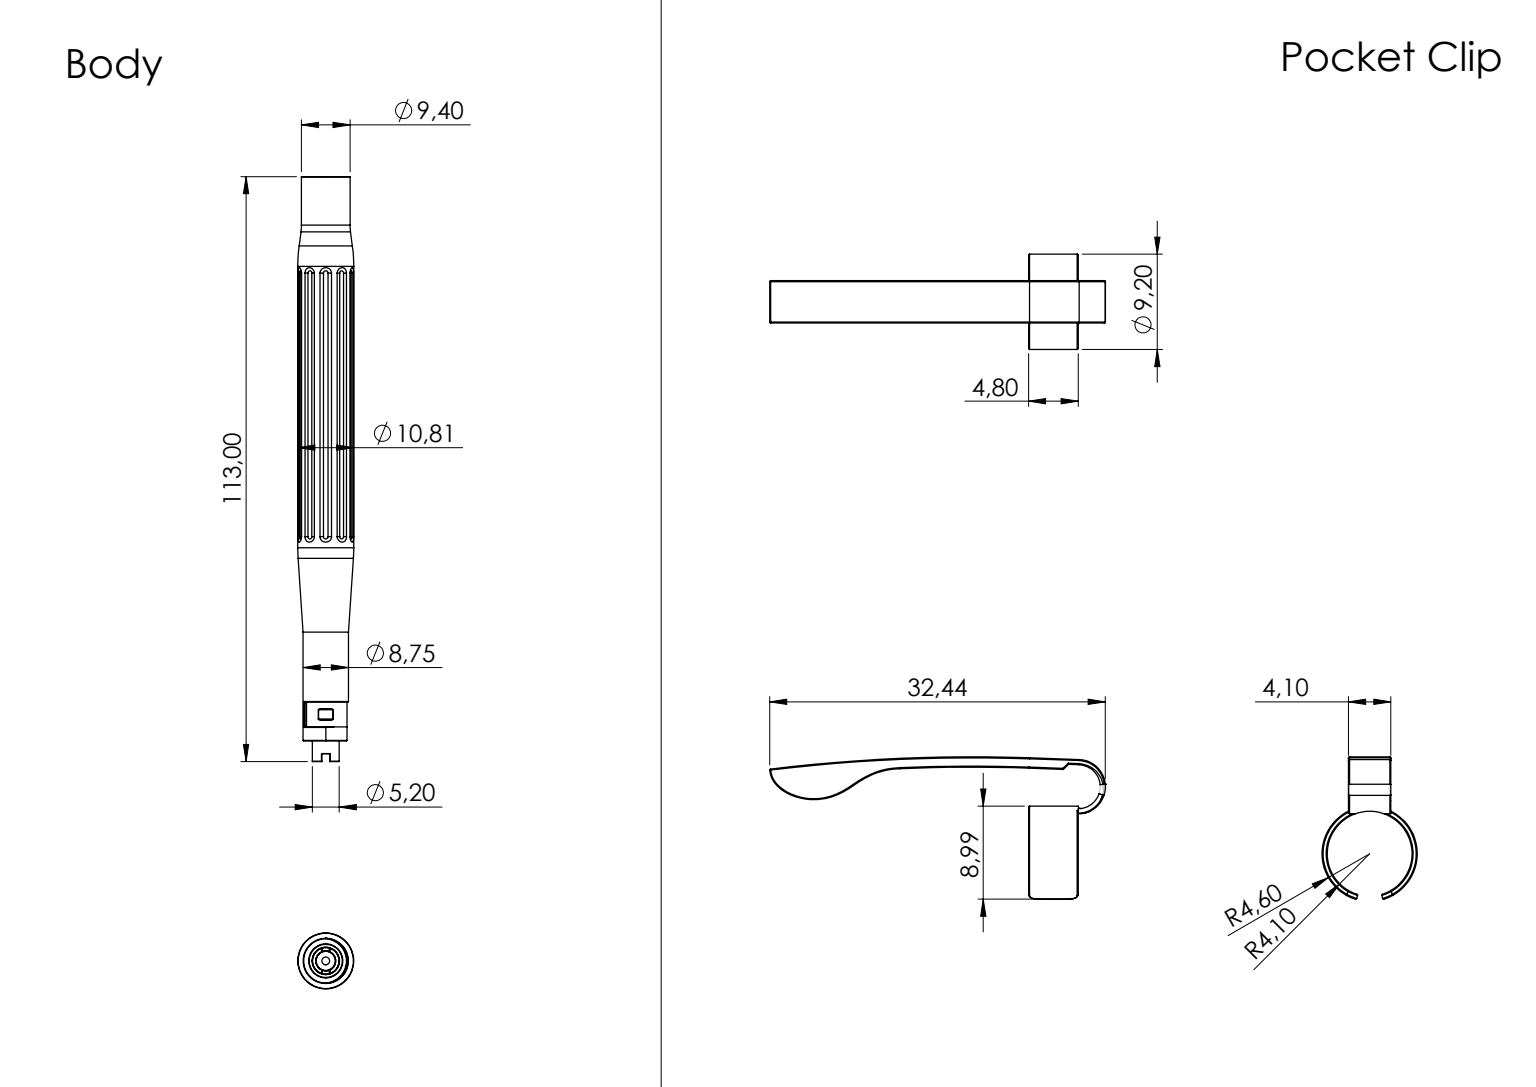
ISO-10303-21;
HEADER;
FILE_DESCRIPTION (('STEP AP214'),
    '1' );
FILE_NAME ('Body.step',
    '2026-10-06T14:00:01',
    ( '' ),
    ( '' ),
    'SwSTEP 2.0',
    'SolidWorks 2020',
    '' );
FILE_SCHEMA (( 'AUTOMOTIVE_DESIGN' ));
ENDSEC;

DATA;
#2=CARTESIAN_POINT ( 'NONE',  ( 51.90000000000001279, -4.227689052994015206, -1.125730994152046804 ) ) ;
#3=CARTESIAN_POINT ( 'NONE',  ( 15.76675455518197388, -3.095036031508637375, 4.435288302043580266 ) ) ;
#4=CARTESIAN_POINT ( 'NONE',  ( 48.30000000000001847, 0.7900853852131533017, -4.025789903357282817 ) ) ;
#5=ADVANCED_FACE ( 'NONE', ( #27029 ), #12933, .F. ) ;
#6=FACE_OUTER_BOUND ( 'NONE', #21820, .T. ) ;
#9=AXIS2_PLACEMENT_3D ( 'NONE', #6479, #25787, #7416 ) ;
#13=EDGE_CURVE ( 'NONE', #19424, #10038, #3404, .T. ) ;
#17=DIRECTION ( 'NONE',  ( 1.000000000000000000, 2.586136946169074517E-16, -0.000000000000000000 ) ) ;
#21=DIRECTION ( 'NONE',  ( 0.000000000000000000, -1.000000000000000000, 0.000000000000000000 ) ) ;
#22=CARTESIAN_POINT ( 'NONE',  ( -35.98994760229849987, 4.804073784580248585, 2.042134692980175803 ) ) ;
#23=LINE ( 'NONE', #15037, #26178 ) ;
#28=ORIENTED_EDGE ( 'NONE', *, *, #15447, .F. ) ;
#29=CARTESIAN_POINT ( 'NONE',  ( 56.95000000000001705, 0.000000000000000000, 0.000000000000000000 ) ) ;
#30=CARTESIAN_POINT ( 'NONE',  ( -35.85663232820584057, -3.426725943139554698, -3.937891353488750301 ) ) ;
#35=ORIENTED_EDGE ( 'NONE', *, *, #5756, .F. ) ;
#39=CIRCLE ( 'NONE', #6115, 0.4576450603546999840 ) ;
#43=CARTESIAN_POINT ( 'NONE',  ( -54.49999999999997868, -1.550000000000000044, 3.332135201338624508 ) ) ;
#47=CARTESIAN_POINT ( 'NONE',  ( -35.85663232820581925, -0.4576450603547171925, -5.200000000000000178 ) ) ;
#49=FACE_OUTER_BOUND ( 'NONE', #3992, .T. ) ;
#50=CARTESIAN_POINT ( 'NONE',  ( 54.42253022455169997, -6.265509898922181047E-05, -4.373069084971676013 ) ) ;
#51=DIRECTION ( 'NONE',  ( 0.000000000000000000, 1.224646799147353454E-16, 1.000000000000000000 ) ) ;
#54=CARTESIAN_POINT ( 'NONE',  ( -36.00197790576391554, -4.683225679163350641, -2.703237727951247393 ) ) ;
#56=CARTESIAN_POINT ( 'NONE',  ( 48.48092587705050960, -1.391939743175890420, 3.849999999996903899 ) ) ;
#61=AXIS2_PLACEMENT_3D ( 'NONE', #970, #25337, #5708 ) ;
#63=ORIENTED_EDGE ( 'NONE', *, *, #635, .F. ) ;
#68=DIRECTION ( 'NONE',  ( 0.000000000000000000, -1.000000000000000000, 0.000000000000000000 ) ) ;
#70=CARTESIAN_POINT ( 'NONE',  ( 48.45334018241207730, -1.329038565861417220, 3.861394075523871816 ) ) ;
#78=CARTESIAN_POINT ( 'NONE',  ( 56.95000000000001705, 0.6999999999999999556, -2.452039967047845437 ) ) ;
#79=CARTESIAN_POINT ( 'NONE',  ( -54.49999516060625382, -1.549196738101655590, 4.063926895246979143 ) ) ;
#82=CARTESIAN_POINT ( 'NONE',  ( 57.03951379057714632, 0.7794871794871794934, 1.732743413496389939 ) ) ;
#83=EDGE_CURVE ( 'NONE', #616, #4702, #25049, .T. ) ;
#88=CARTESIAN_POINT ( 'NONE',  ( 51.80000000000001847, -3.726179070414208372, 1.041421356237310025 ) ) ;
#94=ADVANCED_FACE ( 'NONE', ( #17865 ), #19516, .T. ) ;
#97=CYLINDRICAL_SURFACE ( 'NONE', #25500, 1.000000000000000000 ) ;
#99=CARTESIAN_POINT ( 'NONE',  ( 16.08093158123428523, 5.047763082740414298, 1.943828653492576608 ) ) ;
#101=ORIENTED_EDGE ( 'NONE', *, *, #4763, .T. ) ;
#102=ORIENTED_EDGE ( 'NONE', *, *, #5168, .T. ) ;
#103=DIRECTION ( 'NONE',  ( 0.000000000000000000, 0.000000000000000000, -1.000000000000000000 ) ) ;
#108=CARTESIAN_POINT ( 'NONE',  ( -36.40878371307408656, 5.360483378448119396, 0.7132926830813313135 ) ) ;
#110=FACE_OUTER_BOUND ( 'NONE', #15279, .T. ) ;
#112=DIRECTION ( 'NONE',  ( 0.000000000000000000, 0.000000000000000000, -1.000000000000000000 ) ) ;
#113=DIRECTION ( 'NONE',  ( -1.000000000000000000, -2.586136946169074517E-16, 0.000000000000000000 ) ) ;
#115=CIRCLE ( 'NONE', #28430, 0.1000000000000002554 ) ;
#117=ADVANCED_FACE ( 'NONE', ( #25134 ), #3461, .F. ) ;
#120=CARTESIAN_POINT ( 'NONE',  ( 50.41422517315185559, 1.132063507975340277, -3.941224428058361262 ) ) ;
#121=ADVANCED_FACE ( 'NONE', ( #2812 ), #19777, .T. ) ;
#127=CARTESIAN_POINT ( 'NONE',  ( -36.21152527658242803, -3.291455042465435632, -4.036171416105485577 ) ) ;
#131=EDGE_CURVE ( 'NONE', #11967, #18572, #4827, .T. ) ;
#132=CARTESIAN_POINT ( 'NONE',  ( -54.45981523601835761, 1.500740478982482973, 4.030402907299741599 ) ) ;
#134=FACE_OUTER_BOUND ( 'NONE', #215, .T. ) ;
#135=CARTESIAN_POINT ( 'NONE',  ( 48.39253357792949117, 1.341874354110782486, 3.874311046529112623 ) ) ;
#138=ORIENTED_EDGE ( 'NONE', *, *, #14220, .T. ) ;
#140=CARTESIAN_POINT ( 'NONE',  ( 15.03925126672133139, -3.817150320980667200, 2.203324261490537062 ) ) ;
#141=CARTESIAN_POINT ( 'NONE',  ( 33.47623932017462778, 1.123735532908285650, -5.289358697221546279 ) ) ;
#146=DIRECTION ( 'NONE',  ( 0.000000000000000000, 0.000000000000000000, -1.000000000000000000 ) ) ;
#147=EDGE_CURVE ( 'NONE', #30927, #10142, #27583, .T. ) ;
#148=CARTESIAN_POINT ( 'NONE',  ( -41.12388279035661753, -1.755788972190012401E-14, 0.000000000000000000 ) ) ;
#167=AXIS2_PLACEMENT_3D ( 'NONE', #14057, #2660, #14363 ) ;
#170=FACE_OUTER_BOUND ( 'NONE', #26252, .T. ) ;
#176=CARTESIAN_POINT ( 'NONE',  ( 47.00000000000002132, 2.428612866367529932E-14, -4.100000000000022737 ) ) ;
#178=ADVANCED_FACE ( 'NONE', ( #15936 ), #13241, .T. ) ;
#179=CARTESIAN_POINT ( 'NONE',  ( -35.98952425903315344, -5.086913993735696415, -1.171642046065874743 ) ) ;
#180=ORIENTED_EDGE ( 'NONE', *, *, #3282, .F. ) ;
#183=ORIENTED_EDGE ( 'NONE', *, *, #7527, .F. ) ;
#188=ADVANCED_FACE ( 'NONE', ( #10875 ), #20563, .T. ) ;
#191=CARTESIAN_POINT ( 'NONE',  ( 46.99980596162997415, -4.243812330823901746, 1.064491855880303151 ) ) ;
#192=CARTESIAN_POINT ( 'NONE',  ( 48.40116939571129961, 0.8930800907916158771, -3.925677024646232027 ) ) ;
#194=CARTESIAN_POINT ( 'NONE',  ( 34.55000000000001847, 3.184081677783118191E-16, -2.600000000000000089 ) ) ;
#209=CARTESIAN_POINT ( 'NONE',  ( 15.41170998834797778, 5.326676561279727551, 0.9978806102897876951 ) ) ;
#213=CARTESIAN_POINT ( 'NONE',  ( 48.48434962373865886, -1.386108502191528924, 3.851082811767820413 ) ) ;
#215=EDGE_LOOP ( 'NONE', ( #11588, #9037, #5325, #4414 ) ) ;
#216=CARTESIAN_POINT ( 'NONE',  ( 54.49969840703174384, -0.002993017367635220170, 4.282759600741086636 ) ) ;
#225=CYLINDRICAL_SURFACE ( 'NONE', #7886, 1.000000000000000000 ) ;
#226=PLANE ( 'NONE',  #873 ) ;
#227=CIRCLE ( 'NONE', #16912, 5.147405183146873675 ) ;
#230=VECTOR ( 'NONE', #19201, 1000.000000000000000 ) ;
#234=ORIENTED_EDGE ( 'NONE', *, *, #24307, .F. ) ;
#237=( BOUNDED_SURFACE ( )  B_SPLINE_SURFACE ( 3, 2, ( 
 ( #18207, #22472, #769 ),
 ( #20118, #8066, #17731 ),
 ( #5683, #3307, #12957 ),
 ( #11840, #21216, #1694 ),
 ( #4235, #13877, #16129 ),
 ( #28318, #30847, #18668 ),
 ( #14053, #11689, #9166 ),
 ( #18827, #11541, #18508 ),
 ( #23571, #16434, #23884 ),
 ( #28471, #4086, #21370 ),
 ( #6773, #6625, #1872 ),
 ( #26091, #21047, #30996 ),
 ( #16288, #9487, #23735 ),
 ( #25616, #2026, #30687 ),
 ( #28630, #2175, #8818 ),
 ( #21517, #4405, #13726 ) ),
 .UNSPECIFIED., .F., .F., .F. ) 
 B_SPLINE_SURFACE_WITH_KNOTS ( ( 4, 2, 2, 2, 2, 2, 2, 4 ),
 ( 3, 3 ),
 ( 0.001780502285214259107, 0.002558945925323788048, 0.002753556835351170500, 0.002948167745378552952, 0.003337389565433317423, 0.003726611385488081893, 0.004115833205542846797, 0.004894276845652375738 ),
 ( 0.000000000000000000, 1.000000000000000000 ),
 .UNSPECIFIED. ) 
 GEOMETRIC_REPRESENTATION_ITEM ( )  RATIONAL_B_SPLINE_SURFACE ( (
 ( 1.000000000000000000, 0.9418517008537233837, 1.000000000000000000),
 ( 1.000000000000000000, 0.9417987965885065149, 1.000000000000000000),
 ( 1.000000000000000000, 0.9418198861734086158, 1.000000000000000000),
 ( 1.000000000000000000, 0.9434060303845573925, 1.000000000000000000),
 ( 1.000000000000000000, 0.9437939819948161224, 1.000000000000000000),
 ( 1.000000000000000000, 0.9445989566712799101, 1.000000000000000000),
 ( 1.000000000000000000, 0.9450169930049959754, 1.000000000000000000),
 ( 1.000000000000000000, 0.9461610507673308135, 1.000000000000000000),
 ( 1.000000000000000000, 0.9467217966427053932, 1.000000000000000000),
 ( 1.000000000000000000, 0.9467345476124492398, 1.000000000000000000),
 ( 1.000000000000000000, 0.9461964028052997078, 1.000000000000000000),
 ( 1.000000000000000000, 0.9446801822473757104, 1.000000000000000000),
 ( 1.000000000000000000, 0.9437582546536171790, 1.000000000000000000),
 ( 1.000000000000000000, 0.9418129560296412128, 1.000000000000000000),
 ( 1.000000000000000000, 0.9418016889776917866, 1.000000000000000000),
 ( 1.000000000000000000, 0.9418517008537223845, 1.000000000000000000) ) ) 
 REPRESENTATION_ITEM ( '' )  SURFACE ( )  );
#240=CARTESIAN_POINT ( 'NONE',  ( 16.10667815269232150, 5.098435263432238962, 1.807398698456221142 ) ) ;
#242=ORIENTED_EDGE ( 'NONE', *, *, #16474, .T. ) ;
#246=CARTESIAN_POINT ( 'NONE',  ( -44.49999999999997868, -1.499999999999998668, 4.029888335921975262 ) ) ;
#247=VERTEX_POINT ( 'NONE', #25065 ) ;
#248=EDGE_CURVE ( 'NONE', #1696, #20370, #611, .T. ) ;
#250=ORIENTED_EDGE ( 'NONE', *, *, #30955, .F. ) ;
#252=ADVANCED_FACE ( 'NONE', ( #17489 ), #5461, .T. ) ;
#256=DIRECTION ( 'NONE',  ( -1.000000000000000000, -0.000000000000000000, -0.000000000000000000 ) ) ;
#257=CARTESIAN_POINT ( 'NONE',  ( 16.07512358269907438, -5.233646053067085191, -1.367284724151294872 ) ) ;
#261=EDGE_CURVE ( 'NONE', #13894, #14026, #10669, .T. ) ;
#263=CARTESIAN_POINT ( 'NONE',  ( -36.39645873810205501, -3.590618801409528160, -4.051716037497291367 ) ) ;
#266=CIRCLE ( 'NONE', #22541, 1.000000000000000000 ) ;
#269=CARTESIAN_POINT ( 'NONE',  ( 56.99370871690835116, -0.8156862421929632623, -2.468735699563065378 ) ) ;
#274=CARTESIAN_POINT ( 'NONE',  ( 36.55000000000001847, 0.000000000000000000, -1.899999999999999911 ) ) ;
#278=CARTESIAN_POINT ( 'NONE',  ( 15.22780280894145832, 0.7747498539022198427, -5.363501450340349308 ) ) ;
#279=CARTESIAN_POINT ( 'NONE',  ( -36.56390771145526486, -5.205077242910963520, 1.471673150993815238 ) ) ;
#280=CARTESIAN_POINT ( 'NONE',  ( 48.50000000000002132, -1.426739617975173013, -3.843750000000023093 ) ) ;
#282=ORIENTED_EDGE ( 'NONE', *, *, #8503, .F. ) ;
#290=CARTESIAN_POINT ( 'NONE',  ( 57.04536243881683788, -0.7794871794871796045, 1.732743413496389939 ) ) ;
#291=AXIS2_PLACEMENT_3D ( 'NONE', #19148, #17077, #12003 ) ;
#292=DIRECTION ( 'NONE',  ( -1.000000000000000000, -0.000000000000000000, -0.000000000000000000 ) ) ;
#301=CARTESIAN_POINT ( 'NONE',  ( 51.90000000000001279, 1.734723475976807094E-15, 0.000000000000000000 ) ) ;
#304=EDGE_CURVE ( 'NONE', #17048, #21964, #18751, .T. ) ;
#315=CARTESIAN_POINT ( 'NONE',  ( 57.01990854087920013, 0.7399312420039723115, -2.427820937803477630 ) ) ;
#324=EDGE_CURVE ( 'NONE', #29888, #4483, #21821, .T. ) ;
#325=DIRECTION ( 'NONE',  ( -1.000000000000000000, -2.586136946169074517E-16, 0.000000000000000000 ) ) ;
#328=CARTESIAN_POINT ( 'NONE',  ( 51.70000000000001705, -4.179189514726507682, 0.9999999999999997780 ) ) ;
#332=CARTESIAN_POINT ( 'NONE',  ( -36.92443669619682112, -5.094475812726876995, -1.819860688632578771 ) ) ;
#341=CARTESIAN_POINT ( 'NONE',  ( 50.40811050917463376, 1.340787288841451819, 3.874691554877328414 ) ) ;
#343=CARTESIAN_POINT ( 'NONE',  ( -54.47754877553799702, -1.508273929415538506, 3.305418158118663463 ) ) ;
#349=CARTESIAN_POINT ( 'NONE',  ( -36.43290890416756866, 0.4851603899458080682, -5.391500295856532787 ) ) ;
#350=EDGE_CURVE ( 'NONE', #30188, #2736, #13683, .T. ) ;
#353=CARTESIAN_POINT ( 'NONE',  ( 15.49702763512084047, 4.928592478219022688, -1.658905555082578864 ) ) ;
#354=CARTESIAN_POINT ( 'NONE',  ( 56.95000000000001705, -0.7137254901960784492, 2.500119182087999548 ) ) ;
#364=CARTESIAN_POINT ( 'NONE',  ( 33.47623932017462778, 1.734723475976807489E-15, 0.000000000000000000 ) ) ;
#368=EDGE_LOOP ( 'NONE', ( #14579, #11671, #14342, #26811 ) ) ;
#371=CARTESIAN_POINT ( 'NONE',  ( 15.56401610563845317, 5.370189181194952255, 0.6649548426264916268 ) ) ;
#373=CARTESIAN_POINT ( 'NONE',  ( 48.40000000000001990, -0.6304760106459033064, 3.950000000000022826 ) ) ;
#374=CIRCLE ( 'NONE', #8458, 0.05000000000000012768 ) ;
#376=ORIENTED_EDGE ( 'NONE', *, *, #28015, .T. ) ;
#380=CARTESIAN_POINT ( 'NONE',  ( -35.85663232820584057, 1.793057972834822156, -4.026191436120376999 ) ) ;
#384=CARTESIAN_POINT ( 'NONE',  ( -54.48779575765000516, -1.517266520141195896, 4.041867453639656382 ) ) ;
#386=AXIS2_PLACEMENT_3D ( 'NONE', #15477, #25133, #23717 ) ;
#393=ADVANCED_FACE ( 'NONE', ( #19503 ), #26715, .T. ) ;
#415=ORIENTED_EDGE ( 'NONE', *, *, #7693, .T. ) ;
#420=CARTESIAN_POINT ( 'NONE',  ( 15.41217651307630376, -4.863043649742736285, -1.860644097022675414 ) ) ;
#424=CARTESIAN_POINT ( 'NONE',  ( 50.36059168657180862, 1.279117291415143853, -3.870058441400159754 ) ) ;
#426=CARTESIAN_POINT ( 'NONE',  ( 15.18463186935387377, -4.683225679163126820, -2.703237727951754543 ) ) ;
#432=CARTESIAN_POINT ( 'NONE',  ( -36.68133364217528225, -3.736273719777210456, -3.909490113446789206 ) ) ;
#438=CARTESIAN_POINT ( 'NONE',  ( -36.11692583559979397, -4.683225668089311178, 2.703237747136467473 ) ) ;
#440=CARTESIAN_POINT ( 'NONE',  ( 56.95000000000001705, 0.000000000000000000, 0.000000000000000000 ) ) ;
#441=EDGE_LOOP ( 'NONE', ( #30062, #24496, #16415, #15926 ) ) ;
#444=CARTESIAN_POINT ( 'NONE',  ( 50.50000000000002132, 0.6304760106459513791, 3.950000000000021938 ) ) ;
#446=CARTESIAN_POINT ( 'NONE',  ( -54.44999999999997442, 0.000000000000000000, 4.349999999999997868 ) ) ;
#458=CIRCLE ( 'NONE', #5023, 0.05000000000000012768 ) ;
#467=DIRECTION ( 'NONE',  ( 1.000000000000000000, 3.385297212316258532E-16, -2.459562394685744279E-16 ) ) ;
#469=DIRECTION ( 'NONE',  ( 0.000000000000000000, 0.000000000000000000, 1.000000000000000000 ) ) ;
#473=VERTEX_POINT ( 'NONE', #3169 ) ;
#475=DIRECTION ( 'NONE',  ( -1.000000000000000000, -0.000000000000000000, -0.000000000000000000 ) ) ;
#476=EDGE_CURVE ( 'NONE', #20395, #3490, #29876, .T. ) ;
#478=ORIENTED_EDGE ( 'NONE', *, *, #27718, .F. ) ;
#480=CARTESIAN_POINT ( 'NONE',  ( 50.39883060428874728, 0.8930800907916158771, 3.925677024646232027 ) ) ;
#481=CARTESIAN_POINT ( 'NONE',  ( -36.68133364217572989, -5.320649567603509489, -0.9667173501063568430 ) ) ;
#487=EDGE_CURVE ( 'NONE', #25704, #26503, #27864, .T. ) ;
#494=CARTESIAN_POINT ( 'NONE',  ( 48.37881665787880081, -1.311095223031167656, -3.884869838566831657 ) ) ;
#496=CARTESIAN_POINT ( 'NONE',  ( 51.80019403837007275, -4.243812330823898193, -1.064491855880295157 ) ) ;
#502=EDGE_CURVE ( 'NONE', #31046, #17227, #27711, .T. ) ;
#505=CARTESIAN_POINT ( 'NONE',  ( 15.17256654081408307, 4.804073784580281448, -2.042134692980007937 ) ) ;
#508=LINE ( 'NONE', #19531, #10386 ) ;
#510=CARTESIAN_POINT ( 'NONE',  ( 15.29449157529453984, 2.734387802834222558, -4.440904455451668120 ) ) ;
#513=ORIENTED_EDGE ( 'NONE', *, *, #6499, .F. ) ;
#518=VERTEX_POINT ( 'NONE', #3495 ) ;
#519=ORIENTED_EDGE ( 'NONE', *, *, #15693, .T. ) ;
#520=CARTESIAN_POINT ( 'NONE',  ( 15.03925126672132784, 5.377732432866634937, 0.5657657256216264141 ) ) ;
#524=DIRECTION ( 'NONE',  ( -4.117859380279907901E-15, -0.9495137264943731559, -0.3137254901960768172 ) ) ;
#529=EDGE_CURVE ( 'NONE', #10936, #30188, #15204, .T. ) ;
#533=EDGE_CURVE ( 'NONE', #27746, #12623, #23876, .T. ) ;
#534=CARTESIAN_POINT ( 'NONE',  ( -54.49608498031047787, -1.530604779201329091, 4.051096982736678953 ) ) ;
#539=DIRECTION ( 'NONE',  ( 1.000000000000000000, 0.000000000000000000, 0.000000000000000000 ) ) ;
#540=EDGE_CURVE ( 'NONE', #20985, #4962, #20292, .T. ) ;
#548=ORIENTED_EDGE ( 'NONE', *, *, #30878, .F. ) ;
#558=EDGE_LOOP ( 'NONE', ( #6600, #18904, #20461, #4910 ) ) ;
#560=VERTEX_POINT ( 'NONE', #22668 ) ;
#562=ORIENTED_EDGE ( 'NONE', *, *, #8648, .F. ) ;
#567=CARTESIAN_POINT ( 'NONE',  ( 15.22780280894113325, -4.861582133260076155, -2.394243994562784916 ) ) ;
#568=EDGE_CURVE ( 'NONE', #19552, #25905, #3138, .T. ) ;
#573=CARTESIAN_POINT ( 'NONE',  ( -44.49999999999997868, -1.500000000000000000, 3.300094695611020867 ) ) ;
#581=CARTESIAN_POINT ( 'NONE',  ( -36.30347965937272647, -3.148602930107041065, -4.139959549308994902 ) ) ;
#598=CARTESIAN_POINT ( 'NONE',  ( 56.95000000000001705, -0.6820512820512819596, 1.773360101234998210 ) ) ;
#600=CARTESIAN_POINT ( 'NONE',  ( 58.50000000000001421, 0.000000000000000000, 0.000000000000000000 ) ) ;
#601=AXIS2_PLACEMENT_3D ( 'NONE', #25474, #29769, #15523 ) ;
#603=CIRCLE ( 'NONE', #61, 4.700000000000000178 ) ;
#605=CARTESIAN_POINT ( 'NONE',  ( 48.40000000000001990, 2.428612866367529932E-14, 0.000000000000000000 ) ) ;
#607=ORIENTED_EDGE ( 'NONE', *, *, #22678, .F. ) ;
#608=CARTESIAN_POINT ( 'NONE',  ( 16.07279755198631932, 2.910597594660116805, 4.559461819278099348 ) ) ;
#611=B_SPLINE_CURVE_WITH_KNOTS ( 'NONE', 3,
 ( #22873, #22726, #25234, #10817, #1022, #20026, #10673, #13190, #29668, #29978, #1162, #27768, #14940, #12569, #5615, #22258, #19870, #29499, #7815 ),
 .UNSPECIFIED., .F., .F.,
 ( 4, 3, 3, 3, 3, 3, 4 ),
 ( 0.000000000000000000, 1.485152479261659526E-05, 2.963899638137937738E-05, 4.531421101975830796E-05, 6.339282692920775891E-05, 8.412900350910317146E-05, 8.561427748423838346E-05 ),
 .UNSPECIFIED. ) ;
#612=LINE ( 'NONE', #20579, #31143 ) ;
#613=CARTESIAN_POINT ( 'NONE',  ( -36.38012252111234091, 4.735538777079434603, -2.618062770414225859 ) ) ;
#616=VERTEX_POINT ( 'NONE', #13744 ) ;
#618=VERTEX_POINT ( 'NONE', #31015 ) ;
#622=DIRECTION ( 'NONE',  ( 0.000000000000000000, 0.2745098039215694841, -0.9615843008030765526 ) ) ;
#623=DIRECTION ( 'NONE',  ( -1.000000000000000000, -2.586136946169074517E-16, 0.000000000000000000 ) ) ;
#633=CARTESIAN_POINT ( 'NONE',  ( -36.56390771145526486, -5.076023720898236391, -1.868859051106839475 ) ) ;
#635=EDGE_CURVE ( 'NONE', #25117, #29888, #25505, .T. ) ;
#641=DIRECTION ( 'NONE',  ( 0.000000000000000000, 1.000000000000000000, 0.000000000000000000 ) ) ;
#643=CARTESIAN_POINT ( 'NONE',  ( 15.45522337368519850, -0.1928884786867813006, 5.200000000471195705 ) ) ;
#649=CIRCLE ( 'NONE', #30477, 4.300000000000019362 ) ;
#650=DIRECTION ( 'NONE',  ( 0.000000000000000000, -0.000000000000000000, -1.000000000000000000 ) ) ;
#651=CARTESIAN_POINT ( 'NONE',  ( 15.97944027357901753, -3.614202567155989421, 4.024415706308047014 ) ) ;
#652=CARTESIAN_POINT ( 'NONE',  ( 15.76675455518219238, 5.110933801299809787, -1.769007076671054390 ) ) ;
#655=CARTESIAN_POINT ( 'NONE',  ( 50.42106458229518751, -0.9199776782966014865, -3.998258245321812510 ) ) ;
#656=CARTESIAN_POINT ( 'NONE',  ( -35.85663232820583346, -4.683225679163351529, -2.703237727951242952 ) ) ;
#657=CARTESIAN_POINT ( 'NONE',  ( 15.44631504820162426, 2.881190829692330979, -4.334245811858005837 ) ) ;
#674=ORIENTED_EDGE ( 'NONE', *, *, #25991, .F. ) ;
#678=CIRCLE ( 'NONE', #10773, 1.850000000000000089 ) ;
#681=PLANE ( 'NONE',  #3139 ) ;
#684=FACE_OUTER_BOUND ( 'NONE', #441, .T. ) ;
#686=EDGE_CURVE ( 'NONE', #24297, #29070, #5670, .T. ) ;
#687=CARTESIAN_POINT ( 'NONE',  ( -36.48821680285185209, -3.495540671458102988, 4.131527132740904662 ) ) ;
#688=CARTESIAN_POINT ( 'NONE',  ( 15.03925126672133139, -4.945493884734801782, 1.606888370749709027 ) ) ;
#689=CARTESIAN_POINT ( 'NONE',  ( 50.40000000000001990, 2.428612866367529932E-14, 0.000000000000000000 ) ) ;
#693=AXIS2_PLACEMENT_3D ( 'NONE', #28518, #6823, #16487 ) ;
#694=EDGE_LOOP ( 'NONE', ( #11145, #17669, #9882, #6922 ) ) ;
#697=ORIENTED_EDGE ( 'NONE', *, *, #22187, .T. ) ;
#699=CARTESIAN_POINT ( 'NONE',  ( -54.44999999999997442, 1.499999999999999556, -4.029888335921975262 ) ) ;
#701=CARTESIAN_POINT ( 'NONE',  ( 15.59140265158955074, 4.755985070912251977, 2.573747172434746933 ) ) ;
#708=EDGE_CURVE ( 'NONE', #25469, #23625, #14965, .T. ) ;
#711=EDGE_CURVE ( 'NONE', #13242, #19150, #227, .T. ) ;
#715=CARTESIAN_POINT ( 'NONE',  ( 15.44259799936802047, -4.878092280899799071, -1.814329181850236727 ) ) ;
#722=DIRECTION ( 'NONE',  ( -1.000000000000000000, -0.000000000000000000, -0.000000000000000000 ) ) ;
#726=LINE ( 'NONE', #12044, #17578 ) ;
#727=( BOUNDED_SURFACE ( )  B_SPLINE_SURFACE ( 3, 2, ( 
 ( #12834, #20466, #5581 ),
 ( #10487, #25026, #12537 ),
 ( #20162, #17300, #5726 ),
 ( #27562, #24567, #15231 ),
 ( #22842, #24876, #22516 ),
 ( #10317, #17450, #27263 ),
 ( #26944, #29627, #819 ),
 ( #5891, #1131, #29792 ),
 ( #7953, #13008, #10783 ),
 ( #3357, #17618, #24731 ),
 ( #2886, #5252, #13156 ),
 ( #3192, #8255, #657 ),
 ( #8106, #3044, #22692 ),
 ( #5419, #22223, #510 ),
 ( #12687, #17775, #987 ),
 ( #10167, #27416, #17922 ) ),
 .UNSPECIFIED., .F., .F., .F. ) 
 B_SPLINE_SURFACE_WITH_KNOTS ( ( 4, 2, 2, 2, 2, 2, 2, 4 ),
 ( 3, 3 ),
 ( 0.001780502285214198826, 0.002558945925323778507, 0.002753556835351173536, 0.002948167745378568131, 0.003337389565433357755, 0.003726611385488147379, 0.004115833205542937002, 0.004894276845652516250 ),
 ( 0.000000000000000000, 1.000000000000000000 ),
 .UNSPECIFIED. ) 
 GEOMETRIC_REPRESENTATION_ITEM ( )  RATIONAL_B_SPLINE_SURFACE ( (
 ( 1.000000000000000000, 0.9418517008537241608, 1.000000000000000000),
 ( 1.000000000000000000, 0.9417987965884988544, 1.000000000000000000),
 ( 1.000000000000000000, 0.9418198861734230487, 1.000000000000000000),
 ( 1.000000000000000000, 0.9434060303845539508, 1.000000000000000000),
 ( 1.000000000000000000, 0.9437939819948095721, 1.000000000000000000),
 ( 1.000000000000000000, 0.9445989566712880148, 1.000000000000000000),
 ( 1.000000000000000000, 0.9450169930049983069, 1.000000000000000000),
 ( 1.000000000000000000, 0.9461610507673332560, 1.000000000000000000),
 ( 1.000000000000000000, 0.9467217966427213804, 1.000000000000000000),
 ( 1.000000000000000000, 0.9467345476124363612, 1.000000000000000000),
 ( 1.000000000000000000, 0.9461964028052722853, 1.000000000000000000),
 ( 1.000000000000000000, 0.9446801822474062416, 1.000000000000000000),
 ( 1.000000000000000000, 0.9437582546536901207, 1.000000000000000000),
 ( 1.000000000000000000, 0.9418129560294949965, 1.000000000000000000),
 ( 1.000000000000000000, 0.9418016889778024758, 1.000000000000000000),
 ( 1.000000000000000000, 0.9418517008537236057, 1.000000000000000000) ) ) 
 REPRESENTATION_ITEM ( '' )  SURFACE ( )  );
#731=ADVANCED_FACE ( 'NONE', ( #7124 ), #21860, .F. ) ;
#733=CARTESIAN_POINT ( 'NONE',  ( -36.26369610968621515, -2.881190829692320321, -4.334245811858070674 ) ) ;
#736=DIRECTION ( 'NONE',  ( 0.000000000000000000, -0.9119702176296791141, -0.4102564102564098536 ) ) ;
#739=CARTESIAN_POINT ( 'NONE',  ( 15.30042582489635095, -1.123735543663344938, -5.289358694936611371 ) ) ;
#740=AXIS2_PLACEMENT_3D ( 'NONE', #8039, #24813, #27350 ) ;
#745=DIRECTION ( 'NONE',  ( 0.000000000000000000, 0.000000000000000000, -1.000000000000000000 ) ) ;
#746=DIRECTION ( 'NONE',  ( 0.000000000000000000, 0.000000000000000000, -1.000000000000000000 ) ) ;
#747=ORIENTED_EDGE ( 'NONE', *, *, #9238, .F. ) ;
#749=DIRECTION ( 'NONE',  ( -1.000000000000000000, -2.586136946169074517E-16, 0.000000000000000000 ) ) ;
#750=AXIS2_PLACEMENT_3D ( 'NONE', #11893, #21738, #11742 ) ;
#751=CARTESIAN_POINT ( 'NONE',  ( -44.49999999999997868, 0.000000000000000000, 0.000000000000000000 ) ) ;
#754=CARTESIAN_POINT ( 'NONE',  ( 56.97512559646294505, -0.7466375667864569854, 1.747149777169433094 ) ) ;
#759=CARTESIAN_POINT ( 'NONE',  ( 15.59055531549694074, 0.9785522574022036402, 5.318456145981286909 ) ) ;
#768=CARTESIAN_POINT ( 'NONE',  ( -35.85663232820582635, 4.861582140531628404, -2.394243978978282783 ) ) ;
#769=CARTESIAN_POINT ( 'NONE',  ( -35.85663232820581925, 0.4576450603546987073, 5.200000000000000178 ) ) ;
#770=CARTESIAN_POINT ( 'NONE',  ( 48.44629147628577215, 1.309359793766484925, -3.864871860988134955 ) ) ;
#774=ORIENTED_EDGE ( 'NONE', *, *, #19717, .T. ) ;
#777=CARTESIAN_POINT ( 'NONE',  ( 15.03925126672133139, -4.018128179617529661, -3.618665901676669350 ) ) ;
#778=DIRECTION ( 'NONE',  ( -1.000000000000000000, -0.000000000000000000, -0.000000000000000000 ) ) ;
#787=CARTESIAN_POINT ( 'NONE',  ( 51.79804399563283823, -4.143014423056512463, 1.077153443819862000 ) ) ;
#792=CIRCLE ( 'NONE', #10394, 0.05000000000000012768 ) ;
#809=CARTESIAN_POINT ( 'NONE',  ( 58.50000000000001421, -0.8156862745098042433, 2.468735688885369317 ) ) ;
#812=CARTESIAN_POINT ( 'NONE',  ( -35.85663232820584057, 3.426725943139577790, -3.937891353488711221 ) ) ;
#813=EDGE_CURVE ( 'NONE', #21791, #9481, #23476, .T. ) ;
#816=CARTESIAN_POINT ( 'NONE',  ( 58.45000000000001705, 0.8000000000000002665, 2.421260002560650104 ) ) ;
#818=CARTESIAN_POINT ( 'NONE',  ( 19.23646557533807666, -5.338914163118011480, 0.000000000000000000 ) ) ;
#819=CARTESIAN_POINT ( 'NONE',  ( 15.45522337368517007, 3.212533369474642075, -4.093511368021645502 ) ) ;
#820=CARTESIAN_POINT ( 'NONE',  ( 15.03925126672132961, -0.4576450603546909912, -5.200000000000000178 ) ) ;
#825=TOROIDAL_SURFACE ( 'NONE', #18539, 4.275000000000000355, 0.1000000000000000056 ) ;
#829=ORIENTED_EDGE ( 'NONE', *, *, #540, .T. ) ;
#830=AXIS2_PLACEMENT_3D ( 'NONE', #10089, #14821, #7562 ) ;
#831=CARTESIAN_POINT ( 'NONE',  ( 16.10660252424456118, 5.053896291911992300, -1.944420249220595087 ) ) ;
#832=FACE_OUTER_BOUND ( 'NONE', #30522, .T. ) ;
#838=CIRCLE ( 'NONE', #28645, 0.05000000000000002359 ) ;
#839=DIRECTION ( 'NONE',  ( 0.000000000000000000, 0.000000000000000000, 1.000000000000000000 ) ) ;
#850=CARTESIAN_POINT ( 'NONE',  ( 57.02888841125436414, -0.7778303923484506388, -1.733491207451775207 ) ) ;
#853=CARTESIAN_POINT ( 'NONE',  ( 50.50000000000002132, 2.478823385132571406E-14, 4.100000000000022737 ) ) ;
#855=TOROIDAL_SURFACE ( 'NONE', #7439, 14.70000000000000995, 10.00000000000000000 ) ;
#857=CARTESIAN_POINT ( 'NONE',  ( 50.30000000000001847, -1.426739617975173013, -3.843750000000023093 ) ) ;
#862=AXIS2_PLACEMENT_3D ( 'NONE', #23773, #6339, #16472 ) ;
#867=CARTESIAN_POINT ( 'NONE',  ( -54.49999999999997868, 1.549999999999999600, -4.064480286580312907 ) ) ;
#871=ORIENTED_EDGE ( 'NONE', *, *, #6348, .T. ) ;
#873=AXIS2_PLACEMENT_3D ( 'NONE', #4818, #30956, #16389 ) ;
#877=LINE ( 'NONE', #29989, #14989 ) ;
#879=ORIENTED_EDGE ( 'NONE', *, *, #28610, .F. ) ;
#881=ORIENTED_EDGE ( 'NONE', *, *, #9302, .T. ) ;
#883=ADVANCED_FACE ( 'NONE', ( #20259, #26238, #4545, #26073, #16117, #21027 ), #30830, .T. ) ;
#889=AXIS2_PLACEMENT_3D ( 'NONE', #16006, #20779, #20468 ) ;
#890=CARTESIAN_POINT ( 'NONE',  ( 15.03925126672133139, -5.086913985776139846, -1.171642053949128126 ) ) ;
#895=CIRCLE ( 'NONE', #25653, 0.7500000000000186517 ) ;
#898=FACE_OUTER_BOUND ( 'NONE', #17661, .T. ) ;
#903=CARTESIAN_POINT ( 'NONE',  ( -35.85663232820583346, -4.383220986679503994, -0.4611378927914501769 ) ) ;
#905=CARTESIAN_POINT ( 'NONE',  ( 58.45000000000001705, 0.8000000000000000444, -2.421260002560649660 ) ) ;
#907=ORIENTED_EDGE ( 'NONE', *, *, #18125, .T. ) ;
#910=CIRCLE ( 'NONE', #6467, 30.00000000000000000 ) ;
#918=FACE_OUTER_BOUND ( 'NONE', #25241, .T. ) ;
#926=DIRECTION ( 'NONE',  ( 0.000000000000000000, 0.000000000000000000, 1.000000000000000000 ) ) ;
#927=CARTESIAN_POINT ( 'NONE',  ( 34.55000000000001847, 0.000000000000000000, -2.649999999999999911 ) ) ;
#933=CARTESIAN_POINT ( 'NONE',  ( 51.70000000000001705, -4.179189514726506793, -1.000000000000000000 ) ) ;
#938=( BOUNDED_SURFACE ( )  B_SPLINE_SURFACE ( 3, 2, ( 
 ( #19024, #11734, #2554 ),
 ( #30892, #16809, #26139 ),
 ( #9821, #23778, #2069 ),
 ( #9208, #19488, #24077 ),
 ( #6815, #12054, #9683 ),
 ( #7455, #26771, #5074 ),
 ( #14726, #24387, #18869 ),
 ( #21408, #28682, #26299 ),
 ( #4600, #23927, #17739 ),
 ( #27380, #15509, #24528 ),
 ( #12649, #29433, #19952 ),
 ( #15193, #29585, #12336 ),
 ( #12966, #5373, #3313 ),
 ( #7745, #5690, #17411 ),
 ( #24842, #10282, #22184 ),
 ( #777, #24694, #20281 ) ),
 .UNSPECIFIED., .F., .F., .F. ) 
 B_SPLINE_SURFACE_WITH_KNOTS ( ( 4, 2, 2, 2, 2, 2, 2, 4 ),
 ( 3, 3 ),
 ( 0.001780502285214210318, 0.002558945925323797589, 0.002753556835351194353, 0.002948167745378591116, 0.003337389565433385077, 0.003726611385488179037, 0.004115833205542972564, 0.004894276845652559618 ),
 ( 0.000000000000000000, 1.000000000000000000 ),
 .UNSPECIFIED. ) 
 GEOMETRIC_REPRESENTATION_ITEM ( )  RATIONAL_B_SPLINE_SURFACE ( (
 ( 1.000000000000000000, 0.9418517008537219404, 1.000000000000000000),
 ( 1.000000000000000000, 0.9417987965885504797, 1.000000000000000000),
 ( 1.000000000000000000, 0.9418198861733489968, 1.000000000000000000),
 ( 1.000000000000000000, 0.9434060303845699380, 1.000000000000000000),
 ( 1.000000000000000000, 0.9437939819948041320, 1.000000000000000000),
 ( 1.000000000000000000, 0.9445989566712896801, 1.000000000000000000),
 ( 1.000000000000000000, 0.9450169930049926448, 1.000000000000000000),
 ( 1.000000000000000000, 0.9461610507673384740, 1.000000000000000000),
 ( 1.000000000000000000, 0.9467217966427268205, 1.000000000000000000),
 ( 1.000000000000000000, 0.9467345476124273684, 1.000000000000000000),
 ( 1.000000000000000000, 0.9461964028052701758, 1.000000000000000000),
 ( 1.000000000000000000, 0.9446801822474041321, 1.000000000000000000),
 ( 1.000000000000000000, 0.9437582546536517070, 1.000000000000000000),
 ( 1.000000000000000000, 0.9418129560295660507, 1.000000000000000000),
 ( 1.000000000000000000, 0.9418016889777457434, 1.000000000000000000),
 ( 1.000000000000000000, 0.9418517008537213853, 1.000000000000000000) ) ) 
 REPRESENTATION_ITEM ( '' )  SURFACE ( )  );
#941=CARTESIAN_POINT ( 'NONE',  ( 58.45000000000001705, -0.8000000000000000444, -2.421260002560650104 ) ) ;
#943=EDGE_CURVE ( 'NONE', #26590, #11900, #22875, .T. ) ;
#949=FACE_OUTER_BOUND ( 'NONE', #15304, .T. ) ;
#956=CARTESIAN_POINT ( 'NONE',  ( 58.50000000000001421, 0.8000000000000000444, -2.421260002560650104 ) ) ;
#958=VECTOR ( 'NONE', #6160, 1000.000000000000000 ) ;
#969=EDGE_CURVE ( 'NONE', #29917, #14986, #115, .T. ) ;
#970=CARTESIAN_POINT ( 'NONE',  ( -45.15971931043468146, 0.000000000000000000, 0.000000000000000000 ) ) ;
#974=CARTESIAN_POINT ( 'NONE',  ( 15.03925126672132961, 0.4576450603546987073, 5.200000000000000178 ) ) ;
#976=CARTESIAN_POINT ( 'NONE',  ( 57.05000000000001847, -0.7500000000000000000, -2.421260002560649660 ) ) ;
#983=ORIENTED_EDGE ( 'NONE', *, *, #25197, .F. ) ;
#984=CARTESIAN_POINT ( 'NONE',  ( 50.29999999999740368, -1.409901620923685206, -3.849999999997240518 ) ) ;
#987=CARTESIAN_POINT ( 'NONE',  ( 15.17256654081427492, 2.686240678227970413, -4.475885392925021300 ) ) ;
#992=CARTESIAN_POINT ( 'NONE',  ( 47.10000000000002274, -4.179189514726507682, 0.9999999999999997780 ) ) ;
#994=ORIENTED_EDGE ( 'NONE', *, *, #9268, .T. ) ;
#1000=ORIENTED_EDGE ( 'NONE', *, *, #568, .F. ) ;
#1001=DIRECTION ( 'NONE',  ( 1.000000000000000000, 8.626663965456006092E-17, 1.494526870159786164E-16 ) ) ;
#1007=ORIENTED_EDGE ( 'NONE', *, *, #19113, .F. ) ;
#1008=CIRCLE ( 'NONE', #25269, 0.05000000000000014155 ) ;
#1011=DIRECTION ( 'NONE',  ( -1.000000000000000000, 0.000000000000000000, 0.000000000000000000 ) ) ;
#1012=DIRECTION ( 'NONE',  ( 0.000000000000000000, 0.000000000000000000, 1.000000000000000000 ) ) ;
#1019=DIRECTION ( 'NONE',  ( 1.000000000000000000, 4.939082069373669245E-17, -1.520093157366878429E-16 ) ) ;
#1020=CIRCLE ( 'NONE', #14671, 4.100000000000022737 ) ;
#1022=CARTESIAN_POINT ( 'NONE',  ( -54.46926330052497178, 1.503605180550108944, -3.302415457191590242 ) ) ;
#1028=ORIENTED_EDGE ( 'NONE', *, *, #14158, .T. ) ;
#1029=ORIENTED_EDGE ( 'NONE', *, *, #3047, .F. ) ;
#1035=ORIENTED_EDGE ( 'NONE', *, *, #13354, .T. ) ;
#1044=CARTESIAN_POINT ( 'NONE',  ( 47.07331232995326786, -4.179189507151050087, -1.000000000000000000 ) ) ;
#1049=CARTESIAN_POINT ( 'NONE',  ( 48.47377487419020525, 1.373801017329653762, 3.853344662332955473 ) ) ;
#1065=AXIS2_PLACEMENT_3D ( 'NONE', #15106, #7993, #24766 ) ;
#1071=FACE_OUTER_BOUND ( 'NONE', #23504, .T. ) ;
#1073=DIRECTION ( 'NONE',  ( 0.000000000000000000, -1.000000000000000000, -1.532429380227459806E-15 ) ) ;
#1076=CARTESIAN_POINT ( 'NONE',  ( -36.77443515226919857, 5.298557911012499844, -1.088945631943488701 ) ) ;
#1080=EDGE_CURVE ( 'NONE', #7967, #2662, #20471, .T. ) ;
#1082=EDGE_CURVE ( 'NONE', #13576, #11503, #6680, .T. ) ;
#1085=CARTESIAN_POINT ( 'NONE',  ( 15.61033468494287213, 2.777216423307958593, 4.646230875016923889 ) ) ;
#1086=DIRECTION ( 'NONE',  ( 1.000000000000000000, 0.000000000000000000, 0.000000000000000000 ) ) ;
#1093=VERTEX_POINT ( 'NONE', #17980 ) ;
#1097=CARTESIAN_POINT ( 'NONE',  ( 48.41523095594689607, 1.115727354199254950, 3.895947837398489266 ) ) ;
#1098=CARTESIAN_POINT ( 'NONE',  ( 33.47623932017462778, -4.374999999999999112, 0.000000000000000000 ) ) ;
#1100=EDGE_LOOP ( 'NONE', ( #28602, #8868, #21545 ) ) ;
#1101=VERTEX_POINT ( 'NONE', #24789 ) ;
#1103=CIRCLE ( 'NONE', #12224, 0.05000000000000009298 ) ;
#1105=ORIENTED_EDGE ( 'NONE', *, *, #20548, .F. ) ;
#1110=EDGE_CURVE ( 'NONE', #3021, #6673, #8594, .T. ) ;
#1118=CARTESIAN_POINT ( 'NONE',  ( 48.40000000000002700, -0.6304760106459031954, -3.950000000000022826 ) ) ;
#1120=CARTESIAN_POINT ( 'NONE',  ( 15.87128154250933321, 0.7269167730138683670, 5.359285300587708356 ) ) ;
#1123=CARTESIAN_POINT ( 'NONE',  ( -36.04581030752770232, 0.7747498452705172678, -5.363501451416294863 ) ) ;
#1125=DIRECTION ( 'NONE',  ( 1.000000000000000000, 0.000000000000000000, 0.000000000000000000 ) ) ;
#1126=LINE ( 'NONE', #8249, #22099 ) ;
#1127=EDGE_LOOP ( 'NONE', ( #21119, #3709, #15108, #26941 ) ) ;
#1128=CARTESIAN_POINT ( 'NONE',  ( -35.85663232820584057, -1.123735532908306523, -5.289358697221545391 ) ) ;
#1129=CARTESIAN_POINT ( 'NONE',  ( -36.81959771849334828, 3.629052419422239328, -4.014440194077178781 ) ) ;
#1131=CARTESIAN_POINT ( 'NONE',  ( 15.74504787372188730, 3.350344226587782082, -4.246692235171858343 ) ) ;
#1134=EDGE_CURVE ( 'NONE', #8004, #2659, #17833, .T. ) ;
#1137=CARTESIAN_POINT ( 'NONE',  ( 47.05702803641548826, -4.175266387598157714, 1.009028806847064974 ) ) ;
#1139=EDGE_CURVE ( 'NONE', #17756, #7548, #15178, .T. ) ;
#1140=CARTESIAN_POINT ( 'NONE',  ( 47.04142135623732202, -3.767600426651517509, -1.000000000000000000 ) ) ;
#1141=VERTEX_POINT ( 'NONE', #8013 ) ;
#1142=DIRECTION ( 'NONE',  ( 1.000000000000000000, 2.586136946169074517E-16, -0.000000000000000000 ) ) ;
#1147=ORIENTED_EDGE ( 'NONE', *, *, #8319, .F. ) ;
#1148=CARTESIAN_POINT ( 'NONE',  ( 56.96065904101961763, 0.7273651001630837554, -1.755300599839360265 ) ) ;
#1155=CARTESIAN_POINT ( 'NONE',  ( 57.01898512823798626, -0.7746824256175574019, -1.734896867090173211 ) ) ;
#1162=CARTESIAN_POINT ( 'NONE',  ( -54.49181037333889321, 1.522049374736507144, -3.314263409011526385 ) ) ;
#1169=ORIENTED_EDGE ( 'NONE', *, *, #28931, .F. ) ;
#1177=EDGE_LOOP ( 'NONE', ( #22526, #8657, #22619, #30488 ) ) ;
#1181=ORIENTED_EDGE ( 'NONE', *, *, #20952, .T. ) ;
#1182=FACE_OUTER_BOUND ( 'NONE', #8330, .T. ) ;
#1185=DIRECTION ( 'NONE',  ( 1.000000000000000000, 2.586136946169074517E-16, -0.000000000000000000 ) ) ;
#1188=CARTESIAN_POINT ( 'NONE',  ( -54.44999999999997442, 0.000000000000000000, 4.650000000000000355 ) ) ;
#1190=CARTESIAN_POINT ( 'NONE',  ( 58.45000000000001705, -0.8000000000000000444, 1.778341924377873751 ) ) ;
#1203=ORIENTED_EDGE ( 'NONE', *, *, #21381, .T. ) ;
#1208=ORIENTED_EDGE ( 'NONE', *, *, #19680, .T. ) ;
#1210=CARTESIAN_POINT ( 'NONE',  ( 57.01262970566578758, -0.7335977677777304473, -1.792760110902297921 ) ) ;
#1212=DIRECTION ( 'NONE',  ( 1.000000000000000000, 2.586136946169074517E-16, -0.000000000000000000 ) ) ;
#1213=ORIENTED_EDGE ( 'NONE', *, *, #1304, .T. ) ;
#1214=AXIS2_PLACEMENT_3D ( 'NONE', #1245, #29438, #7751 ) ;
#1215=CARTESIAN_POINT ( 'NONE',  ( -36.31414349454750123, 4.927920137446164972, -1.660974799722044093 ) ) ;
#1218=CARTESIAN_POINT ( 'NONE',  ( -36.14490256869205353, -3.997744010329726816, 3.641645661657106903 ) ) ;
#1219=DIRECTION ( 'NONE',  ( 0.000000000000000000, -1.000000000000000000, -1.532429380227459806E-15 ) ) ;
#1221=DIRECTION ( 'NONE',  ( 0.000000000000000000, -1.000000000000000000, 0.000000000000000000 ) ) ;
#1222=CIRCLE ( 'NONE', #28022, 4.000000000000022204 ) ;
#1224=EDGE_LOOP ( 'NONE', ( #5036, #21057, #27990, #17078 ) ) ;
#1225=CARTESIAN_POINT ( 'NONE',  ( 15.94709373951304698, 2.670851142931325306, 4.702170608191319268 ) ) ;
#1230=CARTESIAN_POINT ( 'NONE',  ( -35.85663232820579793, 4.683225679163358635, -2.703237727951174119 ) ) ;
#1235=B_SPLINE_CURVE_WITH_KNOTS ( 'NONE', 3,
 ( #13102, #18341, #1218, #3609, #27837, #5829, #29892, #25767, #8204, #1386, #13391, #10879, #23090, #13717, #20411, #20568 ),
 .UNSPECIFIED., .F., .F.,
 ( 4, 2, 2, 2, 2, 2, 2, 4 ),
 ( 0.000000000000000000, 0.0004351083927046433489, 0.0008702167854092866979, 0.001740433570818574263, 0.002175541963523217829, 0.002610650356227860527, 0.003045758748932504093, 0.003480867141637147659 ),
 .UNSPECIFIED. ) ;
#1239=VECTOR ( 'NONE', #17750, 1000.000000000000000 ) ;
#1240=CARTESIAN_POINT ( 'NONE',  ( 50.42181344116571751, -1.309616516426922006, 3.885368734293527471 ) ) ;
#1241=CARTESIAN_POINT ( 'NONE',  ( 48.41306782696076993, 1.296871156637316114, 3.889656364559859192 ) ) ;
#1245=CARTESIAN_POINT ( 'NONE',  ( 57.05000000000001847, 0.8000000000000001554, 1.778341924377873973 ) ) ;
#1251=CIRCLE ( 'NONE', #7827, 0.05000000000000143219 ) ;
#1255=CIRCLE ( 'NONE', #22008, 0.1000000000000000472 ) ;
#1257=CARTESIAN_POINT ( 'NONE',  ( 47.00195600436720866, -4.143014423056512463, -1.077153443819862222 ) ) ;
#1259=CARTESIAN_POINT ( 'NONE',  ( 58.45000000000001705, 0.7500000000000000000, 1.778341924377873751 ) ) ;
#1260=CARTESIAN_POINT ( 'NONE',  ( 15.44631504820158874, 0.2166734227622383879, 5.199999998325004924 ) ) ;
#1270=EDGE_CURVE ( 'NONE', #13515, #9408, #13646, .T. ) ;
#1277=EDGE_CURVE ( 'NONE', #13977, #31086, #23503, .T. ) ;
#1282=( BOUNDED_SURFACE ( )  B_SPLINE_SURFACE ( 3, 2, ( 
 ( #8208, #18200, #22466 ),
 ( #20109, #29743, #12950 ),
 ( #27367, #5676, #20577 ),
 ( #27684, #15329, #13108 ),
 ( #13250, #1085, #8356 ),
 ( #1225, #5355, #15018 ),
 ( #22640, #27510, #24976 ),
 ( #608, #10734, #24681 ),
 ( #7890, #10269, #20417 ),
 ( #18036, #6005, #30209 ),
 ( #3616, #19938, #29569 ),
 ( #5525, #15179, #3147 ),
 ( #24831, #12787, #27842 ),
 ( #15946, #20732, #11529 ),
 ( #3926, #13721, #13571 ),
 ( #25773, #23099, #30676 ) ),
 .UNSPECIFIED., .F., .F., .F. ) 
 B_SPLINE_SURFACE_WITH_KNOTS ( ( 4, 2, 2, 2, 2, 2, 2, 4 ),
 ( 3, 3 ),
 ( 0.001780502285214191020, 0.002558945925323769834, 0.002753556835351164429, 0.002948167745378559024, 0.003337389565433348214, 0.003726611385488137838, 0.004115833205542927462, 0.004894276845652505842 ),
 ( 0.000000000000000000, 1.000000000000000000 ),
 .UNSPECIFIED. ) 
 GEOMETRIC_REPRESENTATION_ITEM ( )  RATIONAL_B_SPLINE_SURFACE ( (
 ( 1.000000000000000000, 0.9418517008537246049, 1.000000000000000000),
 ( 1.000000000000000000, 0.9417987965884757617, 1.000000000000000000),
 ( 1.000000000000000000, 0.9418198861734519145, 1.000000000000000000),
 ( 1.000000000000000000, 0.9434060303845467343, 1.000000000000000000),
 ( 1.000000000000000000, 0.9437939819948202302, 1.000000000000000000),
 ( 1.000000000000000000, 0.9445989566712769125, 1.000000000000000000),
 ( 1.000000000000000000, 0.9450169930049800993, 1.000000000000000000),
 ( 1.000000000000000000, 0.9461610507673693382, 1.000000000000000000),
 ( 1.000000000000000000, 0.9467217966427217135, 1.000000000000000000),
 ( 1.000000000000000000, 0.9467345476124366943, 1.000000000000000000),
 ( 1.000000000000000000, 0.9461964028052434195, 1.000000000000000000),
 ( 1.000000000000000000, 0.9446801822474353294, 1.000000000000000000),
 ( 1.000000000000000000, 0.9437582546536613659, 1.000000000000000000),
 ( 1.000000000000000000, 0.9418129560295538383, 1.000000000000000000),
 ( 1.000000000000000000, 0.9418016889777609535, 1.000000000000000000),
 ( 1.000000000000000000, 0.9418517008537241608, 1.000000000000000000) ) ) 
 REPRESENTATION_ITEM ( '' )  SURFACE ( )  );
#1284=CIRCLE ( 'NONE', #13906, 4.300000000000019362 ) ;
#1285=CARTESIAN_POINT ( 'NONE',  ( 47.10000000000002274, -3.826179070414207573, -1.000000000000000000 ) ) ;
#1287=CARTESIAN_POINT ( 'NONE',  ( 15.18463186935387554, 4.018128179617989737, -3.618665901676263896 ) ) ;
#1289=ORIENTED_EDGE ( 'NONE', *, *, #1134, .T. ) ;
#1293=ORIENTED_EDGE ( 'NONE', *, *, #6756, .F. ) ;
#1297=VERTEX_POINT ( 'NONE', #9102 ) ;
#1302=CARTESIAN_POINT ( 'NONE',  ( 56.95000000000001705, -0.6820512820512819596, -1.773360101234998210 ) ) ;
#1303=AXIS2_PLACEMENT_3D ( 'NONE', #19478, #1396, #29899 ) ;
#1304=EDGE_CURVE ( 'NONE', #2662, #9911, #23210, .T. ) ;
#1305=DIRECTION ( 'NONE',  ( -0.000000000000000000, -5.942513678379226626E-16, -1.000000000000000000 ) ) ;
#1314=CARTESIAN_POINT ( 'NONE',  ( 48.48125827213484484, -1.426739617975169905, 3.843750000000023537 ) ) ;
#1319=CIRCLE ( 'NONE', #830, 0.09999999999999986677 ) ;
#1327=CARTESIAN_POINT ( 'NONE',  ( 51.80000000000001847, -3.726179070414207040, -1.041421356237309581 ) ) ;
#1328=ORIENTED_EDGE ( 'NONE', *, *, #18494, .T. ) ;
#1331=CARTESIAN_POINT ( 'NONE',  ( 58.50000000000001421, 0.8000000000000000444, -1.778341924377873751 ) ) ;
#1334=AXIS2_PLACEMENT_3D ( 'NONE', #23771, #1731, #18861 ) ;
#1346=CARTESIAN_POINT ( 'NONE',  ( 15.90468948301721674, 2.602043737612613317, 4.741394629686831230 ) ) ;
#1348=EDGE_CURVE ( 'NONE', #31043, #14710, #13675, .T. ) ;
#1350=CIRCLE ( 'NONE', #6931, 1.000000000000000000 ) ;
#1351=EDGE_CURVE ( 'NONE', #1564, #30058, #17023, .T. ) ;
#1353=CARTESIAN_POINT ( 'NONE',  ( 57.05000000000001847, -0.7500000000000000000, 2.421260002560649660 ) ) ;
#1359=AXIS2_PLACEMENT_3D ( 'NONE', #25228, #8134, #15260 ) ;
#1365=EDGE_CURVE ( 'NONE', #18736, #6720, #22787, .T. ) ;
#1371=DIRECTION ( 'NONE',  ( 0.000000000000000000, 0.000000000000000000, -1.000000000000000000 ) ) ;
#1379=DIRECTION ( 'NONE',  ( 1.000000000000000000, 0.000000000000000000, 0.000000000000000000 ) ) ;
#1380=FACE_OUTER_BOUND ( 'NONE', #4096, .T. ) ;
#1383=CARTESIAN_POINT ( 'NONE',  ( -36.27260443516981780, 4.885888067249658739, -1.790336215468594894 ) ) ;
#1386=CARTESIAN_POINT ( 'NONE',  ( -36.79682133506353381, -2.710596767400086371, 4.680923748383016836 ) ) ;
#1388=VECTOR ( 'NONE', #20619, 1000.000000000000000 ) ;
#1393=CARTESIAN_POINT ( 'NONE',  ( 33.47623932017462778, 1.734723475976807094E-15, -4.375000000000000000 ) ) ;
#1396=DIRECTION ( 'NONE',  ( 0.000000000000000000, -0.9119702176296791141, -0.4102564102564098536 ) ) ;
#1400=CARTESIAN_POINT ( 'NONE',  ( 48.29999997184167881, 0.7900353715961344614, -4.025797886239747214 ) ) ;
#1406=CARTESIAN_POINT ( 'NONE',  ( 48.43940831342823117, 1.279117291415143853, 3.870058441400159754 ) ) ;
#1408=ORIENTED_EDGE ( 'NONE', *, *, #21117, .T. ) ;
#1410=DIRECTION ( 'NONE',  ( -0.000000000000000000, -1.000000000000000000, 0.000000000000000000 ) ) ;
#1413=DIRECTION ( 'NONE',  ( 1.000000000000000000, 0.000000000000000000, 0.000000000000000000 ) ) ;
#1414=ORIENTED_EDGE ( 'NONE', *, *, #7933, .F. ) ;
#1416=DIRECTION ( 'NONE',  ( 0.000000000000000000, -0.4102564102564100201, -0.9119702176296790030 ) ) ;
#1420=B_SPLINE_CURVE_WITH_KNOTS ( 'NONE', 3,
 ( #857, #29359, #15104, #27138, #24763, #12721, #5612, #25062, #3395, #13186, #22399, #20197 ),
 .UNSPECIFIED., .F., .F.,
 ( 4, 2, 2, 2, 2, 4 ),
 ( 0.000000000000000000, 5.522938194211729973E-05, 0.0001104587638842345995, 0.0002209175277684801765, 0.0004418350555369711949, 0.0008836701110739511719 ),
 .UNSPECIFIED. ) ;
#1423=CARTESIAN_POINT ( 'NONE',  ( 47.08054495771335013, -4.178364716350985830, -1.001910748144235308 ) ) ;
#1424=CARTESIAN_POINT ( 'NONE',  ( -36.23324115033477000, 3.272294129011982466, -4.050092634493898558 ) ) ;
#1426=PLANE ( 'NONE',  #20033 ) ;
#1429=CARTESIAN_POINT ( 'NONE',  ( -36.11780688638202008, 1.123735543663980208, -5.289358694936469263 ) ) ;
#1437=DIRECTION ( 'NONE',  ( 0.000000000000000000, 0.000000000000000000, -1.000000000000000000 ) ) ;
#1440=FACE_OUTER_BOUND ( 'NONE', #22331, .T. ) ;
#1447=ADVANCED_FACE ( 'NONE', ( #22244 ), #19856, .F. ) ;
#1449=CARTESIAN_POINT ( 'NONE',  ( 15.90468948301722918, 3.705258523861290509, -3.939862169952828452 ) ) ;
#1455=ORIENTED_EDGE ( 'NONE', *, *, #30812, .T. ) ;
#1456=FACE_OUTER_BOUND ( 'NONE', #29555, .T. ) ;
#1462=DIRECTION ( 'NONE',  ( 0.000000000000000000, 0.000000000000000000, -1.000000000000000000 ) ) ;
#1464=CARTESIAN_POINT ( 'NONE',  ( 57.05000000000001847, -0.7794871794871796045, -1.732743413496389939 ) ) ;
#1474=( BOUNDED_SURFACE ( )  B_SPLINE_SURFACE ( 3, 2, ( 
 ( #6266, #6430, #13691 ),
 ( #16090, #25570, #25741 ),
 ( #4049, #21477, #2759 ),
 ( #26692, #2464, #4989 ),
 ( #23846, #12408, #24158 ),
 ( #12121, #26368, #7211 ) ),
 .UNSPECIFIED., .F., .F., .F. ) 
 B_SPLINE_SURFACE_WITH_KNOTS ( ( 4, 2, 4 ),
 ( 3, 3 ),
 ( 0.0001437848949530132453, 0.0003024153973479680024, 0.0004610458997429227324 ),
 ( 0.000000000000000000, 1.000000000000000000 ),
 .UNSPECIFIED. ) 
 GEOMETRIC_REPRESENTATION_ITEM ( )  RATIONAL_B_SPLINE_SURFACE ( (
 ( 1.000000000000000000, 0.7071067811865723307, 1.000000000000000000),
 ( 1.000000000000000000, 0.7306243023312024576, 1.000000000000000000),
 ( 1.000000000000000000, 0.7490085278696598792, 1.000000000000000000),
 ( 1.000000000000000000, 0.7725095633943623863, 1.000000000000000000),
 ( 1.000000000000000000, 0.7779630306550003871, 1.000000000000000000),
 ( 1.000000000000000000, 0.7779866052154992273, 1.000000000000000000) ) ) 
 REPRESENTATION_ITEM ( '' )  SURFACE ( )  );
#1475=CARTESIAN_POINT ( 'NONE',  ( 57.00872446408695993, 0.7491456045391122753, -2.490007504536590588 ) ) ;
#1479=CARTESIAN_POINT ( 'NONE',  ( -54.49999999999997868, -6.938893903907228378E-14, 0.000000000000000000 ) ) ;
#1483=ORIENTED_EDGE ( 'NONE', *, *, #18154, .T. ) ;
#1489=EDGE_CURVE ( 'NONE', #14148, #10802, #5358, .T. ) ;
#1490=VERTEX_POINT ( 'NONE', #21073 ) ;
#1491=ORIENTED_EDGE ( 'NONE', *, *, #1862, .F. ) ;
#1493=CARTESIAN_POINT ( 'NONE',  ( 48.49151045397272242, -1.391941090707485396, 3.850000000000024070 ) ) ;
#1497=DIRECTION ( 'NONE',  ( 0.000000000000000000, 0.000000000000000000, -1.000000000000000000 ) ) ;
#1506=CARTESIAN_POINT ( 'NONE',  ( 15.03925126672132961, 2.199885893005915527, 4.939696249117695892 ) ) ;
#1510=LINE ( 'NONE', #4047, #10365 ) ;
#1511=AXIS2_PLACEMENT_3D ( 'NONE', #13170, #3373, #5266 ) ;
#1524=CARTESIAN_POINT ( 'NONE',  ( -36.58413561666602476, 3.095036031508457519, 4.435288302043179698 ) ) ;
#1528=EDGE_CURVE ( 'NONE', #28315, #6738, #5269, .T. ) ;
#1535=ORIENTED_EDGE ( 'NONE', *, *, #18081, .T. ) ;
#1536=CARTESIAN_POINT ( 'NONE',  ( -35.98994760229851408, 5.086913989685197812, -1.171642050077498665 ) ) ;
#1538=VECTOR ( 'NONE', #7234, 1000.000000000000000 ) ;
#1539=CARTESIAN_POINT ( 'NONE',  ( -35.85663232820584057, 2.199885893005902204, 4.939696249117695892 ) ) ;
#1540=CARTESIAN_POINT ( 'NONE',  ( 57.05000000000001137, 0.7500000000000000000, 1.746008434843730583 ) ) ;
#1545=CARTESIAN_POINT ( 'NONE',  ( 36.50000000000002132, 9.184850993605150903E-17, 0.7500000000000001110 ) ) ;
#1549=ORIENTED_EDGE ( 'NONE', *, *, #18038, .T. ) ;
#1553=CARTESIAN_POINT ( 'NONE',  ( 48.47204894654066010, 1.409900792624787513, 3.850000304694921827 ) ) ;
#1555=ORIENTED_EDGE ( 'NONE', *, *, #533, .T. ) ;
#1559=EDGE_CURVE ( 'NONE', #3444, #19303, #1222, .T. ) ;
#1563=DIRECTION ( 'NONE',  ( 0.000000000000000000, 0.000000000000000000, -1.000000000000000000 ) ) ;
#1564=VERTEX_POINT ( 'NONE', #5200 ) ;
#1571=VERTEX_POINT ( 'NONE', #19638 ) ;
#1572=ADVANCED_FACE ( 'NONE', ( #4893 ), #27035, .T. ) ;
#1581=CYLINDRICAL_SURFACE ( 'NONE', #862, 1.000000000000000000 ) ;
#1584=VECTOR ( 'NONE', #2324, 1000.000000000000000 ) ;
#1588=CARTESIAN_POINT ( 'NONE',  ( 15.74504787372211290, -5.206628483174585931, 1.466363261642503302 ) ) ;
#1591=FACE_OUTER_BOUND ( 'NONE', #3116, .T. ) ;
#1592=ADVANCED_FACE ( 'NONE', ( #2680 ), #9968, .F. ) ;
#1595=ORIENTED_EDGE ( 'NONE', *, *, #21006, .T. ) ;
#1613=DIRECTION ( 'NONE',  ( 1.520093157366878429E-16, -0.5877852522924742473, 0.8090169943749465631 ) ) ;
#1617=CARTESIAN_POINT ( 'NONE',  ( 56.97364842551142061, 0.7795706648299629560, 2.480376902516343129 ) ) ;
#1619=CARTESIAN_POINT ( 'NONE',  ( 50.39884346364546985, 0.8930148142854623661, -3.925689827643446428 ) ) ;
#1626=CARTESIAN_POINT ( 'NONE',  ( 58.45000000000001705, 0.8000000000000000444, 1.778341924377873751 ) ) ;
#1630=ORIENTED_EDGE ( 'NONE', *, *, #27322, .T. ) ;
#1643=CARTESIAN_POINT ( 'NONE',  ( 47.06862320199297756, -4.259946794064910058, -1.000000024775397289 ) ) ;
#1645=CARTESIAN_POINT ( 'NONE',  ( -45.15971931043468146, 4.700000000000000178, 0.000000000000000000 ) ) ;
#1647=CARTESIAN_POINT ( 'NONE',  ( 15.32752150720753725, 3.997744010329658426, 3.641645661657159749 ) ) ;
#1650=CARTESIAN_POINT ( 'NONE',  ( -36.27260443516977517, -2.900433254921178428, 4.320265374240116252 ) ) ;
#1655=DIRECTION ( 'NONE',  ( 0.000000000000000000, 0.000000000000000000, 1.000000000000000000 ) ) ;
#1658=ORIENTED_EDGE ( 'NONE', *, *, #20916, .T. ) ;
#1664=ADVANCED_FACE ( 'NONE', ( #29419 ), #7881, .T. ) ;
#1668=CARTESIAN_POINT ( 'NONE',  ( -36.92443669619590452, 3.051830235923023604, 4.466755975380251265 ) ) ;
#1672=CYLINDRICAL_SURFACE ( 'NONE', #20988, 4.100000000000022737 ) ;
#1674=DIRECTION ( 'NONE',  ( 0.000000000000000000, -1.000000000000000000, 0.000000000000000000 ) ) ;
#1680=DIRECTION ( 'NONE',  ( -1.000000000000000000, 0.000000000000000000, 0.000000000000000000 ) ) ;
#1687=CARTESIAN_POINT ( 'NONE',  ( 50.40000000000001279, 0.7711297561636268894, -3.938774833552663335 ) ) ;
#1688=EDGE_CURVE ( 'NONE', #3021, #30927, #2747, .T. ) ;
#1691=ADVANCED_FACE ( 'NONE', ( #2535, #12183 ), #29117, .T. ) ;
#1694=CARTESIAN_POINT ( 'NONE',  ( -36.21152527658243514, 0.2904410314644398361, 5.200000000384614296 ) ) ;
#1696=VERTEX_POINT ( 'NONE', #18198 ) ;
#1698=ORIENTED_EDGE ( 'NONE', *, *, #22069, .F. ) ;
#1700=CARTESIAN_POINT ( 'NONE',  ( 48.39328721529930277, 1.343285922954075007, 3.873819829599202791 ) ) ;
#1706=CARTESIAN_POINT ( 'NONE',  ( -44.49999999999997868, 1.499999999999999556, -4.029888335921975262 ) ) ;
#1708=CARTESIAN_POINT ( 'NONE',  ( 58.45000000000001705, 0.7500000000000000000, -1.745709025009608784 ) ) ;
#1709=VERTEX_POINT ( 'NONE', #20571 ) ;
#1720=CARTESIAN_POINT ( 'NONE',  ( 57.04306286658350444, -0.7495164233357125561, 1.778776689171566172 ) ) ;
#1721=CARTESIAN_POINT ( 'NONE',  ( -36.89250464418361020, 3.430438802933478470, -4.182416543699397415 ) ) ;
#1723=AXIS2_PLACEMENT_3D ( 'NONE', #11069, #8535, #18221 ) ;
#1727=CARTESIAN_POINT ( 'NONE',  ( 16.08093158123429234, 0.2888463313200336779, -5.401384060636564399 ) ) ;
#1730=AXIS2_PLACEMENT_3D ( 'NONE', #7436, #14709, #22794 ) ;
#1731=DIRECTION ( 'NONE',  ( 1.000000000000000000, 0.000000000000000000, 0.000000000000000000 ) ) ;
#1738=CARTESIAN_POINT ( 'NONE',  ( -36.11780688638068426, 4.683225673667265276, 2.703237737472885538 ) ) ;
#1739=CARTESIAN_POINT ( 'NONE',  ( 15.66436536804551771, -5.256245472275819175, 1.286369972357283675 ) ) ;
#1740=( GEOMETRIC_REPRESENTATION_CONTEXT ( 3 ) GLOBAL_UNCERTAINTY_ASSIGNED_CONTEXT ( ( #4743 ) ) GLOBAL_UNIT_ASSIGNED_CONTEXT ( ( #18140, #23030, #8747 ) ) REPRESENTATION_CONTEXT ( 'NONE', 'WORKASPACE' ) );
#1741=EDGE_LOOP ( 'NONE', ( #26496, #6868, #28975, #18320 ) ) ;
#1744=CARTESIAN_POINT ( 'NONE',  ( 48.37818655883430807, 1.309616516426969302, 3.885368734293527471 ) ) ;
#1746=ADVANCED_FACE ( 'NONE', ( #13104 ), #15655, .F. ) ;
#1748=AXIS2_PLACEMENT_3D ( 'NONE', #12275, #19279, #14185 ) ;
#1749=CARTESIAN_POINT ( 'NONE',  ( -35.85663232820583346, -3.817150320980530864, 2.203324261490918090 ) ) ;
#1759=ORIENTED_EDGE ( 'NONE', *, *, #20992, .T. ) ;
#1771=VECTOR ( 'NONE', #23692, 1000.000000000000000 ) ;
#1772=CARTESIAN_POINT ( 'NONE',  ( 16.07279755198653604, 5.235729994560204048, -1.359191621353886159 ) ) ;
#1778=CARTESIAN_POINT ( 'NONE',  ( 15.03925126672132784, 3.817150320980643663, 2.203324261490567704 ) ) ;
#1782=CARTESIAN_POINT ( 'NONE',  ( 51.80000000000001847, -3.726179070414207928, 1.100000000000000533 ) ) ;
#1787=VERTEX_POINT ( 'NONE', #18624 ) ;
#1790=ORIENTED_EDGE ( 'NONE', *, *, #24377, .F. ) ;
#1800=VERTEX_POINT ( 'NONE', #1645 ) ;
#1813=AXIS2_PLACEMENT_3D ( 'NONE', #13875, #30364, #15808 ) ;
#1814=CARTESIAN_POINT ( 'NONE',  ( 57.03906491987265781, 0.7487895892850940927, -1.779428968492786867 ) ) ;
#1823=FACE_OUTER_BOUND ( 'NONE', #28727, .T. ) ;
#1830=CARTESIAN_POINT ( 'NONE',  ( 51.85588625589981859, 0.1560022812617363475, -4.362189373992536368 ) ) ;
#1832=AXIS2_PLACEMENT_3D ( 'NONE', #11958, #30628, #30802 ) ;
#1836=CARTESIAN_POINT ( 'NONE',  ( -36.38139716712170468, 2.291889356119548804, 4.901871067649744340 ) ) ;
#1837=ORIENTED_EDGE ( 'NONE', *, *, #11563, .T. ) ;
#1838=LINE ( 'NONE', #21016, #12869 ) ;
#1842=DIRECTION ( 'NONE',  ( -1.000000000000000000, 0.000000000000000000, 0.000000000000000000 ) ) ;
#1844=AXIS2_PLACEMENT_3D ( 'NONE', #9808, #26758, #28820 ) ;
#1851=CARTESIAN_POINT ( 'NONE',  ( -35.85663232820584057, 1.123735532908267665, -5.289358697221546279 ) ) ;
#1856=CARTESIAN_POINT ( 'NONE',  ( 51.86925381625176357, 0.07373004000955572790, 4.369615861601171325 ) ) ;
#1860=DIRECTION ( 'NONE',  ( -1.000000000000000000, 0.000000000000000000, 0.000000000000000000 ) ) ;
#1861=AXIS2_PLACEMENT_3D ( 'NONE', #24937, #17517, #2537 ) ;
#1862=EDGE_CURVE ( 'NONE', #15671, #16732, #14052, .T. ) ;
#1867=ORIENTED_EDGE ( 'NONE', *, *, #22678, .T. ) ;
#1868=CIRCLE ( 'NONE', #21107, 2.549999999999999822 ) ;
#1872=CARTESIAN_POINT ( 'NONE',  ( -36.30424252565905618, -0.1108756495952975957, 5.200000001675011418 ) ) ;
#1878=ORIENTED_EDGE ( 'NONE', *, *, #11695, .T. ) ;
#1886=CIRCLE ( 'NONE', #27175, 0.05000000000000005829 ) ;
#1902=LINE ( 'NONE', #31188, #22603 ) ;
#1904=CARTESIAN_POINT ( 'NONE',  ( -36.31440869660544735, 3.100731772197836911, -4.174739983989952385 ) ) ;
#1905=EDGE_CURVE ( 'NONE', #15713, #3198, #25367, .T. ) ;
#1907=CARTESIAN_POINT ( 'NONE',  ( -35.85663232820584057, -1.854603232583471356E-14, -5.200000000000000178 ) ) ;
#1913=CARTESIAN_POINT ( 'NONE',  ( 50.33046473658142617, -1.366509374015013600, -3.854674997130604908 ) ) ;
#1914=ORIENTED_EDGE ( 'NONE', *, *, #8510, .F. ) ;
#1916=CARTESIAN_POINT ( 'NONE',  ( -54.44999999999997442, -6.938893903907228378E-14, 0.000000000000000000 ) ) ;
#1923=CARTESIAN_POINT ( 'NONE',  ( 48.34316787720665332, 1.211455355144567703, 3.917539841352833285 ) ) ;
#1924=CARTESIAN_POINT ( 'NONE',  ( 50.34656340841117839, -1.329326705022595201, 3.861343257506214766 ) ) ;
#1935=VERTEX_POINT ( 'NONE', #19094 ) ;
#1941=CARTESIAN_POINT ( 'NONE',  ( 57.01810253486932112, -0.8103601741748552856, 2.470489098966295316 ) ) ;
#1942=DIRECTION ( 'NONE',  ( 0.000000000000000000, 0.000000000000000000, -1.000000000000000000 ) ) ;
#1946=( BOUNDED_SURFACE ( )  B_SPLINE_SURFACE ( 3, 2, ( 
 ( #18514, #3770, #28157 ),
 ( #15673, #20889, #13409 ),
 ( #20745, #30055, #22811 ),
 ( #1097, #3940, #6310 ),
 ( #25624, #16295, #22951 ),
 ( #1406, #1241, #27996 ),
 ( #20431, #8676, #1700 ),
 ( #30694, #25320, #8369 ),
 ( #13581, #1553, #6478 ),
 ( #28325, #11216, #13732 ) ),
 .UNSPECIFIED., .F., .F., .F. ) 
 B_SPLINE_SURFACE_WITH_KNOTS ( ( 4, 2, 2, 2, 4 ),
 ( 3, 3 ),
 ( 0.0004005301535625022482, 0.0008279283193725973976, 0.001041627402277645054, 0.001148476943730168936, 0.001255326485182692601 ),
 ( 0.000000000000000000, 1.000000000000000000 ),
 .UNSPECIFIED. ) 
 GEOMETRIC_REPRESENTATION_ITEM ( )  RATIONAL_B_SPLINE_SURFACE ( (
 ( 1.000000000000000000, 0.7071067811865260344, 1.000000000000000000),
 ( 1.000000000000000000, 0.7463463187144947497, 1.000000000000000000),
 ( 1.000000000000000000, 0.7946150999565809725, 1.000000000000000000),
 ( 1.000000000000000000, 0.8720431506958414847, 1.000000000000000000),
 ( 1.000000000000000000, 0.8987780092778684393, 1.000000000000000000),
 ( 1.000000000000000000, 0.9375340664365204857, 1.000000000000000000),
 ( 1.000000000000000000, 0.9504270566176279411, 1.000000000000000000),
 ( 1.000000000000000000, 0.9732249474031190450, 1.000000000000000000),
 ( 1.000000000000000000, 0.9839441327696822892, 1.000000000000000000),
 ( 1.000000000000000000, 0.9842509842514762797, 1.000000000000000000) ) ) 
 REPRESENTATION_ITEM ( '' )  SURFACE ( )  );
#1949=CARTESIAN_POINT ( 'NONE',  ( 57.05000000000001847, 0.7500000000000000000, -2.489477856900920383 ) ) ;
#1951=CARTESIAN_POINT ( 'NONE',  ( 15.44259799936806488, 5.012895491272638893, -1.399447560527434797 ) ) ;
#1955=ORIENTED_EDGE ( 'NONE', *, *, #9126, .T. ) ;
#1972=CARTESIAN_POINT ( 'NONE',  ( 51.80000000000001847, -0.2842225609755594795, -1.577752156565102655E-15 ) ) ;
#1973=ADVANCED_FACE ( 'NONE', ( #26683 ), #14477, .F. ) ;
#1978=LINE ( 'NONE', #26031, #19825 ) ;
#1981=ORIENTED_EDGE ( 'NONE', *, *, #21499, .T. ) ;
#1987=DIRECTION ( 'NONE',  ( -1.000000000000000000, 0.000000000000000000, 0.000000000000000000 ) ) ;
#1988=DIRECTION ( 'NONE',  ( 0.000000000000000000, 0.000000000000000000, 1.000000000000000000 ) ) ;
#1989=DIRECTION ( 'NONE',  ( 0.000000000000000000, -0.000000000000000000, 1.000000000000000000 ) ) ;
#1990=DIRECTION ( 'NONE',  ( 0.000000000000000000, 0.000000000000000000, -1.000000000000000000 ) ) ;
#1993=VERTEX_POINT ( 'NONE', #10515 ) ;
#1995=VERTEX_POINT ( 'NONE', #22717 ) ;
#1999=CARTESIAN_POINT ( 'NONE',  ( -36.22955757456080761, 3.272340825137115772, 4.050058705652215707 ) ) ;
#2002=ORIENTED_EDGE ( 'NONE', *, *, #26851, .F. ) ;
#2003=ADVANCED_FACE ( 'NONE', ( #27591 ), #10192, .T. ) ;
#2007=CARTESIAN_POINT ( 'NONE',  ( 50.45688046812396976, 1.211457450596386209, 3.917546004217189015 ) ) ;
#2009=VERTEX_POINT ( 'NONE', #24598 ) ;
#2012=AXIS2_PLACEMENT_3D ( 'NONE', #25284, #1371, #27494 ) ;
#2014=AXIS2_PLACEMENT_3D ( 'NONE', #25807, #25484, #8694 ) ;
#2018=VECTOR ( 'NONE', #20215, 1000.000000000000000 ) ;
#2025=FACE_OUTER_BOUND ( 'NONE', #23862, .T. ) ;
#2026=CARTESIAN_POINT ( 'NONE',  ( -36.22909104983144601, -0.6969927240738240659, 5.374332520738271057 ) ) ;
#2028=ORIENTED_EDGE ( 'NONE', *, *, #11758, .F. ) ;
#2029=CARTESIAN_POINT ( 'NONE',  ( -36.79682133506353381, -4.944296796129610705, 2.193698057025720072 ) ) ;
#2044=CARTESIAN_POINT ( 'NONE',  ( 33.47623932017462778, 1.123735532908310519, 5.289358697221540950 ) ) ;
#2046=EDGE_CURVE ( 'NONE', #11900, #27954, #16272, .T. ) ;
#2050=CARTESIAN_POINT ( 'NONE',  ( -54.44999999999997442, 1.499999999999999556, -4.029888335921975262 ) ) ;
#2054=CARTESIAN_POINT ( 'NONE',  ( -36.27260443516960464, 2.900433254920971038, -4.320265374240186418 ) ) ;
#2055=LINE ( 'NONE', #9194, #17675 ) ;
#2056=B_SPLINE_CURVE_WITH_KNOTS ( 'NONE', 3,
 ( #26685, #6729, #21326, #11956, #14168, #23693, #26510, #26362, #21796, #23990, #9273, #16872, #12258, #18937, #82, #7208 ),
 .UNSPECIFIED., .F., .F.,
 ( 4, 3, 3, 3, 3, 4 ),
 ( 0.000000000000000000, 3.111139534546023401E-05, 6.583698738123831937E-05, 9.811465807641186142E-05, 0.0001294159172546408877, 0.0001609582457662007114 ),
 .UNSPECIFIED. ) ;
#2058=VECTOR ( 'NONE', #19470, 1000.000000000000000 ) ;
#2059=CARTESIAN_POINT ( 'NONE',  ( 57.02528775048638465, -0.7434661330690420789, -2.425538622349843632 ) ) ;
#2061=DIRECTION ( 'NONE',  ( 0.000000000000000000, -1.626303258728255862E-15, 1.000000000000000000 ) ) ;
#2064=CARTESIAN_POINT ( 'NONE',  ( -44.49999999999997868, 1.499999999999998890, 3.300094695611021756 ) ) ;
#2066=ORIENTED_EDGE ( 'NONE', *, *, #28274, .F. ) ;
#2069=CARTESIAN_POINT ( 'NONE',  ( 15.29384114148407647, -2.734418404389891144, -4.440882220947494297 ) ) ;
#2076=CARTESIAN_POINT ( 'NONE',  ( 56.96117471280891209, 0.7619384116854249767, -2.485869561276773165 ) ) ;
#2094=DIRECTION ( 'NONE',  ( 0.000000000000000000, -8.673617379884032317E-15, -1.000000000000000000 ) ) ;
#2098=CARTESIAN_POINT ( 'NONE',  ( 15.29954477411490821, 5.377732435184259252, -0.5657657035920871103 ) ) ;
#2100=DIRECTION ( 'NONE',  ( 1.000000000000000000, 0.000000000000000000, 0.000000000000000000 ) ) ;
#2102=CARTESIAN_POINT ( 'NONE',  ( 50.40000000000001990, 0.6304760106459518232, -3.950000000000022826 ) ) ;
#2104=CARTESIAN_POINT ( 'NONE',  ( 48.37840743871460347, -1.310166284604358244, 3.885185101012172737 ) ) ;
#2105=CARTESIAN_POINT ( 'NONE',  ( 50.34875358082581442, -1.383300983803858797, 3.859740869727655621 ) ) ;
#2107=DIRECTION ( 'NONE',  ( 1.000000000000000000, 0.000000000000000000, 0.000000000000000000 ) ) ;
#2108=AXIS2_PLACEMENT_3D ( 'NONE', #10341, #20014, #7982 ) ;
#2113=ORIENTED_EDGE ( 'NONE', *, *, #18597, .F. ) ;
#2121=EDGE_LOOP ( 'NONE', ( #1483, #30560, #19045, #30745 ) ) ;
#2122=DIRECTION ( 'NONE',  ( -1.000000000000000000, 0.000000000000000000, 0.000000000000000000 ) ) ;
#2124=CARTESIAN_POINT ( 'NONE',  ( 54.40000000000001990, 0.000000000000000000, -3.299999999999999822 ) ) ;
#2136=CARTESIAN_POINT ( 'NONE',  ( 50.40000000000001990, -4.899999999999999467, -4.100000000000022737 ) ) ;
#2137=EDGE_CURVE ( 'NONE', #22777, #5429, #20332, .T. ) ;
#2140=CARTESIAN_POINT ( 'NONE',  ( 34.50000000000001421, 0.000000000000000000, 0.000000000000000000 ) ) ;
#2141=CARTESIAN_POINT ( 'NONE',  ( 58.50000000000001421, 0.8000000000000000444, 2.421260002560649660 ) ) ;
#2143=ORIENTED_EDGE ( 'NONE', *, *, #12156, .T. ) ;
#2144=ORIENTED_EDGE ( 'NONE', *, *, #28819, .F. ) ;
#2145=DIRECTION ( 'NONE',  ( 0.000000000000000000, 0.000000000000000000, 1.000000000000000000 ) ) ;
#2146=ORIENTED_EDGE ( 'NONE', *, *, #31322, .T. ) ;
#2151=CARTESIAN_POINT ( 'NONE',  ( -36.56390771145526486, 3.008101665203156028, 4.495550615867659694 ) ) ;
#2158=CARTESIAN_POINT ( 'NONE',  ( 50.39865716130687190, 0.9106118309513187015, 3.923752762110599424 ) ) ;
#2162=CARTESIAN_POINT ( 'NONE',  ( 57.05000000000001847, 0.7500000000000000000, 1.778341924377873751 ) ) ;
#2163=CARTESIAN_POINT ( 'NONE',  ( -54.49983832461118283, -1.542920080254277959, -3.327619142904491234 ) ) ;
#2167=CARTESIAN_POINT ( 'NONE',  ( 56.95000000000001705, 0.000000000000000000, 0.000000000000000000 ) ) ;
#2169=AXIS2_PLACEMENT_3D ( 'NONE', #4645, #17626, #19994 ) ;
#2171=EDGE_CURVE ( 'NONE', #19277, #10332, #22348, .T. ) ;
#2174=CARTESIAN_POINT ( 'NONE',  ( 57.05000000000001137, -0.7500000000000000000, -2.421260002560653213 ) ) ;
#2175=CARTESIAN_POINT ( 'NONE',  ( -36.04581030752768811, -0.7747498452693805104, 5.363501451415725541 ) ) ;
#2178=CARTESIAN_POINT ( 'NONE',  ( -54.47328085509070661, 1.505517457405397996, 4.033720452520547894 ) ) ;
#2180=CARTESIAN_POINT ( 'NONE',  ( 15.44259799936805422, 0.2181161761757584028, -5.200000001420963969 ) ) ;
#2193=CYLINDRICAL_SURFACE ( 'NONE', #27936, 0.04999999999999991257 ) ;
#2194=CARTESIAN_POINT ( 'NONE',  ( -37.18272003341174070, -1.653865106024005477E-14, 0.000000000000000000 ) ) ;
#2198=DIRECTION ( 'NONE',  ( 0.000000000000000000, 0.000000000000000000, 1.000000000000000000 ) ) ;
#2199=DIRECTION ( 'NONE',  ( 1.000000000000000000, 0.000000000000000000, -4.738179285253022937E-16 ) ) ;
#2200=EDGE_CURVE ( 'NONE', #11901, #24741, #8672, .T. ) ;
#2202=CARTESIAN_POINT ( 'NONE',  ( 57.00320971560400096, -0.7176258130632211518, 1.806074485252040285 ) ) ;
#2207=CARTESIAN_POINT ( 'NONE',  ( 57.03559403007977124, -0.7482252654948684523, -2.422430812887707230 ) ) ;
#2216=ORIENTED_EDGE ( 'NONE', *, *, #635, .T. ) ;
#2217=LINE ( 'NONE', #11881, #7261 ) ;
#2221=CARTESIAN_POINT ( 'NONE',  ( 16.07512358269929464, -5.037778396015496263, 1.970103387724016386 ) ) ;
#2227=CARTESIAN_POINT ( 'NONE',  ( 57.02825620192501077, 0.8138444489294278661, -2.469346200785457413 ) ) ;
#2232=SURFACE_STYLE_FILL_AREA ( #21893 ) ;
#2239=CARTESIAN_POINT ( 'NONE',  ( -54.44999999999997442, 5.755839955992559655E-16, -4.700000000000000178 ) ) ;
#2242=DIRECTION ( 'NONE',  ( 0.000000000000000000, -1.000000000000000000, 0.000000000000000000 ) ) ;
#2244=EDGE_CURVE ( 'NONE', #19839, #15713, #16035, .T. ) ;
#2245=CARTESIAN_POINT ( 'NONE',  ( 15.03925126672132961, 1.123735532908280765, -5.289358697221546279 ) ) ;
#2246=CARTESIAN_POINT ( 'NONE',  ( -35.85663232820584057, -3.056483311920867862, 4.206888370749728878 ) ) ;
#2251=PLANE ( 'NONE',  #17506 ) ;
#2253=VERTEX_POINT ( 'NONE', #26633 ) ;
#2255=AXIS2_PLACEMENT_3D ( 'NONE', #14695, #24356, #31005 ) ;
#2257=CARTESIAN_POINT ( 'NONE',  ( 48.37893541770432648, -0.9199776782965987110, 3.998258245321878235 ) ) ;
#2258=CARTESIAN_POINT ( 'NONE',  ( 50.40896409817931101, -1.199904535326220767, 3.921111011342365060 ) ) ;
#2261=EDGE_CURVE ( 'NONE', #24391, #2569, #19237, .T. ) ;
#2262=EDGE_LOOP ( 'NONE', ( #1555, #13342, #20827, #1981 ) ) ;
#2265=CARTESIAN_POINT ( 'NONE',  ( -43.84599839145305111, 4.786668705877430874, 0.000000000000000000 ) ) ;
#2268=ORIENTED_EDGE ( 'NONE', *, *, #21431, .T. ) ;
#2278=EDGE_CURVE ( 'NONE', #4498, #9785, #4044, .T. ) ;
#2281=ORIENTED_EDGE ( 'NONE', *, *, #4470, .F. ) ;
#2283=ADVANCED_FACE ( 'NONE', ( #7016 ), #29163, .T. ) ;
#2298=ORIENTED_EDGE ( 'NONE', *, *, #16497, .F. ) ;
#2301=ORIENTED_EDGE ( 'NONE', *, *, #27476, .F. ) ;
#2306=CARTESIAN_POINT ( 'NONE',  ( -35.85663232820584057, 2.686240680702099759, 4.475885388010746979 ) ) ;
#2309=VERTEX_POINT ( 'NONE', #24103 ) ;
#2315=ORIENTED_EDGE ( 'NONE', *, *, #3799, .T. ) ;
#2321=CARTESIAN_POINT ( 'NONE',  ( 57.00000000000001421, 0.6999999999999999556, 1.820027472320129736 ) ) ;
#2324=DIRECTION ( 'NONE',  ( 1.000000000000000000, 2.586136946169074517E-16, -0.000000000000000000 ) ) ;
#2331=CARTESIAN_POINT ( 'NONE',  ( 57.05000000000001847, 0.7500000000000000000, -1.778341924377873751 ) ) ;
#2334=AXIS2_PLACEMENT_3D ( 'NONE', #29970, #27291, #5607 ) ;
#2336=VECTOR ( 'NONE', #6657, 1000.000000000000000 ) ;
#2338=CARTESIAN_POINT ( 'NONE',  ( -36.92398358572908990, -0.2875137064282174415, 5.407399902318747564 ) ) ;
#2339=ORIENTED_EDGE ( 'NONE', *, *, #5681, .F. ) ;
#2340=CARTESIAN_POINT ( 'NONE',  ( 56.95000000000001705, 0.6820512820512819596, 1.773360101234998210 ) ) ;
#2341=CARTESIAN_POINT ( 'NONE',  ( 57.05000000000001847, -0.7794871794871796045, 1.732743413496389939 ) ) ;
#2345=SPHERICAL_SURFACE ( 'NONE', #167, 0.05000000000000000278 ) ;
#2346=ORIENTED_EDGE ( 'NONE', *, *, #30119, .T. ) ;
#2347=CARTESIAN_POINT ( 'NONE',  ( 15.41217651307626291, 0.2668145608218919218, -5.199999998579035498 ) ) ;
#2354=AXIS2_PLACEMENT_3D ( 'NONE', #28391, #16518, #7178 ) ;
#2356=DIRECTION ( 'NONE',  ( 0.000000000000000000, 0.000000000000000000, -1.000000000000000000 ) ) ;
#2360=CARTESIAN_POINT ( 'NONE',  ( 57.00000000000001421, 0.6999999999999999556, 2.452039967047845437 ) ) ;
#2363=AXIS2_PLACEMENT_3D ( 'NONE', #7095, #24024, #28929 ) ;
#2374=CIRCLE ( 'NONE', #4401, 1.899999999999999911 ) ;
#2381=DIRECTION ( 'NONE',  ( 0.000000000000000000, -1.000000000000000000, 0.000000000000000000 ) ) ;
#2382=DIRECTION ( 'NONE',  ( -1.000000000000000000, -2.586136946169074517E-16, 0.000000000000000000 ) ) ;
#2384=VECTOR ( 'NONE', #15364, 1000.000000000000000 ) ;
#2385=CARTESIAN_POINT ( 'NONE',  ( 58.45000000000001705, 0.8000000000000000444, -2.471260002560649927 ) ) ;
#2392=CARTESIAN_POINT ( 'NONE',  ( -36.04581030752630255, 4.861582136949842869, 2.394243986683832315 ) ) ;
#2394=EDGE_LOOP ( 'NONE', ( #27307, #9449, #29332, #27452 ) ) ;
#2395=ORIENTED_EDGE ( 'NONE', *, *, #12678, .F. ) ;
#2396=CARTESIAN_POINT ( 'NONE',  ( 50.30000000000001847, 1.391941090707534023, -3.750000000000022649 ) ) ;
#2398=DIRECTION ( 'NONE',  ( 1.000000000000000000, -0.000000000000000000, -0.000000000000000000 ) ) ;
#2402=CARTESIAN_POINT ( 'NONE',  ( -36.23324115033477710, -4.863061488092512263, -1.860589201779685231 ) ) ;
#2403=ORIENTED_EDGE ( 'NONE', *, *, #2856, .F. ) ;
#2404=VECTOR ( 'NONE', #21854, 1000.000000000000000 ) ;
#2418=EDGE_CURVE ( 'NONE', #14402, #20590, #21249, .T. ) ;
#2420=CARTESIAN_POINT ( 'NONE',  ( -36.92443669619682112, 0.1565107631086873063, -5.407502298984291578 ) ) ;
#2423=CARTESIAN_POINT ( 'NONE',  ( 47.06870114826936913, -4.259946762565045120, 1.000000153509832179 ) ) ;
#2428=AXIS2_PLACEMENT_3D ( 'NONE', #27057, #28981, #2556 ) ;
#2430=CARTESIAN_POINT ( 'NONE',  ( 15.03925126672132961, -0.4576450603546987628, 5.200000000000000178 ) ) ;
#2431=CARTESIAN_POINT ( 'NONE',  ( 48.42155979508061137, -1.181909706220196643, 3.885998080850099790 ) ) ;
#2432=CARTESIAN_POINT ( 'NONE',  ( 50.30000000000001847, -1.409901620910170017, 3.850000000000021849 ) ) ;
#2435=ORIENTED_EDGE ( 'NONE', *, *, #10032, .F. ) ;
#2457=DIRECTION ( 'NONE',  ( 0.000000000000000000, -1.000000000000000000, 0.000000000000000000 ) ) ;
#2464=CARTESIAN_POINT ( 'NONE',  ( 51.76226673693759039, -4.256154442720826658, 1.015631899367400948 ) ) ;
#2479=CARTESIAN_POINT ( 'NONE',  ( 50.40000000000001990, -4.899999999999999467, 4.100000000000022737 ) ) ;
#2485=EDGE_LOOP ( 'NONE', ( #8470, #10363, #14101, #4533 ) ) ;
#2486=CARTESIAN_POINT ( 'NONE',  ( -36.92398358572908990, 5.053896291911939009, 1.944420249220693675 ) ) ;
#2487=ADVANCED_FACE ( 'NONE', ( #17602 ), #14936, .T. ) ;
#2489=CARTESIAN_POINT ( 'NONE',  ( 56.95000076968187130, -0.7321971888534951622, 1.754073505128400878 ) ) ;
#2491=CARTESIAN_POINT ( 'NONE',  ( 57.03449256411899881, 0.7475344026195360758, 1.780552047803072302 ) ) ;
#2492=CARTESIAN_POINT ( 'NONE',  ( -35.85663232820583346, -4.817150320980683631, 2.203324261490539282 ) ) ;
#2497=DIRECTION ( 'NONE',  ( 0.000000000000000000, 0.000000000000000000, 1.000000000000000000 ) ) ;
#2498=CARTESIAN_POINT ( 'NONE',  ( 50.32795105345940101, 1.409900792624783294, -3.850000304694921827 ) ) ;
#2499=CARTESIAN_POINT ( 'NONE',  ( 15.59055531549694429, -5.360541651686761000, -0.7128348320084266776 ) ) ;
#2500=CARTESIAN_POINT ( 'NONE',  ( -36.72207054450174724, 0.6818242347930701941, 5.365311767243446717 ) ) ;
#2505=CARTESIAN_POINT ( 'NONE',  ( -36.23324115033477710, -2.840672495176407075, -4.363684107482597163 ) ) ;
#2507=CYLINDRICAL_SURFACE ( 'NONE', #7444, 0.1000000000000000472 ) ;
#2515=CARTESIAN_POINT ( 'NONE',  ( 15.03925126672122836, 1.123735532908292312, -5.289358697221543615 ) ) ;
#2516=CARTESIAN_POINT ( 'NONE',  ( -36.11122220296839203, -4.822476035523795446, 1.985498375066742982 ) ) ;
#2518=FACE_OUTER_BOUND ( 'NONE', #27815, .T. ) ;
#2519=ORIENTED_EDGE ( 'NONE', *, *, #8623, .T. ) ;
#2523=DIRECTION ( 'NONE',  ( 0.000000000000000000, -1.000000000000000000, 0.000000000000000000 ) ) ;
#2525=CARTESIAN_POINT ( 'NONE',  ( -54.49999516060625382, -1.549196738101655368, -4.063926895246979143 ) ) ;
#2531=AXIS2_PLACEMENT_3D ( 'NONE', #20331, #12549, #15089 ) ;
#2534=CARTESIAN_POINT ( 'NONE',  ( -35.85663232820584057, 1.793057972834477765, -4.026191436120592826 ) ) ;
#2535=FACE_OUTER_BOUND ( 'NONE', #11935, .T. ) ;
#2537=DIRECTION ( 'NONE',  ( 0.000000000000000000, 0.000000000000000000, 1.000000000000000000 ) ) ;
#2538=CARTESIAN_POINT ( 'NONE',  ( 15.45522337368514521, -3.212533369474619427, 4.093511368021648167 ) ) ;
#2546=AXIS2_PLACEMENT_3D ( 'NONE', #9299, #21498, #9465 ) ;
#2552=ADVANCED_FACE ( 'NONE', ( #3795 ), #15832, .T. ) ;
#2553=CARTESIAN_POINT ( 'NONE',  ( 54.40000000000001990, 1.029992063861229212E-15, -4.375000000000002665 ) ) ;
#2554=CARTESIAN_POINT ( 'NONE',  ( 15.03925126672127810, -2.686240680702128625, -4.475885388010734545 ) ) ;
#2555=CARTESIAN_POINT ( 'NONE',  ( -35.85663232820584057, -3.275050215668598774, -2.949461045527609127 ) ) ;
#2556=DIRECTION ( 'NONE',  ( 0.000000000000000000, 0.000000000000000000, -1.000000000000000000 ) ) ;
#2567=B_SPLINE_CURVE_WITH_KNOTS ( 'NONE', 3,
 ( #27347, #29723, #29402, #5656, #8035, #12925, #19919, #14833, #21987, #280 ),
 .UNSPECIFIED., .F., .F.,
 ( 4, 2, 2, 2, 4 ),
 ( 0.000000000000000000, 0.0004363777631660865864, 0.0006545666447491310181, 0.0007636610855406569202, 0.0008727555263321828223 ),
 .UNSPECIFIED. ) ;
#2569=VERTEX_POINT ( 'NONE', #18379 ) ;
#2572=AXIS2_PLACEMENT_3D ( 'NONE', #7590, #12181, #16636 ) ;
#2579=CARTESIAN_POINT ( 'NONE',  ( -36.56390771145571961, 0.2088129849843024799, -5.405094643512487806 ) ) ;
#2581=CARTESIAN_POINT ( 'NONE',  ( 16.10660252424457184, -2.945786441214570672, 4.543674732827748031 ) ) ;
#2582=CARTESIAN_POINT ( 'NONE',  ( 54.49860577577695864, -0.002682860454195030130, -4.292318283074052054 ) ) ;
#2584=EDGE_CURVE ( 'NONE', #23640, #22807, #11115, .T. ) ;
#2587=CARTESIAN_POINT ( 'NONE',  ( -36.14504829323105639, -5.374753047227058822, -0.5963205376973962357 ) ) ;
#2588=VECTOR ( 'NONE', #13273, 1000.000000000000000 ) ;
#2589=DIRECTION ( 'NONE',  ( 1.000000000000000000, -1.165806029810706544E-15, -1.108125256279691767E-14 ) ) ;
#2596=ORIENTED_EDGE ( 'NONE', *, *, #14438, .T. ) ;
#2607=ORIENTED_EDGE ( 'NONE', *, *, #4355, .F. ) ;
#2610=CARTESIAN_POINT ( 'NONE',  ( -54.48118151432741030, -1.510613940323803694, 4.037256667234631280 ) ) ;
#2613=FACE_OUTER_BOUND ( 'NONE', #3696, .T. ) ;
#2615=FACE_OUTER_BOUND ( 'NONE', #17055, .T. ) ;
#2617=DIRECTION ( 'NONE',  ( 0.000000000000000000, 0.000000000000000000, -1.000000000000000000 ) ) ;
#2619=AXIS2_PLACEMENT_3D ( 'NONE', #12861, #1012, #24757 ) ;
#2623=CIRCLE ( 'NONE', #4124, 0.4576450603546982632 ) ;
#2624=VERTEX_POINT ( 'NONE', #1259 ) ;
#2625=CARTESIAN_POINT ( 'NONE',  ( 44.98443556292537693, -3.826179070414207573, 1.100000000000000311 ) ) ;
#2628=CARTESIAN_POINT ( 'NONE',  ( -35.85663232820601820, 2.199885893005899096, 4.939696249117697668 ) ) ;
#2634=EDGE_CURVE ( 'NONE', #24678, #14148, #6039, .T. ) ;
#2637=ORIENTED_EDGE ( 'NONE', *, *, #6688, .T. ) ;
#2646=CARTESIAN_POINT ( 'NONE',  ( 15.03925126672132961, -3.275050215668596998, 2.949461045527590475 ) ) ;
#2653=VECTOR ( 'NONE', #22802, 1000.000000000000000 ) ;
#2654=ORIENTED_EDGE ( 'NONE', *, *, #3672, .F. ) ;
#2658=DIRECTION ( 'NONE',  ( 0.000000000000000000, 1.000000000000000000, -0.000000000000000000 ) ) ;
#2659=VERTEX_POINT ( 'NONE', #26120 ) ;
#2660=DIRECTION ( 'NONE',  ( 0.000000000000000000, 1.000000000000000000, 0.000000000000000000 ) ) ;
#2661=APPLICATION_CONTEXT ( 'automotive_design' ) ;
#2662=VERTEX_POINT ( 'NONE', #26284 ) ;
#2663=CARTESIAN_POINT ( 'NONE',  ( 15.45522337368515409, 0.1928884786868352297, -5.200000000471178829 ) ) ;
#2664=CARTESIAN_POINT ( 'NONE',  ( -36.21152527658240672, -4.855742670514293202, 1.883114206442314309 ) ) ;
#2668=CARTESIAN_POINT ( 'NONE',  ( -35.85663232820584057, 3.426725943139577790, -3.937891353488711221 ) ) ;
#2669=DIRECTION ( 'NONE',  ( 0.000000000000000000, 1.000000000000000000, 0.000000000000000000 ) ) ;
#2678=DIRECTION ( 'NONE',  ( 0.000000000000000000, 1.000000000000000000, 0.000000000000000000 ) ) ;
#2679=AXIS2_PLACEMENT_3D ( 'NONE', #9089, #10829, #20512 ) ;
#2680=FACE_OUTER_BOUND ( 'NONE', #20214, .T. ) ;
#2681=EDGE_CURVE ( 'NONE', #16826, #29056, #7594, .T. ) ;
#2682=ORIENTED_EDGE ( 'NONE', *, *, #31061, .T. ) ;
#2684=CARTESIAN_POINT ( 'NONE',  ( 15.94709373951305409, -3.646691605040370820, 3.993181011920696299 ) ) ;
#2688=EDGE_CURVE ( 'NONE', #31086, #4137, #11081, .T. ) ;
#2691=CARTESIAN_POINT ( 'NONE',  ( -45.15971931043468146, -14.70000000000001883, 1.800230794746610701E-15 ) ) ;
#2692=VERTEX_POINT ( 'NONE', #28821 ) ;
#2694=ORIENTED_EDGE ( 'NONE', *, *, #17758, .F. ) ;
#2702=LINE ( 'NONE', #12342, #230 ) ;
#2705=CARTESIAN_POINT ( 'NONE',  ( 50.38154193469295450, 1.153441674035750708, 3.890342980189691158 ) ) ;
#2706=CARTESIAN_POINT ( 'NONE',  ( -36.56242893520637693, -5.206628483174487343, -1.466363261642641191 ) ) ;
#2709=EDGE_CURVE ( 'NONE', #9170, #21964, #16667, .T. ) ;
#2715=CARTESIAN_POINT ( 'NONE',  ( 58.45000000000001705, 0.8000000000000000444, 2.421260002560649660 ) ) ;
#2717=DIRECTION ( 'NONE',  ( -1.000000000000000000, -0.000000000000000000, -0.000000000000000000 ) ) ;
#2718=CARTESIAN_POINT ( 'NONE',  ( 51.80000000000001847, -4.227689052994008101, -1.125730994152045472 ) ) ;
#2719=DIRECTION ( 'NONE',  ( 1.000000000000000000, 0.000000000000000000, 0.000000000000000000 ) ) ;
#2723=CARTESIAN_POINT ( 'NONE',  ( 48.43966969621123297, 1.282137971188145320, -3.869545987293864897 ) ) ;
#2724=CARTESIAN_POINT ( 'NONE',  ( 15.03925126672132784, 4.683225679163376398, -2.703237727951165237 ) ) ;
#2727=ORIENTED_EDGE ( 'NONE', *, *, #25782, .T. ) ;
#2736=VERTEX_POINT ( 'NONE', #31190 ) ;
#2738=DIRECTION ( 'NONE',  ( -1.000000000000000000, -1.293068473084537258E-16, -0.000000000000000000 ) ) ;
#2747=CIRCLE ( 'NONE', #11346, 0.09999999999999982514 ) ;
#2750=CARTESIAN_POINT ( 'NONE',  ( 48.50000000000002132, -1.409787217987148233, 3.850000000000022737 ) ) ;
#2753=CARTESIAN_POINT ( 'NONE',  ( 51.80000000000001847, -4.131056160354152240, -1.100000000000000089 ) ) ;
#2755=CARTESIAN_POINT ( 'NONE',  ( -35.85663232820584057, 0.9159215771349650259, 4.311190327366005270 ) ) ;
#2756=CARTESIAN_POINT ( 'NONE',  ( 57.00000000000001421, 0.6999999999999999556, 2.452039967047845437 ) ) ;
#2757=CARTESIAN_POINT ( 'NONE',  ( 54.40000000000001990, 0.000000000000000000, 0.000000000000000000 ) ) ;
#2759=CARTESIAN_POINT ( 'NONE',  ( 51.87924854942583863, -4.254543194710165288, 1.020305229671191416 ) ) ;
#2771=AXIS2_PLACEMENT_3D ( 'NONE', #25710, #30445, #11460 ) ;
#2773=AXIS2_PLACEMENT_3D ( 'NONE', #24761, #539, #14935 ) ;
#2778=ORIENTED_EDGE ( 'NONE', *, *, #13678, .T. ) ;
#2791=CIRCLE ( 'NONE', #17473, 4.349999999999997868 ) ;
#2794=CARTESIAN_POINT ( 'NONE',  ( 57.05000000000001137, -0.7500000000000000000, -2.490438859776672231 ) ) ;
#2795=CARTESIAN_POINT ( 'NONE',  ( -36.22955757456082893, -3.272340825137205478, -4.050058705652198832 ) ) ;
#2805=CARTESIAN_POINT ( 'NONE',  ( 58.45000000000001705, 0.8000000000000000444, -2.421260002560649660 ) ) ;
#2806=EDGE_CURVE ( 'NONE', #23938, #13242, #2055, .T. ) ;
#2807=ORIENTED_EDGE ( 'NONE', *, *, #28988, .F. ) ;
#2812=FACE_OUTER_BOUND ( 'NONE', #24844, .T. ) ;
#2814=DIRECTION ( 'NONE',  ( 1.000000000000000000, 0.000000000000000000, 0.000000000000000000 ) ) ;
#2817=AXIS2_PLACEMENT_3D ( 'NONE', #301, #19643, #22172 ) ;
#2820=CARTESIAN_POINT ( 'NONE',  ( 50.30000000000001847, -4.899999999999999467, 3.950000000000022826 ) ) ;
#2821=EDGE_CURVE ( 'NONE', #20943, #1564, #27600, .T. ) ;
#2822=DIRECTION ( 'NONE',  ( 1.000000000000000000, -0.000000000000000000, -0.000000000000000000 ) ) ;
#2827=CARTESIAN_POINT ( 'NONE',  ( 15.48609859788819954, -3.148602930107186282, 4.139959549308917630 ) ) ;
#2829=CARTESIAN_POINT ( 'NONE',  ( 50.50000000000002132, -0.6304760106459029734, 3.950000000000022826 ) ) ;
#2831=CIRCLE ( 'NONE', #16498, 1.000000000000000000 ) ;
#2835=DIRECTION ( 'NONE',  ( 0.000000000000000000, 0.000000000000000000, -1.000000000000000000 ) ) ;
#2837=ORIENTED_EDGE ( 'NONE', *, *, #20652, .T. ) ;
#2838=DIRECTION ( 'NONE',  ( 0.000000000000000000, 0.000000000000000000, -1.000000000000000000 ) ) ;
#2843=CARTESIAN_POINT ( 'NONE',  ( 57.04458252721509126, 0.7500000000000000000, -2.421260002560649660 ) ) ;
#2844=CARTESIAN_POINT ( 'NONE',  ( 44.98443556292537693, -3.726179070414207928, -1.000000000000002220 ) ) ;
#2846=AXIS2_PLACEMENT_3D ( 'NONE', #15912, #30631, #6734 ) ;
#2852=AXIS2_PLACEMENT_3D ( 'NONE', #10632, #1125, #6191 ) ;
#2855=VECTOR ( 'NONE', #4319, 1000.000000000000000 ) ;
#2856=EDGE_CURVE ( 'NONE', #8076, #4056, #458, .T. ) ;
#2859=CARTESIAN_POINT ( 'NONE',  ( -36.63359589171323449, -5.330414537250521612, -0.9106291984479789603 ) ) ;
#2860=ORIENTED_EDGE ( 'NONE', *, *, #14964, .F. ) ;
#2862=FACE_OUTER_BOUND ( 'NONE', #8637, .T. ) ;
#2867=AXIS2_PLACEMENT_3D ( 'NONE', #30258, #21098, #8709 ) ;
#2869=VECTOR ( 'NONE', #28675, 1000.000000000000000 ) ;
#2871=CARTESIAN_POINT ( 'NONE',  ( 48.43940831342823117, -1.279117291415095448, -3.870058441400159754 ) ) ;
#2872=CARTESIAN_POINT ( 'NONE',  ( 51.90000000000001279, 1.734723475976807094E-15, 0.000000000000000000 ) ) ;
#2879=CIRCLE ( 'NONE', #26641, 0.04999999999999969746 ) ;
#2881=CARTESIAN_POINT ( 'NONE',  ( 54.48476976571165409, -0.001523517289327013143, -4.328047699026194017 ) ) ;
#2883=DIRECTION ( 'NONE',  ( -1.000000000000000000, -0.000000000000000000, -0.000000000000000000 ) ) ;
#2884=CARTESIAN_POINT ( 'NONE',  ( -35.85663232820583346, -5.377732432866659806, -0.5657657256215629094 ) ) ;
#2886=CARTESIAN_POINT ( 'NONE',  ( 16.07512358269928399, 2.917650619476306328, -4.554978966839664523 ) ) ;
#2890=ORIENTED_EDGE ( 'NONE', *, *, #2709, .F. ) ;
#2893=ADVANCED_FACE ( 'NONE', ( #10846 ), #8019, .T. ) ;
#2895=ORIENTED_EDGE ( 'NONE', *, *, #11678, .F. ) ;
#2897=CARTESIAN_POINT ( 'NONE',  ( 15.18463186935387910, -5.377732432866779710, 0.5657657256210123498 ) ) ;
#2900=CARTESIAN_POINT ( 'NONE',  ( 15.03925126672132784, 4.683225679163368405, -2.703237727951182112 ) ) ;
#2908=AXIS2_PLACEMENT_3D ( 'NONE', #15482, #4479, #26174 ) ;
#2913=CARTESIAN_POINT ( 'NONE',  ( 51.78359321857947606, -4.158733306197476942, -1.045116725612200259 ) ) ;
#2918=DIRECTION ( 'NONE',  ( 1.000000000000000000, -0.000000000000000000, -0.000000000000000000 ) ) ;
#2919=CARTESIAN_POINT ( 'NONE',  ( 57.02528775048638465, 0.7434661330690420789, 2.425538622349843632 ) ) ;
#2921=CIRCLE ( 'NONE', #6978, 1.899999999999999911 ) ;
#2925=DIRECTION ( 'NONE',  ( 1.000000000000000000, 0.000000000000000000, 0.000000000000000000 ) ) ;
#2941=CIRCLE ( 'NONE', #21682, 4.100000000000022737 ) ;
#2944=EDGE_LOOP ( 'NONE', ( #6028, #13857, #28987 ) ) ;
#2946=EDGE_LOOP ( 'NONE', ( #26559, #27622, #13768, #9867, #4918 ) ) ;
#2950=CARTESIAN_POINT ( 'NONE',  ( 15.44631504820156387, -5.012449653004652284, -1.400819699606176583 ) ) ;
#2958=CIRCLE ( 'NONE', #10540, 0.4576450603546999840 ) ;
#2959=CARTESIAN_POINT ( 'NONE',  ( 51.80000000000001847, 1.029992063861229212E-15, -4.375000000000002665 ) ) ;
#2972=DIRECTION ( 'NONE',  ( -1.000000000000000000, 0.000000000000000000, 0.000000000000000000 ) ) ;
#2985=CARTESIAN_POINT ( 'NONE',  ( 57.03612573316699041, -0.7785448249619018046, 1.733167030474859205 ) ) ;
#2986=CARTESIAN_POINT ( 'NONE',  ( 16.10667815269232861, -3.062358472872038107, -4.459001320275592484 ) ) ;
#2992=CARTESIAN_POINT ( 'NONE',  ( 47.00000000000002132, -3.726179070414207928, 1.710435481158852244 ) ) ;
#2994=CARTESIAN_POINT ( 'NONE',  ( 15.87128154250933321, -2.562020839648921910, 4.763023844700866150 ) ) ;
#2998=CARTESIAN_POINT ( 'NONE',  ( -35.85663232820582635, 4.804073783693455724, -2.042134687550313910 ) ) ;
#3001=ORIENTED_EDGE ( 'NONE', *, *, #8441, .F. ) ;
#3002=CONICAL_SURFACE ( 'NONE', #10584, 4.375000000000000000, 0.06758856876739828545 ) ;
#3004=DIRECTION ( 'NONE',  ( 1.000000000000000000, 0.000000000000000000, -0.000000000000000000 ) ) ;
#3008=CYLINDRICAL_SURFACE ( 'NONE', #6532, 0.9999999999999995559 ) ;
#3009=EDGE_CURVE ( 'NONE', #5897, #24423, #18693, .T. ) ;
#3010=ORIENTED_EDGE ( 'NONE', *, *, #20548, .T. ) ;
#3011=ORIENTED_EDGE ( 'NONE', *, *, #943, .T. ) ;
#3018=CARTESIAN_POINT ( 'NONE',  ( -36.31440869660544024, -4.928592478219097295, -1.658905555082604621 ) ) ;
#3021=VERTEX_POINT ( 'NONE', #13687 ) ;
#3022=AXIS2_PLACEMENT_3D ( 'NONE', #18836, #9497, #13885 ) ;
#3027=CARTESIAN_POINT ( 'NONE',  ( 15.29954477411524039, -1.123735554575206574, 5.289358692618363555 ) ) ;
#3028=EDGE_CURVE ( 'NONE', #28557, #11230, #27764, .T. ) ;
#3029=CARTESIAN_POINT ( 'NONE',  ( 51.73129885173067066, -4.259946762565045120, -1.000000153509809531 ) ) ;
#3036=CARTESIAN_POINT ( 'NONE',  ( 54.47883572522132312, -0.001215825626373222409, -4.337530305537235620 ) ) ;
#3040=AXIS2_PLACEMENT_3D ( 'NONE', #29692, #20375, #13211 ) ;
#3043=CARTESIAN_POINT ( 'NONE',  ( -36.89831264271881395, -5.226279933021941382, -1.394410282272816382 ) ) ;
#3044=CARTESIAN_POINT ( 'NONE',  ( 15.61552784268241822, 2.776541361170906885, -4.646985486732077675 ) ) ;
#3047=EDGE_CURVE ( 'NONE', #21976, #3728, #25735, .T. ) ;
#3052=CARTESIAN_POINT ( 'NONE',  ( 15.03925126672133139, -5.377732432866647372, 0.5657657256215454789 ) ) ;
#3055=CARTESIAN_POINT ( 'NONE',  ( 16.00221665700882312, 4.939398376933317181, -2.210903708596424710 ) ) ;
#3056=EDGE_LOOP ( 'NONE', ( #24773, #10858, #16742, #13020 ) ) ;
#3060=ORIENTED_EDGE ( 'NONE', *, *, #4821, .T. ) ;
#3061=CARTESIAN_POINT ( 'NONE',  ( 54.48476976571165409, -0.001523517289377870247, 4.328047699026194017 ) ) ;
#3062=DIRECTION ( 'NONE',  ( 0.000000000000000000, -1.000000000000000000, 0.000000000000000000 ) ) ;
#3065=CARTESIAN_POINT ( 'NONE',  ( 51.75285304771053774, -4.172892586174061336, -1.014428651009326554 ) ) ;
#3069=EDGE_CURVE ( 'NONE', #25469, #1935, #2831, .T. ) ;
#3072=CARTESIAN_POINT ( 'NONE',  ( -36.22909104983144601, -3.722832355337217791, 3.938244298533509991 ) ) ;
#3076=DIRECTION ( 'NONE',  ( 0.000000000000000000, 0.000000000000000000, -1.000000000000000000 ) ) ;
#3081=ORIENTED_EDGE ( 'NONE', *, *, #1365, .F. ) ;
#3082=VERTEX_POINT ( 'NONE', #21327 ) ;
#3087=ORIENTED_EDGE ( 'NONE', *, *, #20145, .T. ) ;
#3092=ORIENTED_EDGE ( 'NONE', *, *, #18636, .F. ) ;
#3095=DIRECTION ( 'NONE',  ( -0.000000000000000000, 1.000000000000000000, 1.224646799147353207E-16 ) ) ;
#3097=CARTESIAN_POINT ( 'NONE',  ( 15.74504787372189085, -5.074157625981885467, -1.874066637979881822 ) ) ;
#3106=FACE_OUTER_BOUND ( 'NONE', #3671, .T. ) ;
#3108=CARTESIAN_POINT ( 'NONE',  ( 57.00000000000001421, -0.7500000000000000000, 3.499999999999999556 ) ) ;
#3110=CARTESIAN_POINT ( 'NONE',  ( -35.85663232820584057, 3.056483311920880297, -4.206888370749704897 ) ) ;
#3111=EDGE_LOOP ( 'NONE', ( #5349, #1535, #31123, #17405 ) ) ;
#3114=CARTESIAN_POINT ( 'NONE',  ( -36.92443669619772351, -3.051830235923030266, -4.466755975380271693 ) ) ;
#3116=EDGE_LOOP ( 'NONE', ( #8128, #12278, #22121, #22936 ) ) ;
#3118=FACE_OUTER_BOUND ( 'NONE', #13555, .T. ) ;
#3125=VERTEX_POINT ( 'NONE', #18106 ) ;
#3127=B_SPLINE_CURVE_WITH_KNOTS ( 'NONE', 3,
 ( #6196, #5725, #15547, #20465, #20315, #1129, #18246, #25025, #29945, #8411, #25352, #10782, #25200, #15844, #25496, #3808 ),
 .UNSPECIFIED., .F., .F.,
 ( 4, 2, 2, 2, 2, 2, 2, 4 ),
 ( 0.000000000000000000, 0.0004351083927046398795, 0.0008702167854092797590, 0.001740433570818559518, 0.002175541963523200048, 0.002610650356227840578, 0.003045758748932481542, 0.003480867141637122072 ),
 .UNSPECIFIED. ) ;
#3130=AXIS2_PLACEMENT_3D ( 'NONE', #13486, #23470, #9230 ) ;
#3133=CARTESIAN_POINT ( 'NONE',  ( -54.45487361440510909, -1.499999999999999556, -4.029888335921975262 ) ) ;
#3138=CIRCLE ( 'NONE', #8681, 1.000000000000000000 ) ;
#3139=AXIS2_PLACEMENT_3D ( 'NONE', #20012, #12399, #7980 ) ;
#3141=CARTESIAN_POINT ( 'NONE',  ( 57.00000000000001421, -0.6999999999999999556, -1.820027472320129736 ) ) ;
#3144=ORIENTED_EDGE ( 'NONE', *, *, #9670, .T. ) ;
#3147=CARTESIAN_POINT ( 'NONE',  ( 15.44631504820161716, 3.231775792180334061, 4.079530926931304258 ) ) ;
#3149=CARTESIAN_POINT ( 'NONE',  ( 51.70000000000001705, -0.1421112804877788793, -1.100000000000000089 ) ) ;
#3156=PRODUCT_DEFINITION_CONTEXT ( 'detailed design', #26971, 'design' ) ;
#3160=ORIENTED_EDGE ( 'NONE', *, *, #20049, .T. ) ;
#3161=ORIENTED_EDGE ( 'NONE', *, *, #3819, .F. ) ;
#3162=CARTESIAN_POINT ( 'NONE',  ( 58.45000000000001705, 0.7500000000000000000, -2.421260002560649660 ) ) ;
#3163=DIRECTION ( 'NONE',  ( -1.000000000000000000, 0.000000000000000000, 0.000000000000000000 ) ) ;
#3166=CARTESIAN_POINT ( 'NONE',  ( 51.80000000000001847, -4.137078223593629644, 1.088692053889325217 ) ) ;
#3168=AXIS2_PLACEMENT_3D ( 'NONE', #2141, #16570, #18944 ) ;
#3169=CARTESIAN_POINT ( 'NONE',  ( 51.80000000000001847, -3.726179070414207928, -1.710435481158852467 ) ) ;
#3173=ORIENTED_EDGE ( 'NONE', *, *, #13867, .T. ) ;
#3176=CARTESIAN_POINT ( 'NONE',  ( -39.16187796471576377, -1.705048840508494473E-14, 0.000000000000000000 ) ) ;
#3179=ADVANCED_FACE ( 'NONE', ( #15717 ), #6358, .T. ) ;
#3180=CARTESIAN_POINT ( 'NONE',  ( 51.89999993196679640, -4.241636233590472926, -1.073352279313352087 ) ) ;
#3185=DIRECTION ( 'NONE',  ( 0.000000000000000000, -0.9663289263986323263, -0.2573099415204678220 ) ) ;
#3186=CARTESIAN_POINT ( 'NONE',  ( 15.32752150720753725, -2.228039998204434102, 4.927410888447834481 ) ) ;
#3189=EDGE_LOOP ( 'NONE', ( #5675, #9137, #1698, #24754 ) ) ;
#3191=DIRECTION ( 'NONE',  ( 1.000000000000000000, 0.000000000000000000, 0.000000000000000000 ) ) ;
#3192=CARTESIAN_POINT ( 'NONE',  ( 15.95705409078441583, 2.672993279333413241, -4.702725322014949860 ) ) ;
#3195=ORIENTED_EDGE ( 'NONE', *, *, #11695, .F. ) ;
#3198=VERTEX_POINT ( 'NONE', #8266 ) ;
#3199=DIRECTION ( 'NONE',  ( 0.000000000000000000, 1.000000000000000000, 0.000000000000000000 ) ) ;
#3200=ORIENTED_EDGE ( 'NONE', *, *, #23820, .F. ) ;
#3203=CARTESIAN_POINT ( 'NONE',  ( 15.59140265158955430, 5.360483378448146041, -0.7132926830812214014 ) ) ;
#3204=EDGE_LOOP ( 'NONE', ( #12274, #24194, #26446, #18263, #22081 ) ) ;
#3209=CARTESIAN_POINT ( 'NONE',  ( 54.49932581792542408, -0.002837702349018913269, 4.287546236934917765 ) ) ;
#3212=DIRECTION ( 'NONE',  ( 0.000000000000000000, -1.000000000000000000, 0.000000000000000000 ) ) ;
#3221=DIRECTION ( 'NONE',  ( -1.000000000000000000, 0.000000000000000000, 0.000000000000000000 ) ) ;
#3222=CARTESIAN_POINT ( 'NONE',  ( 56.97542489291938494, -0.7477441023849552559, -1.746698826563745977 ) ) ;
#3226=DIRECTION ( 'NONE',  ( 2.459562394685749209E-16, -0.9510565162951544194, 0.3090169943749447312 ) ) ;
#3229=CARTESIAN_POINT ( 'NONE',  ( 33.47623932017462778, 1.734723475976807094E-15, 0.000000000000000000 ) ) ;
#3231=CARTESIAN_POINT ( 'NONE',  ( 48.30000000000001847, -0.6462379109120514054, 4.048750000000023164 ) ) ;
#3241=ORIENTED_EDGE ( 'NONE', *, *, #8062, .F. ) ;
#3242=ADVANCED_FACE ( 'NONE', ( #832 ), #825, .T. ) ;
#3243=ORIENTED_EDGE ( 'NONE', *, *, #24868, .F. ) ;
#3246=ORIENTED_EDGE ( 'NONE', *, *, #22066, .T. ) ;
#3254=CARTESIAN_POINT ( 'NONE',  ( 15.68751737981906125, -5.024465639091984848, -2.007392901578175515 ) ) ;
#3267=CARTESIAN_POINT ( 'NONE',  ( -36.14504829323105639, 1.093755498983955521, 5.295967089285810836 ) ) ;
#3268=ORIENTED_EDGE ( 'NONE', *, *, #2681, .T. ) ;
#3273=VERTEX_POINT ( 'NONE', #11421 ) ;
#3275=ORIENTED_EDGE ( 'NONE', *, *, #27382, .F. ) ;
#3282=EDGE_CURVE ( 'NONE', #29056, #11687, #30129, .T. ) ;
#3292=ORIENTED_EDGE ( 'NONE', *, *, #2244, .T. ) ;
#3300=ORIENTED_EDGE ( 'NONE', *, *, #17085, .T. ) ;
#3301=CARTESIAN_POINT ( 'NONE',  ( 15.03925126672132961, -2.686240680702166816, 4.475885388010711452 ) ) ;
#3307=CARTESIAN_POINT ( 'NONE',  ( -36.22818246778668794, 0.6967302926296138343, 5.374298406428920316 ) ) ;
#3309=ORIENTED_EDGE ( 'NONE', *, *, #7693, .F. ) ;
#3310=FACE_OUTER_BOUND ( 'NONE', #19501, .T. ) ;
#3313=CARTESIAN_POINT ( 'NONE',  ( 15.41586008885044734, -3.272294129011796837, -4.050092634494051325 ) ) ;
#3315=AXIS2_PLACEMENT_3D ( 'NONE', #5512, #20406, #10110 ) ;
#3327=AXIS2_PLACEMENT_3D ( 'NONE', #8358, #1086, #13252 ) ;
#3328=CARTESIAN_POINT ( 'NONE',  ( -35.98994760229851408, -4.804073784580272566, -2.042134692980068333 ) ) ;
#3339=CARTESIAN_POINT ( 'NONE',  ( 48.48122134030800368, -1.391940262981015586, -3.850000000000022293 ) ) ;
#3340=CARTESIAN_POINT ( 'NONE',  ( 15.61033468494287746, -0.4841707035674406301, 5.391286593723129350 ) ) ;
#3345=CARTESIAN_POINT ( 'NONE',  ( -35.85663232820584057, 5.086913985776147840, -1.171642053949061513 ) ) ;
#3347=AXIS2_PLACEMENT_3D ( 'NONE', #20804, #18424, #27765 ) ;
#3350=CIRCLE ( 'NONE', #20045, 1.000000000000000000 ) ;
#3354=CARTESIAN_POINT ( 'NONE',  ( 47.00000000000002132, -3.826179070414207573, 1.000000000000000222 ) ) ;
#3356=DIRECTION ( 'NONE',  ( -1.000000000000000000, 0.000000000000000000, 0.000000000000000000 ) ) ;
#3357=CARTESIAN_POINT ( 'NONE',  ( 16.10705563471230306, 3.051830235923028933, -4.466755975380259258 ) ) ;
#3358=CARTESIAN_POINT ( 'NONE',  ( 57.05000000000001137, 0.7500000000000000000, 2.421260002560653213 ) ) ;
#3363=EDGE_LOOP ( 'NONE', ( #2146, #10642, #5548, #30651 ) ) ;
#3365=CARTESIAN_POINT ( 'NONE',  ( 15.59055531549693896, -4.755763096844272120, 2.574151833883791873 ) ) ;
#3366=EDGE_CURVE ( 'NONE', #10988, #5143, #15953, .T. ) ;
#3368=AXIS2_PLACEMENT_3D ( 'NONE', #2691, #14860, #9679 ) ;
#3369=CARTESIAN_POINT ( 'NONE',  ( 16.00221665700882667, 2.696520634775366076, -4.691964194339891314 ) ) ;
#3370=DIRECTION ( 'NONE',  ( 0.000000000000000000, 0.000000000000000000, 1.000000000000000000 ) ) ;
#3371=ORIENTED_EDGE ( 'NONE', *, *, #24152, .T. ) ;
#3373=DIRECTION ( 'NONE',  ( 1.000000000000000000, 9.742518634817235071E-17, 4.338815227941366087E-17 ) ) ;
#3376=CIRCLE ( 'NONE', #16531, 1.000000000000000000 ) ;
#3377=CARTESIAN_POINT ( 'NONE',  ( 56.98303665332567647, 0.7553445069156616842, -1.743428900644034885 ) ) ;
#3389=CARTESIAN_POINT ( 'NONE',  ( 57.00059118976931671, -0.7088470050679284151, 2.446935707828179485 ) ) ;
#3393=ADVANCED_FACE ( 'NONE', ( #2025 ), #30995, .T. ) ;
#3395=CARTESIAN_POINT ( 'NONE',  ( 50.46999119548826940, -1.140870969100513888, -3.938727831757874664 ) ) ;
#3400=CARTESIAN_POINT ( 'NONE',  ( 51.90000000000001279, -1.084202172485504434E-16, 4.374999999999999112 ) ) ;
#3402=B_SPLINE_CURVE_WITH_KNOTS ( 'NONE', 3,
 ( #976, #29934, #8243, #17908, #2207, #13912, #2059, #14088, #20913, #28348, #11721, #19185, #16316, #18858, #13754, #23608 ),
 .UNSPECIFIED., .F., .F.,
 ( 4, 3, 3, 3, 3, 4 ),
 ( 0.000000000000000000, 8.780272313934440255E-06, 2.643179650512019594E-05, 4.557815634108688274E-05, 6.564640436636450416E-05, 8.596378008536510913E-05 ),
 .UNSPECIFIED. ) ;
#3404=CIRCLE ( 'NONE', #21120, 0.05000000000000012768 ) ;
#3406=VECTOR ( 'NONE', #5662, 1000.000000000000000 ) ;
#3407=EDGE_CURVE ( 'NONE', #17261, #15970, #6471, .T. ) ;
#3414=CARTESIAN_POINT ( 'NONE',  ( 51.80000000000001847, -4.131056160354152240, 1.099999999999999867 ) ) ;
#3423=CARTESIAN_POINT ( 'NONE',  ( 34.50000000000001421, 0.000000000000000000, 0.000000000000000000 ) ) ;
#3425=CIRCLE ( 'NONE', #28180, 1.000000000000000000 ) ;
#3434=CARTESIAN_POINT ( 'NONE',  ( 47.00000000000002132, -3.726179070414207928, 1.100000000000000311 ) ) ;
#3437=CARTESIAN_POINT ( 'NONE',  ( 58.45000000000001705, -0.8000000000000000444, 2.421260002560649660 ) ) ;
#3438=CARTESIAN_POINT ( 'NONE',  ( -35.85663232820584057, 1.123735532908288315, 5.289358697221541838 ) ) ;
#3444=VERTEX_POINT ( 'NONE', #25614 ) ;
#3448=EDGE_LOOP ( 'NONE', ( #24740, #30646, #21922, #14424 ) ) ;
#3454=DIRECTION ( 'NONE',  ( -0.000000000000000000, 0.9875000000000001554, -0.1576190026614806561 ) ) ;
#3457=CARTESIAN_POINT ( 'NONE',  ( 57.00000000000001421, -0.6999999999999999556, -1.820027472320129736 ) ) ;
#3458=VERTEX_POINT ( 'NONE', #1545 ) ;
#3460=DIRECTION ( 'NONE',  ( 0.000000000000000000, 0.000000000000000000, 1.000000000000000000 ) ) ;
#3461=CYLINDRICAL_SURFACE ( 'NONE', #23554, 0.1000000000000000472 ) ;
#3467=CIRCLE ( 'NONE', #25191, 0.1000000000000000472 ) ;
#3472=DIRECTION ( 'NONE',  ( 0.000000000000000000, 0.000000000000000000, -1.000000000000000000 ) ) ;
#3473=EDGE_CURVE ( 'NONE', #9481, #8076, #3850, .T. ) ;
#3477=ORIENTED_EDGE ( 'NONE', *, *, #7992, .F. ) ;
#3484=ORIENTED_EDGE ( 'NONE', *, *, #14885, .T. ) ;
#3485=ORIENTED_EDGE ( 'NONE', *, *, #29057, .T. ) ;
#3488=CIRCLE ( 'NONE', #9586, 3.675000000000029132 ) ;
#3490=VERTEX_POINT ( 'NONE', #11208 ) ;
#3495=CARTESIAN_POINT ( 'NONE',  ( 51.90000000000001279, -4.227689052994015206, 1.125730994152046582 ) ) ;
#3498=ORIENTED_EDGE ( 'NONE', *, *, #15692, .T. ) ;
#3502=CARTESIAN_POINT ( 'NONE',  ( 15.67083574136752233, 0.3995010896672199774, 5.397102918580290343 ) ) ;
#3503=EDGE_CURVE ( 'NONE', #26503, #9408, #20882, .T. ) ;
#3510=DIRECTION ( 'NONE',  ( 0.000000000000000000, 0.000000000000000000, 1.000000000000000000 ) ) ;
#3514=ORIENTED_EDGE ( 'NONE', *, *, #2244, .F. ) ;
#3515=CARTESIAN_POINT ( 'NONE',  ( 50.40741710815419196, -1.342093792059618762, -3.874237195466570416 ) ) ;
#3516=CARTESIAN_POINT ( 'NONE',  ( 36.50000000000002132, 0.000000000000000000, 0.000000000000000000 ) ) ;
#3519=CARTESIAN_POINT ( 'NONE',  ( -54.44999999999997442, -1.500000000000000222, -3.300094695611020867 ) ) ;
#3528=EDGE_LOOP ( 'NONE', ( #415, #8028, #2607, #19594 ) ) ;
#3529=B_SPLINE_CURVE_WITH_KNOTS ( 'NONE', 3,
 ( #28835, #26448, #17738, #27523, #15192, #1240, #5689, #15339, #25463, #29755 ),
 .UNSPECIFIED., .F., .F.,
 ( 4, 2, 2, 2, 4 ),
 ( 0.000000000000000000, 0.0004363777631660871827, 0.0006545666447491323191, 0.0007636610855406580044, 0.0008727555263321836896 ),
 .UNSPECIFIED. ) ;
#3532=VERTEX_POINT ( 'NONE', #19444 ) ;
#3534=CIRCLE ( 'NONE', #29310, 0.09999999999999986677 ) ;
#3536=VECTOR ( 'NONE', #28101, 1000.000000000000000 ) ;
#3538=DIRECTION ( 'NONE',  ( -1.000000000000000000, -0.000000000000000000, -0.000000000000000000 ) ) ;
#3544=PLANE ( 'NONE',  #8895 ) ;
#3555=VERTEX_POINT ( 'NONE', #9779 ) ;
#3556=CARTESIAN_POINT ( 'NONE',  ( 50.46953806735880477, -1.143620537822792826, 3.937943076466138059 ) ) ;
#3557=CARTESIAN_POINT ( 'NONE',  ( -36.81959771849335539, 0.5763363385013660078, -5.380853831843024793 ) ) ;
#3558=TOROIDAL_SURFACE ( 'NONE', #21783, 1.850000000000000089, 0.05000000000000000278 ) ;
#3559=ORIENTED_EDGE ( 'NONE', *, *, #15795, .T. ) ;
#3567=VERTEX_POINT ( 'NONE', #26866 ) ;
#3572=VERTEX_POINT ( 'NONE', #6946 ) ;
#3576=DIRECTION ( 'NONE',  ( -1.000000000000000000, -2.586136946169074517E-16, 0.000000000000000000 ) ) ;
#3587=FACE_OUTER_BOUND ( 'NONE', #26256, .T. ) ;
#3588=EDGE_LOOP ( 'NONE', ( #25622, #30153, #8301, #3200 ) ) ;
#3590=ORIENTED_EDGE ( 'NONE', *, *, #9432, .T. ) ;
#3600=CARTESIAN_POINT ( 'NONE',  ( 57.04540039768303217, -0.7500000000000000000, -1.778341924377873751 ) ) ;
#3602=FACE_OUTER_BOUND ( 'NONE', #13881, .T. ) ;
#3603=SPHERICAL_SURFACE ( 'NONE', #30210, 0.05000000000000000278 ) ;
#3609=CARTESIAN_POINT ( 'NONE',  ( -36.40793637698146057, -3.917775493694432676, 3.727542820438226379 ) ) ;
#3610=DIRECTION ( 'NONE',  ( 1.000000000000000000, -1.805490781531896312E-17, 1.716160222047132579E-16 ) ) ;
#3616=CARTESIAN_POINT ( 'NONE',  ( 16.07512358269928399, 3.430438802933705400, 4.182416543699213562 ) ) ;
#3618=ADVANCED_FACE ( 'NONE', ( #26554 ), #5059, .T. ) ;
#3619=DIRECTION ( 'NONE',  ( 0.000000000000000000, 1.000000000000000000, 0.000000000000000000 ) ) ;
#3623=CARTESIAN_POINT ( 'NONE',  ( 48.50000000000354561, 1.426739617988885822, -3.843749999997122746 ) ) ;
#3625=AXIS2_PLACEMENT_3D ( 'NONE', #24149, #3221, #27759 ) ;
#3626=DIRECTION ( 'NONE',  ( 0.000000000000000000, -1.000000000000000000, 0.000000000000000000 ) ) ;
#3627=VERTEX_POINT ( 'NONE', #2340 ) ;
#3632=CARTESIAN_POINT ( 'NONE',  ( 47.00000000000002132, 2.264383216608037083E-15, -4.275000000000000355 ) ) ;
#3653=CARTESIAN_POINT ( 'NONE',  ( -35.85663232820584767, 3.817150320980521983, -2.203324261490877678 ) ) ;
#3655=EDGE_LOOP ( 'NONE', ( #7297, #5658, #2596, #6910 ) ) ;
#3656=CARTESIAN_POINT ( 'NONE',  ( 50.37844020491943553, -1.181909706220196643, -3.885998080850099790 ) ) ;
#3657=( BOUNDED_SURFACE ( )  B_SPLINE_SURFACE ( 3, 2, ( 
 ( #14406, #26451, #31038 ),
 ( #9360, #28513, #11735 ),
 ( #18870, #9537, #30736 ),
 ( #6816, #16481, #21731 ),
 ( #28683, #9043, #16327 ),
 ( #21262, #28836, #18717 ),
 ( #26140, #16810, #19197 ),
 ( #4278, #6997, #28360 ),
 ( #12055, #11884, #4128 ),
 ( #4449, #11408, #16659 ),
 ( #19025, #26300, #6665 ),
 ( #28980, #14099, #21099 ),
 ( #4601, #14258, #23928 ),
 ( #7147, #9209, #24078 ),
 ( #1738, #2392, #22 ),
 ( #25820, #9684, #30893 ) ),
 .UNSPECIFIED., .F., .F., .T. ) 
 B_SPLINE_SURFACE_WITH_KNOTS ( ( 4, 2, 2, 2, 2, 2, 2, 4 ),
 ( 3, 3 ),
 ( 0.001780502285214233737, 0.002558945925323762895, 0.002753556835351145347, 0.002948167745378527799, 0.003337389565433292269, 0.003726611385488056739, 0.004115833205542821643, 0.004894276845652350584 ),
 ( 0.000000000000000000, 1.000000000000000000 ),
 .UNSPECIFIED. ) 
 GEOMETRIC_REPRESENTATION_ITEM ( )  RATIONAL_B_SPLINE_SURFACE ( (
 ( 1.000000000000000000, 0.9418517008537257151, 1.000000000000000000),
 ( 1.000000000000000000, 0.9417987965884543344, 1.000000000000000000),
 ( 1.000000000000000000, 0.9418198861734828897, 1.000000000000000000),
 ( 1.000000000000000000, 0.9434060303845416273, 1.000000000000000000),
 ( 1.000000000000000000, 0.9437939819948035769, 1.000000000000000000),
 ( 1.000000000000000000, 0.9445989566712962304, 1.000000000000000000),
 ( 1.000000000000000000, 0.9450169930049948652, 1.000000000000000000),
 ( 1.000000000000000000, 0.9461610507673405834, 1.000000000000000000),
 ( 1.000000000000000000, 0.9467217966426996201, 1.000000000000000000),
 ( 1.000000000000000000, 0.9467345476124578996, 1.000000000000000000),
 ( 1.000000000000000000, 0.9461964028052806119, 1.000000000000000000),
 ( 1.000000000000000000, 0.9446801822474001353, 1.000000000000000000),
 ( 1.000000000000000000, 0.9437582546536619210, 1.000000000000000000),
 ( 1.000000000000000000, 0.9418129560295545044, 1.000000000000000000),
 ( 1.000000000000000000, 0.9418016889777601763, 1.000000000000000000),
 ( 1.000000000000000000, 0.9418517008537246049, 1.000000000000000000) ) ) 
 REPRESENTATION_ITEM ( '' )  SURFACE ( )  );
#3658=DIRECTION ( 'NONE',  ( 0.000000000000000000, 0.000000000000000000, -1.000000000000000000 ) ) ;
#3669=LINE ( 'NONE', #20478, #23016 ) ;
#3671=EDGE_LOOP ( 'NONE', ( #25294, #8373, #6957, #3275 ) ) ;
#3672=EDGE_CURVE ( 'NONE', #1297, #13242, #18947, .T. ) ;
#3696=EDGE_LOOP ( 'NONE', ( #5415, #9753, #3060, #1213, #6279, #28375 ) ) ;
#3697=LINE ( 'NONE', #25864, #15408 ) ;
#3701=CARTESIAN_POINT ( 'NONE',  ( 51.75857864376271067, -3.767600426651517509, -1.000000000000000000 ) ) ;
#3706=ORIENTED_EDGE ( 'NONE', *, *, #27001, .T. ) ;
#3707=EDGE_CURVE ( 'NONE', #2009, #10802, #17415, .T. ) ;
#3709=ORIENTED_EDGE ( 'NONE', *, *, #4981, .F. ) ;
#3714=CARTESIAN_POINT ( 'NONE',  ( 51.80000000000001847, 1.521694824349937303, 3.995005614707771269 ) ) ;
#3728=VERTEX_POINT ( 'NONE', #25534 ) ;
#3736=CARTESIAN_POINT ( 'NONE',  ( -54.49999999999997868, -1.550000000000000044, 3.332135201338624508 ) ) ;
#3741=CARTESIAN_POINT ( 'NONE',  ( 57.04073536323585358, -0.7493370604887438224, -1.778939771162194372 ) ) ;
#3743=CYLINDRICAL_SURFACE ( 'NONE', #21161, 0.09999999999999982514 ) ;
#3745=DIRECTION ( 'NONE',  ( 1.000000000000000000, 0.000000000000000000, 0.000000000000000000 ) ) ;
#3747=AXIS2_PLACEMENT_3D ( 'NONE', #6171, #15818, #20750 ) ;
#3748=CARTESIAN_POINT ( 'NONE',  ( -36.11187263677958015, 5.068523420888933373, -1.228242390833621300 ) ) ;
#3764=LINE ( 'NONE', #8670, #25720 ) ;
#3770=CARTESIAN_POINT ( 'NONE',  ( 48.40000000000002700, 0.6462379109121008103, 4.048750000000028493 ) ) ;
#3776=DIRECTION ( 'NONE',  ( 0.000000000000000000, 0.000000000000000000, 1.000000000000000000 ) ) ;
#3778=DIRECTION ( 'NONE',  ( 1.000000000000000000, 0.000000000000000000, 0.000000000000000000 ) ) ;
#3784=CIRCLE ( 'NONE', #16427, 3.200000000000000178 ) ;
#3785=DIRECTION ( 'NONE',  ( 1.000000000000000000, 0.000000000000000000, 0.000000000000000000 ) ) ;
#3795=FACE_OUTER_BOUND ( 'NONE', #16966, .T. ) ;
#3799=EDGE_CURVE ( 'NONE', #3728, #14710, #26024, .T. ) ;
#3805=ORIENTED_EDGE ( 'NONE', *, *, #29545, .T. ) ;
#3808=CARTESIAN_POINT ( 'NONE',  ( -35.85663232820584057, 2.199885893005988358, -4.939696249117657700 ) ) ;
#3809=DIRECTION ( 'NONE',  ( 0.000000000000000000, 0.000000000000000000, 1.000000000000000000 ) ) ;
#3813=ORIENTED_EDGE ( 'NONE', *, *, #14851, .T. ) ;
#3818=AXIS2_PLACEMENT_3D ( 'NONE', #8982, #24017, #28305 ) ;
#3819=EDGE_CURVE ( 'NONE', #22708, #13977, #21974, .T. ) ;
#3823=CARTESIAN_POINT ( 'NONE',  ( 15.18459684427939749, 2.199885893006011006, -4.939696249117653259 ) ) ;
#3825=ORIENTED_EDGE ( 'NONE', *, *, #16917, .F. ) ;
#3830=VECTOR ( 'NONE', #23103, 1000.000000000000000 ) ;
#3838=CARTESIAN_POINT ( 'NONE',  ( -54.44999999999997442, 0.000000000000000000, 0.000000000000000000 ) ) ;
#3839=AXIS2_PLACEMENT_3D ( 'NONE', #10193, #5277, #19720 ) ;
#3840=AXIS2_PLACEMENT_3D ( 'NONE', #13794, #18748, #6694 ) ;
#3842=CARTESIAN_POINT ( 'NONE',  ( 15.03925126672132961, -2.686240680702127737, -4.475885388010735433 ) ) ;
#3850=CIRCLE ( 'NONE', #18015, 0.05000000000000012768 ) ;
#3859=ORIENTED_EDGE ( 'NONE', *, *, #30155, .T. ) ;
#3864=CIRCLE ( 'NONE', #30640, 4.000000000000022204 ) ;
#3867=ORIENTED_EDGE ( 'NONE', *, *, #8777, .T. ) ;
#3868=AXIS2_PLACEMENT_3D ( 'NONE', #22289, #7698, #5794 ) ;
#3871=EDGE_LOOP ( 'NONE', ( #16670, #13448, #102, #26624 ) ) ;
#3876=DIRECTION ( 'NONE',  ( 0.000000000000000000, 1.000000000000000000, 0.000000000000000000 ) ) ;
#3878=CARTESIAN_POINT ( 'NONE',  ( 57.05000000000001847, -0.8156862745098041323, -2.468735688885368873 ) ) ;
#3887=CIRCLE ( 'NONE', #5403, 0.09999999999999997780 ) ;
#3893=AXIS2_PLACEMENT_3D ( 'NONE', #29048, #7357, #4987 ) ;
#3903=CARTESIAN_POINT ( 'NONE',  ( 47.00000000000002132, 1.734723475976807094E-15, 4.275000000000000355 ) ) ;
#3904=CARTESIAN_POINT ( 'NONE',  ( -36.31414349454750123, 3.102491976071082735, 4.173461118157660188 ) ) ;
#3918=CARTESIAN_POINT ( 'NONE',  ( -36.58361892165972762, 5.109611055794863077, -1.772889539330479547 ) ) ;
#3926=CARTESIAN_POINT ( 'NONE',  ( 15.30042582489668312, 4.018128186974561089, 3.618665893507494236 ) ) ;
#3931=TOROIDAL_SURFACE ( 'NONE', #28718, 4.000000000000022204, 0.1000000000000000056 ) ;
#3935=DIRECTION ( 'NONE',  ( -1.000000000000000000, 0.000000000000000000, -0.000000000000000000 ) ) ;
#3940=CARTESIAN_POINT ( 'NONE',  ( 48.38577482684819131, 1.132063507975338945, 3.941224428058327511 ) ) ;
#3943=CYLINDRICAL_SURFACE ( 'NONE', #1723, 5.407411300779133789 ) ;
#3953=CARTESIAN_POINT ( 'NONE',  ( -54.49999999999997868, -1.549999999999999600, 4.064480286580312907 ) ) ;
#3957=CARTESIAN_POINT ( 'NONE',  ( -36.38012252111052902, 2.292272662152775364, -4.901537128432196688 ) ) ;
#3965=TOROIDAL_SURFACE ( 'NONE', #23703, 3.675000000000000711, 0.05000000000000000278 ) ;
#3969=VERTEX_POINT ( 'NONE', #2430 ) ;
#3972=DIRECTION ( 'NONE',  ( 0.000000000000000000, 0.000000000000000000, -1.000000000000000000 ) ) ;
#3975=FACE_OUTER_BOUND ( 'NONE', #3204, .T. ) ;
#3989=CARTESIAN_POINT ( 'NONE',  ( 56.95220615073115056, 0.7055010433615873655, -1.764201441664152270 ) ) ;
#3991=EDGE_CURVE ( 'NONE', #8886, #28473, #21186, .T. ) ;
#3992=EDGE_LOOP ( 'NONE', ( #21304, #17259, #23825, #18720 ) ) ;
#3999=CARTESIAN_POINT ( 'NONE',  ( 58.50000000000001421, 0.8000000000000000444, 2.421260002560650104 ) ) ;
#4007=CARTESIAN_POINT ( 'NONE',  ( 47.00000000000002132, -1.426739617975173013, 3.843750000000023093 ) ) ;
#4011=DIRECTION ( 'NONE',  ( 3.167104333282667910E-32, -1.224646799147353207E-16, 1.000000000000000000 ) ) ;
#4012=ORIENTED_EDGE ( 'NONE', *, *, #1082, .T. ) ;
#4013=CARTESIAN_POINT ( 'NONE',  ( 58.50000000000001421, -0.8000000000000000444, -2.421260002560650104 ) ) ;
#4017=FILL_AREA_STYLE_COLOUR ( '', #28031 ) ;
#4020=CARTESIAN_POINT ( 'NONE',  ( 56.95349779155813508, 0.7404564066163630276, -2.492333105726597164 ) ) ;
#4022=ORIENTED_EDGE ( 'NONE', *, *, #17072, .T. ) ;
#4041=CARTESIAN_POINT ( 'NONE',  ( 15.59140265158955962, 2.334862116274945887, 4.877703086529577625 ) ) ;
#4043=CARTESIAN_POINT ( 'NONE',  ( 50.40000000000001990, 1.409787217987196861, -3.950000000000022826 ) ) ;
#4044=CIRCLE ( 'NONE', #5043, 4.375000000000000000 ) ;
#4045=CARTESIAN_POINT ( 'NONE',  ( 57.02678890911435872, 0.7442859487862443224, -1.783438914669892128 ) ) ;
#4046=CARTESIAN_POINT ( 'NONE',  ( -36.25997906085271438, -2.880023619481960839, 4.335093843541793390 ) ) ;
#4047=CARTESIAN_POINT ( 'NONE',  ( -35.85663232820584057, 4.804073783693455724, -2.042134687550314354 ) ) ;
#4048=AXIS2_PLACEMENT_3D ( 'NONE', #16712, #31091, #18769 ) ;
#4049=CARTESIAN_POINT ( 'NONE',  ( 51.78962428791817274, -4.157296476791675133, 1.048491968755490555 ) ) ;
#4051=CARTESIAN_POINT ( 'NONE',  ( 57.05000000000001847, 0.8000000000000002665, -2.421260002560650104 ) ) ;
#4053=ORIENTED_EDGE ( 'NONE', *, *, #15994, .T. ) ;
#4056=VERTEX_POINT ( 'NONE', #13006 ) ;
#4059=CARTESIAN_POINT ( 'NONE',  ( 15.03925126672132784, 4.945493884734818657, -1.606888370749675499 ) ) ;
#4060=CARTESIAN_POINT ( 'NONE',  ( -36.48174642953001978, 3.496282614933940991, 4.130238739723520958 ) ) ;
#4068=DIRECTION ( 'NONE',  ( -2.459562394685755126E-16, 0.9510565162951566398, -0.3090169943749383474 ) ) ;
#4075=EDGE_CURVE ( 'NONE', #25905, #30422, #3127, .T. ) ;
#4077=CARTESIAN_POINT ( 'NONE',  ( -35.85663232820584057, -2.686240680702151717, -4.475885388010727439 ) ) ;
#4078=ADVANCED_FACE ( 'NONE', ( #30257 ), #23152, .T. ) ;
#4080=CARTESIAN_POINT ( 'NONE',  ( 47.00000000000002132, -3.726179070414207928, 1.710435481158852244 ) ) ;
#4082=EDGE_CURVE ( 'NONE', #23319, #247, #678, .T. ) ;
#4086=CARTESIAN_POINT ( 'NONE',  ( -36.58413561666693425, -0.1030603059131488530, 5.407440145940149989 ) ) ;
#4087=CIRCLE ( 'NONE', #17757, 0.1000000000000000472 ) ;
#4088=CARTESIAN_POINT ( 'NONE',  ( 48.40134283869316789, 0.9106118309513187015, -3.923752762110599424 ) ) ;
#4091=EDGE_LOOP ( 'NONE', ( #15490, #29293 ) ) ;
#4096=EDGE_LOOP ( 'NONE', ( #14308, #18177, #562, #6679 ) ) ;
#4099=PLANE ( 'NONE',  #10991 ) ;
#4105=TOROIDAL_SURFACE ( 'NONE', #8156, 1.949999999999999956, 0.05000000000000000278 ) ;
#4111=CARTESIAN_POINT ( 'NONE',  ( 57.04037853559506743, -0.7490840064628494499, 1.779165039991060571 ) ) ;
#4116=EDGE_CURVE ( 'NONE', #3567, #26982, #21429, .T. ) ;
#4117=VECTOR ( 'NONE', #4940, 1000.000000000000000 ) ;
#4119=DIRECTION ( 'NONE',  ( 0.000000000000000000, 0.000000000000000000, -1.000000000000000000 ) ) ;
#4123=VERTEX_POINT ( 'NONE', #12833 ) ;
#4124=AXIS2_PLACEMENT_3D ( 'NONE', #22932, #4223, #27679 ) ;
#4125=DIRECTION ( 'NONE',  ( 1.000000000000000000, 0.000000000000000000, 0.000000000000000000 ) ) ;
#4127=CARTESIAN_POINT ( 'NONE',  ( 48.30000000000001847, 2.428612866367529932E-14, 0.000000000000000000 ) ) ;
#4128=CARTESIAN_POINT ( 'NONE',  ( -36.31414349454749413, 4.963067629822528026, 1.552801941062302182 ) ) ;
#4129=CARTESIAN_POINT ( 'NONE',  ( 15.57907767661756182, -5.286410563980378008, 1.167394352644079092 ) ) ;
#4137=VERTEX_POINT ( 'NONE', #818 ) ;
#4139=ORIENTED_EDGE ( 'NONE', *, *, #30205, .F. ) ;
#4144=ORIENTED_EDGE ( 'NONE', *, *, #18455, .F. ) ;
#4147=ORIENTED_EDGE ( 'NONE', *, *, #21499, .F. ) ;
#4149=CARTESIAN_POINT ( 'NONE',  ( 58.45000000000001705, -0.7500000000000000000, -2.421260002560649660 ) ) ;
#4150=DIRECTION ( 'NONE',  ( 1.000000000000000000, 0.000000000000000000, 0.000000000000000000 ) ) ;
#4153=EDGE_CURVE ( 'NONE', #26067, #3458, #8707, .T. ) ;
#4157=CYLINDRICAL_SURFACE ( 'NONE', #3840, 0.1000000000000000472 ) ;
#4159=CARTESIAN_POINT ( 'NONE',  ( 57.05000000000001847, 0.8156862745098039102, -2.468735688885368873 ) ) ;
#4161=ORIENTED_EDGE ( 'NONE', *, *, #27382, .T. ) ;
#4162=CARTESIAN_POINT ( 'NONE',  ( 48.30000000000001847, 0.6462379109120995890, -4.048750000000023164 ) ) ;
#4163=CARTESIAN_POINT ( 'NONE',  ( 50.39869454013827976, -0.9107929593199907137, 3.923749358243191043 ) ) ;
#4166=ORIENTED_EDGE ( 'NONE', *, *, #30155, .F. ) ;
#4176=VERTEX_POINT ( 'NONE', #26298 ) ;
#4181=ORIENTED_EDGE ( 'NONE', *, *, #1277, .F. ) ;
#4188=CARTESIAN_POINT ( 'NONE',  ( 16.10660252424456473, 3.410993390446818374, 4.205682099886888459 ) ) ;
#4189=ADVANCED_FACE ( 'NONE', ( #11733 ), #22935, .T. ) ;
#4190=DIRECTION ( 'NONE',  ( 1.000000000000000000, 0.000000000000000000, 0.000000000000000000 ) ) ;
#4191=CARTESIAN_POINT ( 'NONE',  ( 57.04767748491563140, 0.7500000000000049960, -1.778341924377874639 ) ) ;
#4192=CARTESIAN_POINT ( 'NONE',  ( -35.98952425903311791, -2.686240675664594235, 4.475885398016349548 ) ) ;
#4197=CARTESIAN_POINT ( 'NONE',  ( 54.50000000000002132, -0.003244837758135472351, 4.274998768541100169 ) ) ;
#4198=CIRCLE ( 'NONE', #26470, 4.375000000000000000 ) ;
#4205=ADVANCED_FACE ( 'NONE', ( #16003 ), #11245, .F. ) ;
#4209=CARTESIAN_POINT ( 'NONE',  ( -36.23324115033521764, 2.840672495176659318, 4.363684107482471930 ) ) ;
#4211=FACE_OUTER_BOUND ( 'NONE', #7307, .T. ) ;
#4218=ORIENTED_EDGE ( 'NONE', *, *, #2634, .T. ) ;
#4219=CARTESIAN_POINT ( 'NONE',  ( 57.05000000000001137, -0.7794871794871797155, 1.732743413496401930 ) ) ;
#4223=DIRECTION ( 'NONE',  ( -1.520093157366847861E-16, 0.5877852522924624790, 0.8090169943749551118 ) ) ;
#4226=CARTESIAN_POINT ( 'NONE',  ( 51.84429591523409897, 0.2531794267987216851, 4.351658421183466352 ) ) ;
#4228=CARTESIAN_POINT ( 'NONE',  ( 50.38476904405314372, 1.115727354199254950, -3.895947837398489266 ) ) ;
#4231=EDGE_LOOP ( 'NONE', ( #5289, #23761, #22530, #22067 ) ) ;
#4235=CARTESIAN_POINT ( 'NONE',  ( -36.68133364217572989, 0.7247683022688486965, 5.358970532132285136 ) ) ;
#4236=DIRECTION ( 'NONE',  ( 0.000000000000000000, 0.000000000000000000, 1.000000000000000000 ) ) ;
#4239=LINE ( 'NONE', #23575, #6737 ) ;
#4242=AXIS2_PLACEMENT_3D ( 'NONE', #7911, #5853, #25324 ) ;
#4244=ORIENTED_EDGE ( 'NONE', *, *, #27945, .T. ) ;
#4246=DIRECTION ( 'NONE',  ( 0.000000000000000000, 0.000000000000000000, 1.000000000000000000 ) ) ;
#4258=ORIENTED_EDGE ( 'NONE', *, *, #12404, .T. ) ;
#4259=AXIS2_PLACEMENT_3D ( 'NONE', #600, #29562, #12939 ) ;
#4260=CARTESIAN_POINT ( 'NONE',  ( 15.03925126672132961, -2.686240680702165928, 4.475885388010711452 ) ) ;
#4262=CARTESIAN_POINT ( 'NONE',  ( -36.11122220296831387, 2.734418404389770796, -4.440882220947520054 ) ) ;
#4266=CARTESIAN_POINT ( 'NONE',  ( 15.90468948301722918, 0.6818242347930796310, -5.365311767243446717 ) ) ;
#4267=DIRECTION ( 'NONE',  ( 0.000000000000000000, -1.000000000000000000, 0.000000000000000000 ) ) ;
#4275=EDGE_CURVE ( 'NONE', #8161, #19631, #25664, .T. ) ;
#4277=DIRECTION ( 'NONE',  ( -1.000000000000000000, -0.000000000000000000, -0.000000000000000000 ) ) ;
#4278=CARTESIAN_POINT ( 'NONE',  ( -36.89017861347081606, 5.235729994560179179, 1.359191621353925905 ) ) ;
#4283=CARTESIAN_POINT ( 'NONE',  ( -36.42771574642760868, -4.977801270594346406, 2.126472881633285628 ) ) ;
#4286=AXIS2_PLACEMENT_3D ( 'NONE', #29880, #30023, #745 ) ;
#4288=ORIENTED_EDGE ( 'NONE', *, *, #3028, .F. ) ;
#4292=EDGE_CURVE ( 'NONE', #3728, #7731, #21180, .T. ) ;
#4294=ORIENTED_EDGE ( 'NONE', *, *, #6688, .F. ) ;
#4302=CIRCLE ( 'NONE', #9383, 0.4576450603546999840 ) ;
#4305=CARTESIAN_POINT ( 'NONE',  ( -36.00197790576392265, 5.377732432866631385, -0.5657657256215206099 ) ) ;
#4307=CARTESIAN_POINT ( 'NONE',  ( 57.05000000000001847, -0.8156862745098041323, -2.468735688885368873 ) ) ;
#4308=DIRECTION ( 'NONE',  ( 1.000000000000000000, 2.586136946169074517E-16, -0.000000000000000000 ) ) ;
#4310=CARTESIAN_POINT ( 'NONE',  ( -36.00201293083839715, -4.018128179617960427, -3.618665901676318075 ) ) ;
#4313=DIRECTION ( 'NONE',  ( 1.000000000000000000, 0.000000000000000000, 0.000000000000000000 ) ) ;
#4319=DIRECTION ( 'NONE',  ( 1.000000000000000000, -0.000000000000000000, -0.000000000000000000 ) ) ;
#4320=ORIENTED_EDGE ( 'NONE', *, *, #19627, .T. ) ;
#4327=CARTESIAN_POINT ( 'NONE',  ( 15.49676243306308088, 4.927920137446221815, 1.660974799722156892 ) ) ;
#4328=ORIENTED_EDGE ( 'NONE', *, *, #21675, .T. ) ;
#4331=EDGE_CURVE ( 'NONE', #6201, #31046, #3467, .T. ) ;
#4334=DIRECTION ( 'NONE',  ( 0.000000000000000000, -1.517883041479702421E-14, -1.000000000000000000 ) ) ;
#4344=CARTESIAN_POINT ( 'NONE',  ( 57.01033040358699111, -0.8080171122822069618, -2.471263581425196421 ) ) ;
#4345=VERTEX_POINT ( 'NONE', #8863 ) ;
#4355=EDGE_CURVE ( 'NONE', #29040, #1141, #13568, .T. ) ;
#4369=CARTESIAN_POINT ( 'NONE',  ( -36.38012252111052902, 3.953287617511453078, 3.694739123711269890 ) ) ;
#4370=ORIENTED_EDGE ( 'NONE', *, *, #29219, .F. ) ;
#4374=CARTESIAN_POINT ( 'NONE',  ( 56.95000000000001705, 0.000000000000000000, 0.000000000000000000 ) ) ;
#4376=EDGE_LOOP ( 'NONE', ( #3161, #15196, #21884, #16621, #7858 ) ) ;
#4377=CARTESIAN_POINT ( 'NONE',  ( 50.33814819168215138, 1.426738236278596972, 3.843750512866276559 ) ) ;
#4378=DIRECTION ( 'NONE',  ( 0.000000000000000000, 0.000000000000000000, 1.000000000000000000 ) ) ;
#4380=ORIENTED_EDGE ( 'NONE', *, *, #8875, .F. ) ;
#4381=CYLINDRICAL_SURFACE ( 'NONE', #2546, 0.05000000000000143219 ) ;
#4384=AXIS2_PLACEMENT_3D ( 'NONE', #7289, #14098, #21 ) ;
#4385=CARTESIAN_POINT ( 'NONE',  ( -54.45495050826418293, -1.500000000000000000, -3.300094695611020867 ) ) ;
#4391=CARTESIAN_POINT ( 'NONE',  ( 51.87254251396529980, 0.05753116748212284276, 4.370911451931760894 ) ) ;
#4395=DIRECTION ( 'NONE',  ( 1.000000000000000000, 0.000000000000000000, 0.000000000000000000 ) ) ;
#4401=AXIS2_PLACEMENT_3D ( 'NONE', #29, #2398, #28076 ) ;
#4405=CARTESIAN_POINT ( 'NONE',  ( -35.85663232820596136, -0.7747498368337714103, 5.363501452440941897 ) ) ;
#4408=CARTESIAN_POINT ( 'NONE',  ( -36.40793637698146057, -5.360541651686778764, 0.7128348320083932599 ) ) ;
#4412=LINE ( 'NONE', #16620, #28304 ) ;
#4414=ORIENTED_EDGE ( 'NONE', *, *, #14813, .F. ) ;
#4416=AXIS2_PLACEMENT_3D ( 'NONE', #25261, #12305, #19460 ) ;
#4421=AXIS2_PLACEMENT_3D ( 'NONE', #21859, #26273, #146 ) ;
#4427=CARTESIAN_POINT ( 'NONE',  ( -54.49131719536980967, 1.521332553059528081, -4.044684194243342468 ) ) ;
#4435=CARTESIAN_POINT ( 'NONE',  ( -36.11780688638067716, 4.018128186974130323, -3.618665893507954756 ) ) ;
#4440=DIRECTION ( 'NONE',  ( -1.000000000000000000, -0.000000000000000000, -0.000000000000000000 ) ) ;
#4442=LINE ( 'NONE', #31199, #2336 ) ;
#4443=CARTESIAN_POINT ( 'NONE',  ( 50.30000000000001847, -1.391941090707485396, 3.850000000000022737 ) ) ;
#4444=LINE ( 'NONE', #26133, #26123 ) ;
#4445=ORIENTED_EDGE ( 'NONE', *, *, #5485, .F. ) ;
#4449=CARTESIAN_POINT ( 'NONE',  ( -36.92443669619682112, 5.094475812726813935, 1.819860688632667367 ) ) ;
#4450=CARTESIAN_POINT ( 'NONE',  ( 15.86395258069124203, -5.320649567603481955, 0.9667173501064290075 ) ) ;
#4456=ORIENTED_EDGE ( 'NONE', *, *, #11758, .T. ) ;
#4461=( NAMED_UNIT ( * ) PLANE_ANGLE_UNIT ( ) SI_UNIT ( $, .RADIAN. ) );
#4463=ORIENTED_EDGE ( 'NONE', *, *, #28999, .T. ) ;
#4470=EDGE_CURVE ( 'NONE', #17229, #13576, #28758, .T. ) ;
#4476=CARTESIAN_POINT ( 'NONE',  ( -36.14504829323105639, 4.698774973472866101, -2.676767126782043427 ) ) ;
#4478=LINE ( 'NONE', #14129, #19077 ) ;
#4479=DIRECTION ( 'NONE',  ( 1.000000000000000000, 0.000000000000000000, 0.000000000000000000 ) ) ;
#4480=CARTESIAN_POINT ( 'NONE',  ( -36.52679053911623441, -2.412550141807427106, -4.840569432287353813 ) ) ;
#4481=B_SPLINE_CURVE_WITH_KNOTS ( 'NONE', 3,
 ( #25389, #1314, #20200, #27300, #24767, #6086, #8453, #18133, #29979, #18279, #22557, #3231 ),
 .UNSPECIFIED., .F., .F.,
 ( 4, 2, 2, 2, 2, 4 ),
 ( 0.000000000000000000, 5.522938194211729973E-05, 0.0001104587638842345995, 0.0002209175277684801765, 0.0004418350555369711949, 0.0008836701110739511719 ),
 .UNSPECIFIED. ) ;
#4483=VERTEX_POINT ( 'NONE', #15034 ) ;
#4484=DIRECTION ( 'NONE',  ( -1.000000000000000000, -0.000000000000000000, -0.000000000000000000 ) ) ;
#4491=ORIENTED_EDGE ( 'NONE', *, *, #1688, .T. ) ;
#4496=CARTESIAN_POINT ( 'NONE',  ( 15.98305126557427869, 4.951626736499044057, 2.174059107776793454 ) ) ;
#4498=VERTEX_POINT ( 'NONE', #2553 ) ;
#4503=CARTESIAN_POINT ( 'NONE',  ( 48.30000000000001847, 2.478823385132571406E-14, 4.100000000000022737 ) ) ;
#4506=ORIENTED_EDGE ( 'NONE', *, *, #29746, .F. ) ;
#4510=ADVANCED_FACE ( 'NONE', ( #7607 ), #30250, .T. ) ;
#4515=CARTESIAN_POINT ( 'NONE',  ( 50.50000000000002132, 2.428612866367529932E-14, 0.000000000000000000 ) ) ;
#4518=FACE_OUTER_BOUND ( 'NONE', #29031, .T. ) ;
#4524=EDGE_CURVE ( 'NONE', #21420, #12623, #3529, .T. ) ;
#4526=ORIENTED_EDGE ( 'NONE', *, *, #27619, .T. ) ;
#4529=DIRECTION ( 'NONE',  ( 1.000000000000000000, 0.000000000000000000, 0.000000000000000000 ) ) ;
#4532=CARTESIAN_POINT ( 'NONE',  ( -36.80043232705877898, 3.597789892641451104, 4.037455662930098832 ) ) ;
#4533=ORIENTED_EDGE ( 'NONE', *, *, #5340, .T. ) ;
#4540=EDGE_LOOP ( 'NONE', ( #15894, #24992, #23976, #20010 ) ) ;
#4545=FACE_BOUND ( 'NONE', #19947, .T. ) ;
#4548=CARTESIAN_POINT ( 'NONE',  ( 15.03925126672133139, -5.377732432866647372, 0.5657657256215454789 ) ) ;
#4550=CARTESIAN_POINT ( 'NONE',  ( 15.03925126672123369, -4.683225679163331101, -2.703237727951255387 ) ) ;
#4555=CARTESIAN_POINT ( 'NONE',  ( 50.50000000000002132, 2.428612866367529932E-14, 0.000000000000000000 ) ) ;
#4564=ORIENTED_EDGE ( 'NONE', *, *, #10947, .T. ) ;
#4580=CARTESIAN_POINT ( 'NONE',  ( -36.00201293083839005, 4.018128179617898255, 3.618665901676350938 ) ) ;
#4588=CARTESIAN_POINT ( 'NONE',  ( -36.04581030752699888, 3.779372845002908932, -3.883777290284648576 ) ) ;
#4589=CARTESIAN_POINT ( 'NONE',  ( 48.37784963381696457, 1.308847734660516071, -3.885629509820973659 ) ) ;
#4593=CYLINDRICAL_SURFACE ( 'NONE', #6962, 1.000000000000000000 ) ;
#4598=DIRECTION ( 'NONE',  ( -1.000000000000000000, -0.000000000000000000, -0.000000000000000000 ) ) ;
#4600=CARTESIAN_POINT ( 'NONE',  ( 16.10624235918717773, -3.046685255238767986, -4.470266847515925512 ) ) ;
#4601=CARTESIAN_POINT ( 'NONE',  ( -36.68866260399369850, 4.872353571451107257, 2.347449169364858701 ) ) ;
#4602=CARTESIAN_POINT ( 'NONE',  ( 15.03925126672133317, -4.861582140531632845, 2.394243978978315646 ) ) ;
#4611=ORIENTED_EDGE ( 'NONE', *, *, #28999, .F. ) ;
#4621=DIRECTION ( 'NONE',  ( 1.000000000000000000, 0.000000000000000000, 0.000000000000000000 ) ) ;
#4626=CARTESIAN_POINT ( 'NONE',  ( -41.12388279035661753, -1.755788972190012401E-14, 0.000000000000000000 ) ) ;
#4630=CYLINDRICAL_SURFACE ( 'NONE', #23584, 3.625000000000028866 ) ;
#4635=CARTESIAN_POINT ( 'NONE',  ( 50.38693217303928407, -1.296871156637275702, 3.889656364559860080 ) ) ;
#4645=CARTESIAN_POINT ( 'NONE',  ( 34.55000000000001847, 0.000000000000000000, 0.000000000000000000 ) ) ;
#4649=CARTESIAN_POINT ( 'NONE',  ( 15.41080140630216988, 4.895960019030393795, 2.323379425334584081 ) ) ;
#4650=ORIENTED_EDGE ( 'NONE', *, *, #12450, .T. ) ;
#4651=VECTOR ( 'NONE', #3785, 1000.000000000000000 ) ;
#4662=LINE ( 'NONE', #9427, #25032 ) ;
#4664=ORIENTED_EDGE ( 'NONE', *, *, #27378, .F. ) ;
#4666=DIRECTION ( 'NONE',  ( 1.000000000000000000, 0.000000000000000000, 0.000000000000000000 ) ) ;
#4667=CARTESIAN_POINT ( 'NONE',  ( 47.00000000000002132, -3.976179070414207928, -1.000000000000000000 ) ) ;
#4673=EDGE_CURVE ( 'NONE', #2624, #4056, #16618, .T. ) ;
#4683=ORIENTED_EDGE ( 'NONE', *, *, #31020, .F. ) ;
#4688=CARTESIAN_POINT ( 'NONE',  ( -36.72207054450174724, 5.313409993919671948, 1.009519134730257228 ) ) ;
#4689=ORIENTED_EDGE ( 'NONE', *, *, #2821, .T. ) ;
#4692=CARTESIAN_POINT ( 'NONE',  ( 57.00074754615238248, 0.7099475343046129927, 1.812279303590036639 ) ) ;
#4694=CARTESIAN_POINT ( 'NONE',  ( -54.48833221701376317, -1.517896399908648108, -3.311598511234999709 ) ) ;
#4702=VERTEX_POINT ( 'NONE', #27994 ) ;
#4707=EDGE_CURVE ( 'NONE', #12071, #26982, #10685, .T. ) ;
#4708=CARTESIAN_POINT ( 'NONE',  ( -54.49999516060625382, 1.549196738101655590, 4.063926895246979143 ) ) ;
#4709=( BOUNDED_SURFACE ( )  B_SPLINE_SURFACE ( 3, 2, ( 
 ( #28864, #28713, #11608 ),
 ( #6849, #2423, #16838 ),
 ( #7176, #12084, #21291 ),
 ( #26477, #191, #28540 ),
 ( #21760, #26796, #19524 ),
 ( #16991, #11761, #21436 ) ),
 .UNSPECIFIED., .F., .F., .F. ) 
 B_SPLINE_SURFACE_WITH_KNOTS ( ( 4, 2, 4 ),
 ( 3, 3 ),
 ( 0.0001319104779587709254, 0.0002905946498119449514, 0.0004492788216651190315 ),
 ( 0.000000000000000000, 1.000000000000000000 ),
 .UNSPECIFIED. ) 
 GEOMETRIC_REPRESENTATION_ITEM ( )  RATIONAL_B_SPLINE_SURFACE ( (
 ( 1.000000000000000000, 0.7779866052154992273, 1.000000000000000000),
 ( 1.000000000000000000, 0.7780052684394881402, 1.000000000000000000),
 ( 1.000000000000000000, 0.7724636952541197310, 1.000000000000000000),
 ( 1.000000000000000000, 0.7490013934199948320, 1.000000000000000000),
 ( 1.000000000000000000, 0.7305684325697214820, 1.000000000000000000),
 ( 1.000000000000000000, 0.7071067811865471286, 1.000000000000000000) ) ) 
 REPRESENTATION_ITEM ( '' )  SURFACE ( )  );
#4715=DIRECTION ( 'NONE',  ( 0.000000000000000000, 1.000000000000000000, 0.000000000000000000 ) ) ;
#4726=ORIENTED_EDGE ( 'NONE', *, *, #1365, .T. ) ;
#4729=CARTESIAN_POINT ( 'NONE',  ( 15.39414421509790287, -3.291455042465448511, 4.036171416105464260 ) ) ;
#4738=DIRECTION ( 'NONE',  ( 1.000000000000000000, 5.172273892338137201E-16, 0.000000000000000000 ) ) ;
#4743=UNCERTAINTY_MEASURE_WITH_UNIT (LENGTH_MEASURE( 1.000000000000000082E-05 ), #18140, 'distance_accuracy_value', 'NONE');
#4748=CARTESIAN_POINT ( 'NONE',  ( -35.85663232820583346, 3.817150320979498357, 2.203324261493436520 ) ) ;
#4750=ORIENTED_EDGE ( 'NONE', *, *, #27378, .T. ) ;
#4755=CARTESIAN_POINT ( 'NONE',  ( 57.01810253486932112, 0.8103601741748552856, -2.470489098966295316 ) ) ;
#4759=CARTESIAN_POINT ( 'NONE',  ( -36.68866260399371271, -4.872353571451353282, -2.347449169364439925 ) ) ;
#4761=( LENGTH_UNIT ( ) NAMED_UNIT ( * ) SI_UNIT ( .MILLI., .METRE. ) );
#4763=EDGE_CURVE ( 'NONE', #6711, #18916, #31319, .T. ) ;
#4767=ORIENTED_EDGE ( 'NONE', *, *, #26690, .F. ) ;
#4769=CARTESIAN_POINT ( 'NONE',  ( 50.49731030164353029, 0.9327905306641951499, 3.995066436131523346 ) ) ;
#4771=AXIS2_PLACEMENT_3D ( 'NONE', #15325, #1221, #5674 ) ;
#4772=CARTESIAN_POINT ( 'NONE',  ( -54.45996984137642727, -1.500763111530254434, 3.300586169551323223 ) ) ;
#4773=ADVANCED_FACE ( 'NONE', ( #134 ), #8729, .T. ) ;
#4776=CARTESIAN_POINT ( 'NONE',  ( -36.92362342067168868, -0.1627367787821575318, -5.407318510437578496 ) ) ;
#4782=ORIENTED_EDGE ( 'NONE', *, *, #10819, .T. ) ;
#4788=CARTESIAN_POINT ( 'NONE',  ( 48.43389689255278796, -1.399562922973020429, 3.853849143137397792 ) ) ;
#4789=CARTESIAN_POINT ( 'NONE',  ( 50.40671278470074412, -1.343285922954033040, 3.873819829599201015 ) ) ;
#4793=CYLINDRICAL_SURFACE ( 'NONE', #30152, 4.375000000000000000 ) ;
#4794=EDGE_LOOP ( 'NONE', ( #11511, #7083, #6770 ) ) ;
#4800=CARTESIAN_POINT ( 'NONE',  ( 15.61033468494287391, 4.977801270594249594, 2.126472881633401091 ) ) ;
#4805=FACE_OUTER_BOUND ( 'NONE', #12100, .T. ) ;
#4806=CARTESIAN_POINT ( 'NONE',  ( -35.85663232820584057, -4.945493884734809775, 1.606888370749721684 ) ) ;
#4815=ORIENTED_EDGE ( 'NONE', *, *, #4331, .F. ) ;
#4816=DIRECTION ( 'NONE',  ( 0.000000000000000000, 1.000000000000000000, 0.000000000000000000 ) ) ;
#4818=CARTESIAN_POINT ( 'NONE',  ( 57.00000000000001421, 0.000000000000000000, 0.000000000000000000 ) ) ;
#4821=EDGE_CURVE ( 'NONE', #27463, #2662, #15221, .T. ) ;
#4823=FACE_OUTER_BOUND ( 'NONE', #2485, .T. ) ;
#4827=CIRCLE ( 'NONE', #9897, 3.675000000000000711 ) ;
#4830=ORIENTED_EDGE ( 'NONE', *, *, #14813, .T. ) ;
#4831=FACE_OUTER_BOUND ( 'NONE', #29175, .T. ) ;
#4832=ORIENTED_EDGE ( 'NONE', *, *, #20783, .F. ) ;
#4833=DIRECTION ( 'NONE',  ( 0.000000000000000000, 0.000000000000000000, -1.000000000000000000 ) ) ;
#4839=ORIENTED_EDGE ( 'NONE', *, *, #8216, .T. ) ;
#4845=CARTESIAN_POINT ( 'NONE',  ( -36.81959771849334828, 4.939398376933260337, 2.210903708596522410 ) ) ;
#4850=CARTESIAN_POINT ( 'NONE',  ( 33.47623932017462778, -2.199885893005940840, 4.939696249117685234 ) ) ;
#4858=AXIS2_PLACEMENT_3D ( 'NONE', #11044, #1212, #30495 ) ;
#4859=CIRCLE ( 'NONE', #24560, 0.7500000000000001110 ) ;
#4862=VERTEX_POINT ( 'NONE', #11971 ) ;
#4864=CARTESIAN_POINT ( 'NONE',  ( -36.40793637698146057, -0.9785522574022036402, 5.318456145981289573 ) ) ;
#4870=ADVANCED_FACE ( 'NONE', ( #16884 ), #17051, .T. ) ;
#4871=CARTESIAN_POINT ( 'NONE',  ( -54.49983703358571319, 1.542636180423125225, 4.059406436927349482 ) ) ;
#4874=CARTESIAN_POINT ( 'NONE',  ( 15.68751737981905947, 0.3564988296781282928, -5.398869307934854866 ) ) ;
#4877=ORIENTED_EDGE ( 'NONE', *, *, #22395, .F. ) ;
#4879=FACE_OUTER_BOUND ( 'NONE', #5294, .T. ) ;
#4881=AXIS2_PLACEMENT_3D ( 'NONE', #15224, #22837, #8559 ) ;
#4883=CARTESIAN_POINT ( 'NONE',  ( -54.49608498031047787, -1.530604779201329535, -4.051096982736679841 ) ) ;
#4884=ORIENTED_EDGE ( 'NONE', *, *, #25906, .T. ) ;
#4887=FACE_OUTER_BOUND ( 'NONE', #21748, .T. ) ;
#4890=DIRECTION ( 'NONE',  ( -1.000000000000000000, -0.000000000000000000, -0.000000000000000000 ) ) ;
#4893=FACE_OUTER_BOUND ( 'NONE', #12551, .T. ) ;
#4895=ADVANCED_FACE ( 'NONE', ( #14180 ), #4105, .T. ) ;
#4902=AXIS2_PLACEMENT_3D ( 'NONE', #6658, #30397, #16320 ) ;
#4910=ORIENTED_EDGE ( 'NONE', *, *, #4673, .T. ) ;
#4913=CIRCLE ( 'NONE', #22636, 0.05000000000000012768 ) ;
#4917=DIRECTION ( 'NONE',  ( 1.000000000000000000, 0.000000000000000000, 0.000000000000000000 ) ) ;
#4918=ORIENTED_EDGE ( 'NONE', *, *, #28677, .F. ) ;
#4920=DIRECTION ( 'NONE',  ( 0.000000000000000000, 0.000000000000000000, -1.000000000000000000 ) ) ;
#4936=ADVANCED_FACE ( 'NONE', ( #26377 ), #97, .T. ) ;
#4940=DIRECTION ( 'NONE',  ( 0.000000000000000000, 0.000000000000000000, 1.000000000000000000 ) ) ;
#4941=CARTESIAN_POINT ( 'NONE',  ( -54.44999999999997442, -1.500000000000000000, 3.300094695611020867 ) ) ;
#4945=CARTESIAN_POINT ( 'NONE',  ( -36.89017861347081606, -0.3252614978953602964, -5.399488438498864618 ) ) ;
#4949=CARTESIAN_POINT ( 'NONE',  ( 15.70940947763171280, -2.412550141807447091, 4.840569432287336049 ) ) ;
#4953=ADVANCED_FACE ( 'NONE', ( #4996 ), #10063, .F. ) ;
#4954=CIRCLE ( 'NONE', #7987, 1.000000000000000000 ) ;
#4955=CARTESIAN_POINT ( 'NONE',  ( 15.03925126672133139, -4.817150320980666756, 2.203324261490539282 ) ) ;
#4956=CARTESIAN_POINT ( 'NONE',  ( -36.14490256869204643, -4.698781674909506378, -2.676750094560167881 ) ) ;
#4957=FACE_OUTER_BOUND ( 'NONE', #7909, .T. ) ;
#4961=FACE_OUTER_BOUND ( 'NONE', #22319, .T. ) ;
#4962=VERTEX_POINT ( 'NONE', #11811 ) ;
#4970=LINE ( 'NONE', #29342, #19734 ) ;
#4973=DIRECTION ( 'NONE',  ( 1.000000000000000000, 3.125586771759065906E-16, 0.000000000000000000 ) ) ;
#4981=EDGE_CURVE ( 'NONE', #25975, #1935, #19962, .T. ) ;
#4986=CARTESIAN_POINT ( 'NONE',  ( 57.04458252721509126, -0.7500000000000000000, 2.421260002560649660 ) ) ;
#4987=DIRECTION ( 'NONE',  ( 0.000000000000000000, 0.000000000000000000, 1.000000000000000000 ) ) ;
#4989=CARTESIAN_POINT ( 'NONE',  ( 51.80576158887517835, -4.272136569073781587, 0.9439330974870294710 ) ) ;
#4993=ORIENTED_EDGE ( 'NONE', *, *, #1270, .F. ) ;
#4996=FACE_OUTER_BOUND ( 'NONE', #3448, .T. ) ;
#5003=DIRECTION ( 'NONE',  ( 1.000000000000000000, -0.000000000000000000, -0.000000000000000000 ) ) ;
#5006=ORIENTED_EDGE ( 'NONE', *, *, #9302, .F. ) ;
#5008=EDGE_CURVE ( 'NONE', #1696, #14148, #14947, .T. ) ;
#5011=CARTESIAN_POINT ( 'NONE',  ( 57.03577985506672832, 0.7479400494557524315, 1.780189605359982608 ) ) ;
#5020=CARTESIAN_POINT ( 'NONE',  ( 15.97944027357902819, -4.944296796129584948, -2.193698057025752490 ) ) ;
#5023=AXIS2_PLACEMENT_3D ( 'NONE', #15767, #10700, #22901 ) ;
#5025=CARTESIAN_POINT ( 'NONE',  ( -36.92362342067078629, -3.309998894527926172, -4.278958290368498396 ) ) ;
#5026=DIRECTION ( 'NONE',  ( 1.000000000000000000, 0.000000000000000000, 0.000000000000000000 ) ) ;
#5028=EDGE_LOOP ( 'NONE', ( #31262, #16063, #18258, #23587 ) ) ;
#5032=CARTESIAN_POINT ( 'NONE',  ( 15.61033468494287924, 0.4841707035674313042, -5.391286593723154219 ) ) ;
#5033=CARTESIAN_POINT ( 'NONE',  ( -36.58361892166016816, -5.109611055794880841, 1.772889539330528619 ) ) ;
#5036=ORIENTED_EDGE ( 'NONE', *, *, #350, .T. ) ;
#5038=CARTESIAN_POINT ( 'NONE',  ( 58.50000000000001421, -0.8000000000000000444, -2.421260002560649660 ) ) ;
#5041=AXIS2_PLACEMENT_3D ( 'NONE', #440, #12015, #19771 ) ;
#5043=AXIS2_PLACEMENT_3D ( 'NONE', #9381, #21753, #31233 ) ;
#5045=CARTESIAN_POINT ( 'NONE',  ( -54.49999999999997868, -1.549598385535858380, -4.064203588144675194 ) ) ;
#5056=ORIENTED_EDGE ( 'NONE', *, *, #5838, .T. ) ;
#5058=CARTESIAN_POINT ( 'NONE',  ( 15.57907767661756360, -3.590618801409561911, 4.051716037497246070 ) ) ;
#5059=( BOUNDED_SURFACE ( )  B_SPLINE_SURFACE ( 3, 2, ( 
 ( #12158, #21840, #31153 ),
 ( #14682, #24343, #5176 ),
 ( #21977, #7102, #269 ),
 ( #2174, #2794, #21516 ) ),
 .UNSPECIFIED., .F., .F., .F. ) 
 B_SPLINE_SURFACE_WITH_KNOTS ( ( 4, 4 ),
 ( 3, 3 ),
 ( 7.146054570217184225E-05, 0.0002313930902385299038 ),
 ( 0.000000000000000000, 1.000000000000000000 ),
 .UNSPECIFIED. ) 
 GEOMETRIC_REPRESENTATION_ITEM ( )  RATIONAL_B_SPLINE_SURFACE ( (
 ( 1.000000000000000000, 0.7071067811864972796, 1.000000000000000000),
 ( 1.000000000000000000, 0.6583912147046423469, 1.000000000000000000),
 ( 1.000000000000000000, 0.5850387677749523396, 1.000000000000000000),
 ( 1.000000000000000000, 0.5857791861290068125, 1.000000000000000000) ) ) 
 REPRESENTATION_ITEM ( '' )  SURFACE ( )  );
#5061=DIRECTION ( 'NONE',  ( 0.000000000000000000, 0.000000000000000000, -1.000000000000000000 ) ) ;
#5064=VECTOR ( 'NONE', #21462, 1000.000000000000000 ) ;
#5068=CARTESIAN_POINT ( 'NONE',  ( 50.38701762163459819, -1.088467210617550807, -3.899823238510139678 ) ) ;
#5070=B_SPLINE_CURVE_WITH_KNOTS ( 'NONE', 3,
 ( #5552, #8084, #10457, #5701, #5386, #27238, #22196, #15203, #24998, #2705, #7920, #480, #7617, #29443 ),
 .UNSPECIFIED., .F., .F.,
 ( 4, 2, 2, 2, 2, 2, 4 ),
 ( 0.000000000000000000, 2.506106230924540920E-05, 5.012212461849081840E-05, 0.0001002442492369731529, 0.0002004884984739371985, 0.0004009769969478685966, 0.0008019539938957305795 ),
 .UNSPECIFIED. ) ;
#5072=VERTEX_POINT ( 'NONE', #7999 ) ;
#5074=CARTESIAN_POINT ( 'NONE',  ( 15.44259799936805777, -2.880023619481785424, -4.335093843541868885 ) ) ;
#5086=CARTESIAN_POINT ( 'NONE',  ( -36.22955757456080050, -5.027944117024021331, -1.353132643598599305 ) ) ;
#5096=CARTESIAN_POINT ( 'NONE',  ( -54.49983832461118283, -1.542920080254279958, 3.327619142904489014 ) ) ;
#5099=CARTESIAN_POINT ( 'NONE',  ( 58.50000000000001421, -0.8000000000000000444, 2.421260002560649660 ) ) ;
#5100=CARTESIAN_POINT ( 'NONE',  ( -36.25997906085255096, -0.2181161761758297624, -5.200000001420975515 ) ) ;
#5103=CARTESIAN_POINT ( 'NONE',  ( 15.48609859788815690, 4.980680447166627722, -1.498595263773850661 ) ) ;
#5105=ORIENTED_EDGE ( 'NONE', *, *, #5434, .T. ) ;
#5109=CARTESIAN_POINT ( 'NONE',  ( 48.46185180831791683, -1.426738236278548566, 3.843750512866276559 ) ) ;
#5111=CARTESIAN_POINT ( 'NONE',  ( 58.45000000000001705, -0.8000000000000000444, -1.778341924377873751 ) ) ;
#5118=ORIENTED_EDGE ( 'NONE', *, *, #26851, .T. ) ;
#5125=CARTESIAN_POINT ( 'NONE',  ( 33.47623932017462778, -4.018128179617534101, -3.618665901676658692 ) ) ;
#5133=CARTESIAN_POINT ( 'NONE',  ( 57.00555950015162665, -0.7236022373656367801, 2.438089627148707805 ) ) ;
#5134=CARTESIAN_POINT ( 'NONE',  ( -36.56390771145571250, -3.345968172200375790, 4.250076229745575418 ) ) ;
#5141=ORIENTED_EDGE ( 'NONE', *, *, #24882, .F. ) ;
#5143=VERTEX_POINT ( 'NONE', #1782 ) ;
#5144=CIRCLE ( 'NONE', #26374, 0.4576450603546982632 ) ;
#5145=ADVANCED_FACE ( 'NONE', ( #6238 ), #30601, .T. ) ;
#5149=CARTESIAN_POINT ( 'NONE',  ( 15.03925126672132784, 4.683225679163323996, 2.703237727951258051 ) ) ;
#5150=CARTESIAN_POINT ( 'NONE',  ( -36.22909104983142470, 2.595074437874489437, 4.757608386864812466 ) ) ;
#5167=CARTESIAN_POINT ( 'NONE',  ( 50.30000000000001847, 1.391941090707540685, -3.850000000000022293 ) ) ;
#5168=EDGE_CURVE ( 'NONE', #26348, #1696, #3697, .T. ) ;
#5172=ADVANCED_FACE ( 'NONE', ( #27925 ), #11140, .T. ) ;
#5173=MANIFOLD_SOLID_BREP ( 'Stock-MAS-683-1', #14520 ) ;
#5176=CARTESIAN_POINT ( 'NONE',  ( 56.95000081403880188, -0.7675332364161941978, -2.484758330364432943 ) ) ;
#5177=CARTESIAN_POINT ( 'NONE',  ( -35.85663232820601820, -2.199885893005943061, -4.939696249117692339 ) ) ;
#5183=CARTESIAN_POINT ( 'NONE',  ( 48.30000000000003268, 0.7901969350670130510, 4.025772098418840983 ) ) ;
#5185=DIRECTION ( 'NONE',  ( 1.000000000000000000, 0.000000000000000000, -0.000000000000000000 ) ) ;
#5189=DIRECTION ( 'NONE',  ( -1.000000000000000000, -1.293068473084537258E-16, -0.000000000000000000 ) ) ;
#5194=CARTESIAN_POINT ( 'NONE',  ( 36.50000000000002132, -0.8000000000000000444, 1.778341924377873751 ) ) ;
#5200=CARTESIAN_POINT ( 'NONE',  ( 48.50000000000002132, 1.391941090707534023, 3.850000000000022737 ) ) ;
#5201=ORIENTED_EDGE ( 'NONE', *, *, #1082, .F. ) ;
#5202=B_SPLINE_CURVE_WITH_KNOTS ( 'NONE', 3,
 ( #23616, #28197, #11402, #9036, #1913, #11575, #21404, #31032, #12197, #16952, #5068, #19650, #7738, #24070 ),
 .UNSPECIFIED., .F., .F.,
 ( 4, 2, 2, 2, 2, 2, 4 ),
 ( 0.000000000000000000, 2.506106230924558877E-05, 5.012212461849117754E-05, 0.0001002442492369727192, 0.0002004884984739364396, 0.0004009769969478670787, 0.0008019539938957288448 ),
 .UNSPECIFIED. ) ;
#5204=FACE_OUTER_BOUND ( 'NONE', #27411, .T. ) ;
#5207=FACE_OUTER_BOUND ( 'NONE', #11250, .T. ) ;
#5212=FACE_OUTER_BOUND ( 'NONE', #19208, .T. ) ;
#5215=ORIENTED_EDGE ( 'NONE', *, *, #2584, .T. ) ;
#5216=DIRECTION ( 'NONE',  ( -1.000000000000000000, 0.000000000000000000, 0.000000000000000000 ) ) ;
#5220=FACE_OUTER_BOUND ( 'NONE', #30306, .T. ) ;
#5227=CARTESIAN_POINT ( 'NONE',  ( 51.77696287275522735, -4.162962223351915902, 1.036150832289953971 ) ) ;
#5229=CARTESIAN_POINT ( 'NONE',  ( -36.11122220296834229, -5.068511731019583522, -1.228278365481880297 ) ) ;
#5236=CARTESIAN_POINT ( 'NONE',  ( 48.30000000000002558, -0.6462379109120511833, -4.048750000000022276 ) ) ;
#5238=DIRECTION ( 'NONE',  ( 1.000000000000000000, -0.000000000000000000, -0.000000000000000000 ) ) ;
#5243=DIRECTION ( 'NONE',  ( 0.000000000000000000, -0.9333474217026306308, 0.3589743589743588648 ) ) ;
#5244=CARTESIAN_POINT ( 'NONE',  ( -36.11692583559979397, -1.123735554575807427, -5.289358692618237434 ) ) ;
#5245=ADVANCED_FACE ( 'NONE', ( #23821 ), #28728, .F. ) ;
#5251=CARTESIAN_POINT ( 'NONE',  ( -36.52679053911622731, -4.797009389500161092, -2.498041539401842925 ) ) ;
#5252=CARTESIAN_POINT ( 'NONE',  ( 15.74652664997094931, 3.008101665203244846, -4.495550615867462518 ) ) ;
#5253=DIRECTION ( 'NONE',  ( 1.520093157366863885E-16, -0.5877852522924685852, -0.8090169943749507819 ) ) ;
#5255=ORIENTED_EDGE ( 'NONE', *, *, #9238, .T. ) ;
#5257=EDGE_CURVE ( 'NONE', #25072, #30388, #20223, .T. ) ;
#5261=ORIENTED_EDGE ( 'NONE', *, *, #9015, .T. ) ;
#5266=DIRECTION ( 'NONE',  ( 0.000000000000000000, 1.000000000000000000, 0.000000000000000000 ) ) ;
#5269=CIRCLE ( 'NONE', #11856, 0.4576450603546999840 ) ;
#5273=VERTEX_POINT ( 'NONE', #29300 ) ;
#5275=DIRECTION ( 'NONE',  ( 0.000000000000000000, 0.000000000000000000, -1.000000000000000000 ) ) ;
#5277=DIRECTION ( 'NONE',  ( 1.000000000000000000, 0.000000000000000000, 0.000000000000000000 ) ) ;
#5278=CARTESIAN_POINT ( 'NONE',  ( 57.00500393873097238, 0.7225500701544015358, 2.438740121660158078 ) ) ;
#5280=CARTESIAN_POINT ( 'NONE',  ( -35.85663232820592583, -3.426725943139568020, 3.937891353488737423 ) ) ;
#5283=CARTESIAN_POINT ( 'NONE',  ( 51.80000000000001847, -3.726179070414207928, 1.100000000000000533 ) ) ;
#5286=ORIENTED_EDGE ( 'NONE', *, *, #22542, .F. ) ;
#5289=ORIENTED_EDGE ( 'NONE', *, *, #29184, .T. ) ;
#5294=EDGE_LOOP ( 'NONE', ( #8058, #30938, #15112, #14632, #18512 ) ) ;
#5298=ORIENTED_EDGE ( 'NONE', *, *, #3819, .T. ) ;
#5305=CARTESIAN_POINT ( 'NONE',  ( 15.29954477411456892, -4.683225668089734839, -2.703237747135711189 ) ) ;
#5313=CIRCLE ( 'NONE', #21536, 0.05000000000000002359 ) ;
#5323=EDGE_CURVE ( 'NONE', #9517, #9001, #15042, .T. ) ;
#5325=ORIENTED_EDGE ( 'NONE', *, *, #27536, .T. ) ;
#5327=CARTESIAN_POINT ( 'NONE',  ( 15.94709373951305054, 0.6031025731807972967, -5.374022845360688194 ) ) ;
#5328=CARTESIAN_POINT ( 'NONE',  ( -35.85663232820601820, -5.377732432866662471, 0.5657657256215425923 ) ) ;
#5339=CARTESIAN_POINT ( 'NONE',  ( 57.05000000000001847, -0.7794871794871796045, 1.732743413496389939 ) ) ;
#5340=EDGE_CURVE ( 'NONE', #7978, #6201, #24701, .T. ) ;
#5343=TOROIDAL_SURFACE ( 'NONE', #6368, 4.275000000000000355, 0.1000000000000000056 ) ;
#5349=ORIENTED_EDGE ( 'NONE', *, *, #16851, .T. ) ;
#5355=CARTESIAN_POINT ( 'NONE',  ( 15.66436536804550883, 2.847679722116457146, 4.601476325142709101 ) ) ;
#5358=B_SPLINE_CURVE_WITH_KNOTS ( 'NONE', 3,
 ( #2050, #23759, #16457, #11714, #9021, #18851, #18692, #11229, #9188, #16150, #4427, #16788, #21392, #7128, #28494, #25801, #9340, #30534, #21239 ),
 .UNSPECIFIED., .F., .F.,
 ( 4, 3, 3, 3, 3, 3, 4 ),
 ( 0.000000000000000000, 1.462084321540209121E-05, 2.917085440492037316E-05, 4.467649728434973632E-05, 6.285390091960512901E-05, 8.531547445983615763E-05, 8.677858956768834506E-05 ),
 .UNSPECIFIED. ) ;
#5371=UNCERTAINTY_MEASURE_WITH_UNIT (LENGTH_MEASURE( 1.000000000000000082E-05 ), #4761, 'distance_accuracy_value', 'NONE');
#5372=CARTESIAN_POINT ( 'NONE',  ( -54.44999999999997442, 0.000000000000000000, 0.000000000000000000 ) ) ;
#5373=CARTESIAN_POINT ( 'NONE',  ( 15.61552784268254079, -3.561547362098998359, -4.076645242318565288 ) ) ;
#5374=FACE_OUTER_BOUND ( 'NONE', #22304, .T. ) ;
#5375=DIRECTION ( 'NONE',  ( 0.000000000000000000, 0.000000000000000000, 1.000000000000000000 ) ) ;
#5376=AXIS2_PLACEMENT_3D ( 'NONE', #13041, #14937, #22723 ) ;
#5382=CARTESIAN_POINT ( 'NONE',  ( 34.50000000000001421, 0.000000000000000000, 0.000000000000000000 ) ) ;
#5386=CARTESIAN_POINT ( 'NONE',  ( 50.33046473658143327, 1.366509374015061784, 3.854674997130605352 ) ) ;
#5388=CARTESIAN_POINT ( 'NONE',  ( -36.38012252111052902, -5.369990034204360718, -0.6654225812206043811 ) ) ;
#5394=CIRCLE ( 'NONE', #24631, 0.05000000000000012768 ) ;
#5399=CIRCLE ( 'NONE', #4902, 2.649999999999999911 ) ;
#5400=CARTESIAN_POINT ( 'NONE',  ( 50.50000000000002842, 0.7900853852131533017, 4.025789903357282817 ) ) ;
#5402=CARTESIAN_POINT ( 'NONE',  ( -54.48833221701376317, -1.517896399908648553, 3.311598511234999265 ) ) ;
#5403=AXIS2_PLACEMENT_3D ( 'NONE', #10479, #22214, #3185 ) ;
#5404=CARTESIAN_POINT ( 'NONE',  ( 51.80000000000001137, -4.131056160354152240, -1.100000000000000533 ) ) ;
#5409=CARTESIAN_POINT ( 'NONE',  ( -36.42771574642738841, -0.4841707035675313908, -5.391286593723126686 ) ) ;
#5412=CARTESIAN_POINT ( 'NONE',  ( 48.45334018241208440, 1.329038565861465848, -3.861394075523872260 ) ) ;
#5413=CARTESIAN_POINT ( 'NONE',  ( 16.10705563471229596, 5.094475812726745545, -1.819860688632924939 ) ) ;
#5415=ORIENTED_EDGE ( 'NONE', *, *, #27375, .T. ) ;
#5417=CARTESIAN_POINT ( 'NONE',  ( -36.40793637698146057, -4.755763096844269455, -2.574151833883825624 ) ) ;
#5419=CARTESIAN_POINT ( 'NONE',  ( 15.56401610563845139, 2.291889356119606536, -4.901871067649723024 ) ) ;
#5424=CARTESIAN_POINT ( 'NONE',  ( 51.86913982414762359, 0.07429701114036996179, -4.369569592321115081 ) ) ;
#5425=CIRCLE ( 'NONE', #23133, 0.4576450603546982632 ) ;
#5428=CARTESIAN_POINT ( 'NONE',  ( 15.32766723174653833, -5.374753047227047276, 0.5963205376973673699 ) ) ;
#5429=VERTEX_POINT ( 'NONE', #15967 ) ;
#5430=ORIENTED_EDGE ( 'NONE', *, *, #10947, .F. ) ;
#5431=EDGE_CURVE ( 'NONE', #30058, #5273, #5528, .T. ) ;
#5432=CARTESIAN_POINT ( 'NONE',  ( 15.41586008885036563, 5.027926281937914688, 1.353187539902049430 ) ) ;
#5433=ORIENTED_EDGE ( 'NONE', *, *, #17085, .F. ) ;
#5434=EDGE_CURVE ( 'NONE', #24812, #9170, #24254, .T. ) ;
#5442=VECTOR ( 'NONE', #1305, 1000.000000000000000 ) ;
#5446=ORIENTED_EDGE ( 'NONE', *, *, #12639, .F. ) ;
#5452=CARTESIAN_POINT ( 'NONE',  ( 57.02888566337306031, -0.7456496514153734267, 2.424120212325347357 ) ) ;
#5459=CYLINDRICAL_SURFACE ( 'NONE', #18545, 0.04999999999999991257 ) ;
#5461=CYLINDRICAL_SURFACE ( 'NONE', #1065, 0.05000000000000143219 ) ;
#5469=CYLINDRICAL_SURFACE ( 'NONE', #21606, 0.1000000000000000472 ) ;
#5481=CARTESIAN_POINT ( 'NONE',  ( 15.41170998834774508, -5.326676561279859001, -0.9978806102896248253 ) ) ;
#5485=EDGE_CURVE ( 'NONE', #23938, #1800, #26785, .T. ) ;
#5486=CARTESIAN_POINT ( 'NONE',  ( 19.23646557533807666, -1.947877022684209034E-15, 0.000000000000000000 ) ) ;
#5488=CARTESIAN_POINT ( 'NONE',  ( -35.98952425903313213, -3.426725954212505698, -3.937891351789589489 ) ) ;
#5494=DIRECTION ( 'NONE',  ( 1.000000000000000000, 0.000000000000000000, 0.000000000000000000 ) ) ;
#5495=EDGE_CURVE ( 'NONE', #7645, #518, #29307, .T. ) ;
#5508=DIRECTION ( 'NONE',  ( -1.000000000000000000, 0.000000000000000000, 0.000000000000000000 ) ) ;
#5510=CARTESIAN_POINT ( 'NONE',  ( -35.85663232820584057, -5.086913985776159386, 1.171642053949095930 ) ) ;
#5512=CARTESIAN_POINT ( 'NONE',  ( 46.90000000000001279, -4.131056160354152240, -1.100000000000000089 ) ) ;
#5519=CARTESIAN_POINT ( 'NONE',  ( -44.49999999999999289, -1.499999999999999556, 4.029888335921975262 ) ) ;
#5523=ORIENTED_EDGE ( 'NONE', *, *, #10430, .T. ) ;
#5525=CARTESIAN_POINT ( 'NONE',  ( 15.95705409078441583, 3.646557212684218729, 3.995389720703451886 ) ) ;
#5528=CIRCLE ( 'NONE', #25256, 0.09999999999999982514 ) ;
#5529=CARTESIAN_POINT ( 'NONE',  ( 54.50000000000002132, 0.000000000000000000, -3.299999999999999822 ) ) ;
#5534=EDGE_LOOP ( 'NONE', ( #18806, #3559, #3813, #17504 ) ) ;
#5541=CARTESIAN_POINT ( 'NONE',  ( -35.85663232820584057, -2.199885893005943949, -4.939696249117691451 ) ) ;
#5542=ORIENTED_EDGE ( 'NONE', *, *, #18455, .T. ) ;
#5543=EDGE_LOOP ( 'NONE', ( #28133, #15373, #7472, #9372 ) ) ;
#5548=ORIENTED_EDGE ( 'NONE', *, *, #10667, .F. ) ;
#5552=CARTESIAN_POINT ( 'NONE',  ( 50.30000000000001847, 1.391941090707534023, 3.850000000000022737 ) ) ;
#5555=PRODUCT_CONTEXT ( 'NONE', #2661, 'mechanical' ) ;
#5557=( BOUNDED_SURFACE ( )  B_SPLINE_SURFACE ( 3, 2, ( 
 ( #26939, #12532, #24416 ),
 ( #22058, #21914, #12682 ),
 ( #24725, #24872, #24562 ),
 ( #19981, #22362, #354 ) ),
 .UNSPECIFIED., .F., .F., .F. ) 
 B_SPLINE_SURFACE_WITH_KNOTS ( ( 4, 4 ),
 ( 3, 3 ),
 ( 6.470519842244164266E-05, 0.0002246728259156070709 ),
 ( 0.000000000000000000, 1.000000000000000000 ),
 .UNSPECIFIED. ) 
 GEOMETRIC_REPRESENTATION_ITEM ( )  RATIONAL_B_SPLINE_SURFACE ( (
 ( 1.000000000000000000, 0.5857791861290068125, 1.000000000000000000),
 ( 1.000000000000000000, 0.5849685391560944803, 1.000000000000000000),
 ( 1.000000000000000000, 0.6585504321673580908, 1.000000000000000000),
 ( 1.000000000000000000, 0.7071067811864985009, 1.000000000000000000) ) ) 
 REPRESENTATION_ITEM ( '' )  SURFACE ( )  );
#5561=AXIS2_PLACEMENT_3D ( 'NONE', #2715, #9705, #4621 ) ;
#5564=CARTESIAN_POINT ( 'NONE',  ( 48.45124641917420405, -1.383300983803864570, -3.859740869727656953 ) ) ;
#5565=CARTESIAN_POINT ( 'NONE',  ( 15.48686146417450082, 0.1108756495953548971, 5.200000001674996319 ) ) ;
#5574=DIRECTION ( 'NONE',  ( -0.000000000000000000, -0.000000000000000000, 1.000000000000000000 ) ) ;
#5578=CARTESIAN_POINT ( 'NONE',  ( 50.41047473690879599, -0.7808213810458148885, -4.027268569371626583 ) ) ;
#5581=CARTESIAN_POINT ( 'NONE',  ( 15.03925126672127810, 3.426725943139600439, -3.937891353488703228 ) ) ;
#5586=CARTESIAN_POINT ( 'NONE',  ( 51.80000000000001847, -4.259181259350203419, 1.099999999999999645 ) ) ;
#5590=EDGE_LOOP ( 'NONE', ( #4181, #8795, #9087, #23539, #1837 ) ) ;
#5592=EDGE_CURVE ( 'NONE', #13616, #24615, #28644, .T. ) ;
#5607=DIRECTION ( 'NONE',  ( 0.000000000000000000, 0.000000000000000000, -1.000000000000000000 ) ) ;
#5612=CARTESIAN_POINT ( 'NONE',  ( 50.42215036618306812, -1.308847734660468332, -3.885629509820973659 ) ) ;
#5615=CARTESIAN_POINT ( 'NONE',  ( -54.49983832461118283, 1.542920080254278181, -3.327619142904491234 ) ) ;
#5618=ORIENTED_EDGE ( 'NONE', *, *, #26820, .F. ) ;
#5619=CARTESIAN_POINT ( 'NONE',  ( -54.47754877553799702, 1.508273929415538062, 3.305418158118663907 ) ) ;
#5620=ORIENTED_EDGE ( 'NONE', *, *, #16543, .T. ) ;
#5635=CARTESIAN_POINT ( 'NONE',  ( 16.07279755198655380, -5.034707333629182990, -1.977875755500475563 ) ) ;
#5641=CARTESIAN_POINT ( 'NONE',  ( 50.34875358082582864, 1.383300983803910089, -3.859740869727648072 ) ) ;
#5643=ADVANCED_FACE ( 'NONE', ( #25791 ), #4099, .F. ) ;
#5649=CARTESIAN_POINT ( 'NONE',  ( -36.27260443516964017, -3.212533369474692257, -4.093511368021621522 ) ) ;
#5652=DIRECTION ( 'NONE',  ( 1.000000000000000000, 2.586136946169074517E-16, -0.000000000000000000 ) ) ;
#5656=CARTESIAN_POINT ( 'NONE',  ( 48.33022520384532328, -1.142230555601074116, -3.938343097974785767 ) ) ;
#5658=ORIENTED_EDGE ( 'NONE', *, *, #21538, .F. ) ;
#5662=DIRECTION ( 'NONE',  ( -1.000000000000000000, -0.000000000000000000, -0.000000000000000000 ) ) ;
#5667=CARTESIAN_POINT ( 'NONE',  ( 56.95000000000001705, 0.000000000000000000, 0.000000000000000000 ) ) ;
#5670=CIRCLE ( 'NONE', #27905, 2.549999999999999822 ) ;
#5673=LINE ( 'NONE', #5519, #13169 ) ;
#5674=DIRECTION ( 'NONE',  ( 0.000000000000000000, 0.000000000000000000, -1.000000000000000000 ) ) ;
#5675=ORIENTED_EDGE ( 'NONE', *, *, #15556, .F. ) ;
#5676=CARTESIAN_POINT ( 'NONE',  ( 15.41080140630217343, 2.595266697484422291, 4.757426534476680402 ) ) ;
#5681=EDGE_CURVE ( 'NONE', #6673, #13582, #7970, .T. ) ;
#5683=CARTESIAN_POINT ( 'NONE',  ( -36.38012252111052902, 1.026563698233470268, 5.312790900508079339 ) ) ;
#5684=CARTESIAN_POINT ( 'NONE',  ( 48.37840743871460347, 1.310166284604407760, -3.885185101012171849 ) ) ;
#5689=CARTESIAN_POINT ( 'NONE',  ( 50.40746642207054151, -1.341874354110735634, 3.874311046529113511 ) ) ;
#5690=CARTESIAN_POINT ( 'NONE',  ( 15.41170998834775041, -3.722832355336850529, -3.938244298533932319 ) ) ;
#5695=ADVANCED_FACE ( 'NONE', ( #29554 ), #29699, .T. ) ;
#5699=CARTESIAN_POINT ( 'NONE',  ( 51.74134002894188455, -4.175606900721715142, 1.008275291528680562 ) ) ;
#5701=CARTESIAN_POINT ( 'NONE',  ( 50.32627973729707094, 1.373706569044511605, 3.853361913240786585 ) ) ;
#5706=EDGE_CURVE ( 'NONE', #26067, #26007, #895, .T. ) ;
#5708=DIRECTION ( 'NONE',  ( 0.000000000000000000, 1.000000000000000000, 0.000000000000000000 ) ) ;
#5711=CARTESIAN_POINT ( 'NONE',  ( 15.76623786017542272, -0.1071614981651040632, 5.407381887150171984 ) ) ;
#5715=CARTESIAN_POINT ( 'NONE',  ( -35.85663232820596136, 0.7747498368337510932, -5.363501452440939232 ) ) ;
#5716=EDGE_CURVE ( 'NONE', #9190, #23361, #26670, .T. ) ;
#5717=AXIS2_PLACEMENT_3D ( 'NONE', #15843, #4125, #13761 ) ;
#5718=EDGE_CURVE ( 'NONE', #16074, #5072, #27173, .T. ) ;
#5724=CARTESIAN_POINT ( 'NONE',  ( 50.31907412294955861, -1.391939743175890420, -3.849999999996903899 ) ) ;
#5725=CARTESIAN_POINT ( 'NONE',  ( -36.00197790576392265, 4.018128179617553641, -3.618665901676621388 ) ) ;
#5726=CARTESIAN_POINT ( 'NONE',  ( 15.29384114148379759, 3.378548217643521756, -3.972894518062563662 ) ) ;
#5728=CARTESIAN_POINT ( 'NONE',  ( 15.03925126672132961, 3.275050215668553921, 2.949461045527632219 ) ) ;
#5731=CARTESIAN_POINT ( 'NONE',  ( -54.49999999999997868, 1.734723475976807094E-15, -4.375000000000000000 ) ) ;
#5732=ADVANCED_FACE ( 'NONE', ( #7718 ), #24666, .T. ) ;
#5734=EDGE_LOOP ( 'NONE', ( #9256, #29772, #27898, #15881 ) ) ;
#5735=CARTESIAN_POINT ( 'NONE',  ( 15.70940947763171280, -4.797009389500164644, 2.498041539401808731 ) ) ;
#5738=CARTESIAN_POINT ( 'NONE',  ( 15.03925126672132606, 5.340403872473315161, 0.9205822173396651653 ) ) ;
#5750=EDGE_LOOP ( 'NONE', ( #22041, #3805, #23300, #4258 ) ) ;
#5752=PLANE ( 'NONE',  #15497 ) ;
#5755=CARTESIAN_POINT ( 'NONE',  ( 58.45000000000001705, -0.7500000000000000000, 1.778341924377873751 ) ) ;
#5756=EDGE_CURVE ( 'NONE', #11417, #9170, #374, .T. ) ;
#5760=EDGE_CURVE ( 'NONE', #3125, #1800, #26161, .T. ) ;
#5766=TOROIDAL_SURFACE ( 'NONE', #10801, 14.70000000000000995, 10.00000000000000000 ) ;
#5780=CARTESIAN_POINT ( 'NONE',  ( 48.40000000000001990, -1.409787217987148233, -3.950000000000022826 ) ) ;
#5785=CARTESIAN_POINT ( 'NONE',  ( 48.40000000000001990, 2.428612866367529932E-14, 0.000000000000000000 ) ) ;
#5787=CARTESIAN_POINT ( 'NONE',  ( 16.10624235918718128, -5.092377074781565760, -1.825725187625025780 ) ) ;
#5789=TOROIDAL_SURFACE ( 'NONE', #3747, 4.284222560975607053, 0.1000000000000000056 ) ;
#5794=DIRECTION ( 'NONE',  ( 0.000000000000000000, -0.1576190026614809614, 0.9875000000000001554 ) ) ;
#5809=ORIENTED_EDGE ( 'NONE', *, *, #13059, .T. ) ;
#5812=DIRECTION ( 'NONE',  ( 0.000000000000000000, -0.000000000000000000, -1.000000000000000000 ) ) ;
#5826=EDGE_CURVE ( 'NONE', #14710, #1490, #12172, .T. ) ;
#5828=EDGE_CURVE ( 'NONE', #12135, #20165, #22653, .T. ) ;
#5829=CARTESIAN_POINT ( 'NONE',  ( -36.81959771849335539, -3.629052419422241993, 4.014440194077206314 ) ) ;
#5830=DIRECTION ( 'NONE',  ( 1.000000000000000000, 0.000000000000000000, 0.000000000000000000 ) ) ;
#5834=CARTESIAN_POINT ( 'NONE',  ( 15.48686146417447951, -2.966783028120464127, 4.272059443775220622 ) ) ;
#5835=ORIENTED_EDGE ( 'NONE', *, *, #9587, .T. ) ;
#5837=DIRECTION ( 'NONE',  ( 1.000000000000000000, 0.000000000000000000, 0.000000000000000000 ) ) ;
#5838=EDGE_CURVE ( 'NONE', #8004, #6093, #14107, .T. ) ;
#5847=DIRECTION ( 'NONE',  ( 0.000000000000000000, -0.9615843008030765526, -0.2745098039215693730 ) ) ;
#5849=AXIS2_PLACEMENT_3D ( 'NONE', #8976, #6285, #18019 ) ;
#5853=DIRECTION ( 'NONE',  ( 1.000000000000000000, 0.000000000000000000, 0.000000000000000000 ) ) ;
#5854=CIRCLE ( 'NONE', #24535, 0.05000000000000012768 ) ;
#5855=CARTESIAN_POINT ( 'NONE',  ( 48.50000000000002132, -1.391941090707485396, 3.750000000000022649 ) ) ;
#5864=ADVANCED_FACE ( 'NONE', ( #13092 ), #10575, .F. ) ;
#5870=CARTESIAN_POINT ( 'NONE',  ( 47.01551613116910744, -4.158727452193214269, -1.045216533296355887 ) ) ;
#5872=CARTESIAN_POINT ( 'NONE',  ( 48.38950019258942348, -0.7811435014052807713, -4.027217152859519089 ) ) ;
#5875=VECTOR ( 'NONE', #6536, 1000.000000000000000 ) ;
#5879=CARTESIAN_POINT ( 'NONE',  ( 56.95000000000001705, 0.000000000000000000, 0.000000000000000000 ) ) ;
#5883=VECTOR ( 'NONE', #1860, 1000.000000000000000 ) ;
#5889=( BOUNDED_SURFACE ( )  B_SPLINE_SURFACE ( 3, 2, ( 
 ( #28453, #13859, #28921 ),
 ( #25916, #23719, #2489 ),
 ( #16896, #21822, #28774 ),
 ( #18965, #26391, #4219 ) ),
 .UNSPECIFIED., .F., .F., .F. ) 
 B_SPLINE_SURFACE_WITH_KNOTS ( ( 4, 4 ),
 ( 3, 3 ),
 ( 7.500129584393919939E-05, 0.0002378367988924469107 ),
 ( 0.000000000000000000, 1.000000000000000000 ),
 .UNSPECIFIED. ) 
 GEOMETRIC_REPRESENTATION_ITEM ( )  RATIONAL_B_SPLINE_SURFACE ( (
 ( 1.000000000000000000, 0.7071067811864996111, 1.000000000000000000),
 ( 1.000000000000000000, 0.7717803178830575650, 1.000000000000000000),
 ( 1.000000000000000000, 0.8407248428044677979, 1.000000000000000000),
 ( 1.000000000000000000, 0.8397191227596303431, 1.000000000000000000) ) ) 
 REPRESENTATION_ITEM ( '' )  SURFACE ( )  );
#5891=CARTESIAN_POINT ( 'NONE',  ( 16.07279755198654314, 3.436881753486524360, -4.177093996075191384 ) ) ;
#5894=ORIENTED_EDGE ( 'NONE', *, *, #31020, .T. ) ;
#5897=VERTEX_POINT ( 'NONE', #23080 ) ;
#5914=ORIENTED_EDGE ( 'NONE', *, *, #25882, .F. ) ;
#5917=AXIS2_PLACEMENT_3D ( 'NONE', #6225, #18127, #30284 ) ;
#5921=CARTESIAN_POINT ( 'NONE',  ( 56.95766603241608550, -0.7209790597604740503, -1.757928312873409116 ) ) ;
#5922=DIRECTION ( 'NONE',  ( 1.000000000000000000, -0.000000000000000000, -0.000000000000000000 ) ) ;
#5927=DIRECTION ( 'NONE',  ( 0.000000000000000000, 0.000000000000000000, -1.000000000000000000 ) ) ;
#5931=AXIS2_PLACEMENT_3D ( 'NONE', #5111, #12539, #22369 ) ;
#5934=CARTESIAN_POINT ( 'NONE',  ( 50.42115343657336268, -0.9200365198983494475, 3.998286360709618403 ) ) ;
#5939=ORIENTED_EDGE ( 'NONE', *, *, #30955, .T. ) ;
#5945=DIRECTION ( 'NONE',  ( 0.000000000000000000, 0.000000000000000000, 1.000000000000000000 ) ) ;
#5948=CARTESIAN_POINT ( 'NONE',  ( 34.50000000000001421, 0.000000000000000000, 0.000000000000000000 ) ) ;
#5960=AXIS2_PLACEMENT_3D ( 'NONE', #17340, #17664, #22410 ) ;
#5967=CARTESIAN_POINT ( 'NONE',  ( 48.49162684147595570, 1.391941090707552897, 3.850000000000020517 ) ) ;
#5975=AXIS2_PLACEMENT_3D ( 'NONE', #18425, #6228, #8599 ) ;
#5976=EDGE_CURVE ( 'NONE', #9170, #2253, #12771, .T. ) ;
#5978=FACE_OUTER_BOUND ( 'NONE', #12545, .T. ) ;
#5982=CIRCLE ( 'NONE', #26124, 4.384222560975607585 ) ;
#5985=CARTESIAN_POINT ( 'NONE',  ( 15.03925126672132961, -0.4576450603546909357, -5.200000000000000178 ) ) ;
#5994=DIRECTION ( 'NONE',  ( 0.000000000000000000, 1.000000000000000000, 0.000000000000000000 ) ) ;
#5997=CARTESIAN_POINT ( 'NONE',  ( -36.04581030752768100, 5.340403874104499238, -0.9205822090004349700 ) ) ;
#6005=CARTESIAN_POINT ( 'NONE',  ( 15.76675455518197211, 3.261791109367046637, 4.314133646218528462 ) ) ;
#6012=FACE_OUTER_BOUND ( 'NONE', #25519, .T. ) ;
#6021=CARTESIAN_POINT ( 'NONE',  ( 47.00000000000002132, -3.726179070414207928, -1.000000000000002220 ) ) ;
#6028=ORIENTED_EDGE ( 'NONE', *, *, #19116, .F. ) ;
#6032=CARTESIAN_POINT ( 'NONE',  ( 36.50000000000002132, 0.000000000000000000, -1.899999999999999911 ) ) ;
#6039=LINE ( 'NONE', #18699, #6071 ) ;
#6041=CARTESIAN_POINT ( 'NONE',  ( 15.56401610563845850, 1.027070083876111761, 5.312835761376648591 ) ) ;
#6052=CARTESIAN_POINT ( 'NONE',  ( 50.42159256128543632, -1.310166284604358244, -3.885185101012172737 ) ) ;
#6056=CARTESIAN_POINT ( 'NONE',  ( 56.99370871690835116, 0.8156862421929632623, 2.468735699563065378 ) ) ;
#6057=ORIENTED_EDGE ( 'NONE', *, *, #6217, .F. ) ;
#6064=CYLINDRICAL_SURFACE ( 'NONE', #26918, 4.100000000000022737 ) ;
#6071=VECTOR ( 'NONE', #23137, 1000.000000000000000 ) ;
#6073=ORIENTED_EDGE ( 'NONE', *, *, #17877, .T. ) ;
#6074=VECTOR ( 'NONE', #31087, 1000.000000000000000 ) ;
#6078=CARTESIAN_POINT ( 'NONE',  ( 56.98297952491088836, -0.7550874052942159187, -1.743526814789472912 ) ) ;
#6084=EDGE_CURVE ( 'NONE', #20395, #2624, #7450, .T. ) ;
#6086=CARTESIAN_POINT ( 'NONE',  ( 48.39188949082539892, -1.340787288841403635, 3.874691554877328858 ) ) ;
#6088=ADVANCED_FACE ( 'NONE', ( #30823 ), #14544, .T. ) ;
#6090=CARTESIAN_POINT ( 'NONE',  ( -36.92398358572908279, 0.2875137064281962362, -5.407399902318745788 ) ) ;
#6093=VERTEX_POINT ( 'NONE', #18486 ) ;
#6098=ORIENTED_EDGE ( 'NONE', *, *, #16848, .F. ) ;
#6110=CARTESIAN_POINT ( 'NONE',  ( 15.03925126672132961, -1.123735532908273216, 5.289358697221548944 ) ) ;
#6115=AXIS2_PLACEMENT_3D ( 'NONE', #8273, #17940, #23285 ) ;
#6118=CARTESIAN_POINT ( 'NONE',  ( 47.04142135623732912, -3.767600426651517065, 1.000000000000000222 ) ) ;
#6121=EDGE_CURVE ( 'NONE', #8161, #1297, #19626, .T. ) ;
#6124=ORIENTED_EDGE ( 'NONE', *, *, #21538, .T. ) ;
#6130=CARTESIAN_POINT ( 'NONE',  ( 15.17256654081424472, -0.4576450652446781842, -5.200000002521312226 ) ) ;
#6139=CARTESIAN_POINT ( 'NONE',  ( 50.29999999999740368, 1.409901620923733390, 3.849999999997240518 ) ) ;
#6140=DIRECTION ( 'NONE',  ( 1.000000000000000000, 2.586136946169074517E-16, -0.000000000000000000 ) ) ;
#6143=CARTESIAN_POINT ( 'NONE',  ( -36.48821680285229263, 5.256402525810011994, -1.287848407636733139 ) ) ;
#6149=ORIENTED_EDGE ( 'NONE', *, *, #20855, .F. ) ;
#6151=CIRCLE ( 'NONE', #23852, 0.7500000000000186517 ) ;
#6153=CARTESIAN_POINT ( 'NONE',  ( 33.47623932017462778, -4.374999999999999112, 0.000000000000000000 ) ) ;
#6156=CARTESIAN_POINT ( 'NONE',  ( 51.87987261549070439, -4.254270342444942621, 1.021450466989924477 ) ) ;
#6160=DIRECTION ( 'NONE',  ( 1.000000000000000000, 2.586136946169074517E-16, -0.000000000000000000 ) ) ;
#6164=CARTESIAN_POINT ( 'NONE',  ( 48.50000000000002132, -4.899999999999999467, -3.950000000000022826 ) ) ;
#6169=ORIENTED_EDGE ( 'NONE', *, *, #26088, .F. ) ;
#6171=CARTESIAN_POINT ( 'NONE',  ( 54.40000000000001990, -0.2842225609755594795, -1.577752156565102655E-15 ) ) ;
#6176=FACE_OUTER_BOUND ( 'NONE', #28367, .T. ) ;
#6188=CARTESIAN_POINT ( 'NONE',  ( 15.03925126672132784, 0.7747498368337703001, 5.363501452440938344 ) ) ;
#6189=LINE ( 'NONE', #20151, #2384 ) ;
#6191=DIRECTION ( 'NONE',  ( 0.000000000000000000, 0.000000000000000000, -1.000000000000000000 ) ) ;
#6193=ORIENTED_EDGE ( 'NONE', *, *, #4275, .T. ) ;
#6196=CARTESIAN_POINT ( 'NONE',  ( -35.85663232820584057, 4.018128179617551865, -3.618665901676622720 ) ) ;
#6198=LINE ( 'NONE', #16326, #24605 ) ;
#6200=CARTESIAN_POINT ( 'NONE',  ( 15.03925126672127988, -5.086913985776152280, 1.171642053949085494 ) ) ;
#6201=VERTEX_POINT ( 'NONE', #7381 ) ;
#6203=CARTESIAN_POINT ( 'NONE',  ( 47.04714695228949495, -4.172892586174061336, 1.014428651009327442 ) ) ;
#6205=B_SPLINE_CURVE_WITH_KNOTS ( 'NONE', 3,
 ( #2, #20063, #9669, #27326, #8018, #27473 ),
 .UNSPECIFIED., .F., .F.,
 ( 4, 2, 4 ),
 ( 0.000000000000000000, 0.0001614717865051737596, 0.0003229435730103475191 ),
 .UNSPECIFIED. ) ;
#6213=CARTESIAN_POINT ( 'NONE',  ( -54.44999999999997442, 2.818925648462311528E-15, 9.856100559121352825E-17 ) ) ;
#6216=ORIENTED_EDGE ( 'NONE', *, *, #19892, .F. ) ;
#6217=EDGE_CURVE ( 'NONE', #25275, #10297, #26992, .T. ) ;
#6225=CARTESIAN_POINT ( 'NONE',  ( 17.21035195517769267, -2.471857751707523654E-15, 0.000000000000000000 ) ) ;
#6226=CARTESIAN_POINT ( 'NONE',  ( 47.00000000000002132, 1.734723475976807094E-15, 0.000000000000000000 ) ) ;
#6228=DIRECTION ( 'NONE',  ( -1.000000000000000000, -0.000000000000000000, -0.000000000000000000 ) ) ;
#6229=DIRECTION ( 'NONE',  ( -0.000000000000000000, 8.673617379884032317E-15, 1.000000000000000000 ) ) ;
#6232=DIRECTION ( 'NONE',  ( 0.000000000000000000, 0.000000000000000000, 1.000000000000000000 ) ) ;
#6238=FACE_OUTER_BOUND ( 'NONE', #23691, .T. ) ;
#6246=ORIENTED_EDGE ( 'NONE', *, *, #2171, .F. ) ;
#6249=DIRECTION ( 'NONE',  ( -1.000000000000000000, -4.939082069373669245E-17, 1.520093157366878429E-16 ) ) ;
#6256=CARTESIAN_POINT ( 'NONE',  ( 47.00000000000002842, -4.131056160354152240, -1.099999999999999867 ) ) ;
#6260=CARTESIAN_POINT ( 'NONE',  ( 15.32766723174653123, 2.228024565339362439, 4.927420728799238425 ) ) ;
#6266=CARTESIAN_POINT ( 'NONE',  ( 51.80000000000001137, -4.131056160354152240, 1.099999999999999423 ) ) ;
#6267=DIRECTION ( 'NONE',  ( -2.085103575917242148E-15, -0.9615843008030771077, 0.2745098039215673746 ) ) ;
#6279=ORIENTED_EDGE ( 'NONE', *, *, #10194, .T. ) ;
#6283=DIRECTION ( 'NONE',  ( 1.000000000000000000, 0.000000000000000000, 0.000000000000000000 ) ) ;
#6285=DIRECTION ( 'NONE',  ( -1.520093157366894206E-16, 0.5877852522924802425, -0.8090169943749422332 ) ) ;
#6294=AXIS2_PLACEMENT_3D ( 'NONE', #16937, #24055, #24676 ) ;
#6302=DIRECTION ( 'NONE',  ( 0.000000000000000000, 0.000000000000000000, -1.000000000000000000 ) ) ;
#6305=ORIENTED_EDGE ( 'NONE', *, *, #1277, .T. ) ;
#6308=AXIS2_PLACEMENT_3D ( 'NONE', #22996, #10949, #20637 ) ;
#6310=CARTESIAN_POINT ( 'NONE',  ( 48.33046193264123502, 1.143620537822834349, 3.937943076466140724 ) ) ;
#6321=CARTESIAN_POINT ( 'NONE',  ( -36.40793637698146767, 2.334444681449654446, 4.877899991435294957 ) ) ;
#6339=DIRECTION ( 'NONE',  ( -1.000000000000000000, -2.586136946169074517E-16, 0.000000000000000000 ) ) ;
#6341=VECTOR ( 'NONE', #25701, 1000.000000000000000 ) ;
#6344=DIRECTION ( 'NONE',  ( 0.000000000000000000, 0.000000000000000000, 1.000000000000000000 ) ) ;
#6348=EDGE_CURVE ( 'NONE', #23319, #20985, #19245, .T. ) ;
#6351=DIRECTION ( 'NONE',  ( 1.000000000000000000, 2.586136946169074517E-16, -0.000000000000000000 ) ) ;
#6356=EDGE_LOOP ( 'NONE', ( #15149, #7411, #7301, #24469, #14305, #8492, #28636, #19032, #5835 ) ) ;
#6357=DIRECTION ( 'NONE',  ( -1.000000000000000000, -0.000000000000000000, -0.000000000000000000 ) ) ;
#6358=CYLINDRICAL_SURFACE ( 'NONE', #22070, 0.04999999999999991257 ) ;
#6365=EDGE_CURVE ( 'NONE', #19303, #3444, #8158, .T. ) ;
#6368=AXIS2_PLACEMENT_3D ( 'NONE', #2872, #22045, #7315 ) ;
#6370=CARTESIAN_POINT ( 'NONE',  ( 56.96117471280891209, -0.7619384116854249767, 2.485869561276773165 ) ) ;
#6373=LINE ( 'NONE', #16036, #5875 ) ;
#6375=CARTESIAN_POINT ( 'NONE',  ( 57.04707324256202128, 0.7500000000000492939, 2.421260002560643443 ) ) ;
#6380=CARTESIAN_POINT ( 'NONE',  ( -36.40878371307407946, 4.755985070912289281, -2.573747172434650121 ) ) ;
#6387=CARTESIAN_POINT ( 'NONE',  ( 47.00000000000002132, -3.726179070414207928, 1.100000000000000311 ) ) ;
#6389=CIRCLE ( 'NONE', #24097, 4.299999999999998046 ) ;
#6390=CARTESIAN_POINT ( 'NONE',  ( -35.85663232820584057, -1.123735532908306523, -5.289358697221545391 ) ) ;
#6394=EDGE_CURVE ( 'NONE', #2692, #24817, #21254, .T. ) ;
#6422=CIRCLE ( 'NONE', #18075, 0.09999999999999997780 ) ;
#6426=CARTESIAN_POINT ( 'NONE',  ( -36.22955757456062287, -2.840625797033914157, 4.363718033548201092 ) ) ;
#6429=CIRCLE ( 'NONE', #18577, 1.000000000000000000 ) ;
#6430=CARTESIAN_POINT ( 'NONE',  ( 51.80000000000001137, -4.227689052994008101, 1.125730994152044362 ) ) ;
#6446=ORIENTED_EDGE ( 'NONE', *, *, #3672, .T. ) ;
#6448=AXIS2_PLACEMENT_3D ( 'NONE', #19119, #31288, #26225 ) ;
#6450=AXIS2_PLACEMENT_3D ( 'NONE', #22988, #20631, #27418 ) ;
#6453=CARTESIAN_POINT ( 'NONE',  ( -41.12388279035661753, 5.147405183146855023, 0.000000000000000000 ) ) ;
#6456=DIRECTION ( 'NONE',  ( 0.000000000000000000, 0.000000000000000000, 1.000000000000000000 ) ) ;
#6467=AXIS2_PLACEMENT_3D ( 'NONE', #21315, #16711, #2122 ) ;
#6471=LINE ( 'NONE', #16128, #19540 ) ;
#6473=CARTESIAN_POINT ( 'NONE',  ( 48.40000000000002700, 0.6462379109121004772, -4.048750000000028493 ) ) ;
#6478=CARTESIAN_POINT ( 'NONE',  ( 48.46244267249164039, 1.426738769040801769, 3.843750315111145621 ) ) ;
#6479=CARTESIAN_POINT ( 'NONE',  ( 58.45000000000001705, 0.000000000000000000, 0.000000000000000000 ) ) ;
#6483=CARTESIAN_POINT ( 'NONE',  ( 58.45000000000001705, -0.7500000000000000000, -1.778341924377873751 ) ) ;
#6487=CARTESIAN_POINT ( 'NONE',  ( -36.79682133506352670, 3.614202567155919255, 4.024415706308089646 ) ) ;
#6488=CIRCLE ( 'NONE', #20140, 0.05000000000000012768 ) ;
#6491=CARTESIAN_POINT ( 'NONE',  ( 51.90000000000001279, -1.084202172485504434E-16, 4.374999999999999112 ) ) ;
#6499=EDGE_CURVE ( 'NONE', #8955, #25147, #11002, .T. ) ;
#6500=CARTESIAN_POINT ( 'NONE',  ( 15.59055531549694074, -0.9785522574021975339, -5.318456145981289573 ) ) ;
#6501=CARTESIAN_POINT ( 'NONE',  ( 33.47623932017462778, 2.199885893005919968, 4.939696249117695892 ) ) ;
#6502=FACE_OUTER_BOUND ( 'NONE', #694, .T. ) ;
#6503=AXIS2_PLACEMENT_3D ( 'NONE', #28358, #11579, #14097 ) ;
#6505=DIRECTION ( 'NONE',  ( -1.000000000000000000, -0.000000000000000000, -0.000000000000000000 ) ) ;
#6507=VERTEX_POINT ( 'NONE', #25551 ) ;
#6509=EDGE_CURVE ( 'NONE', #30058, #6673, #14082, .T. ) ;
#6512=CARTESIAN_POINT ( 'NONE',  ( 15.03925126672132961, 1.793057972834757541, 4.026191436120407197 ) ) ;
#6516=ADVANCED_FACE ( 'NONE', ( #21784 ), #17016, .F. ) ;
#6517=ORIENTED_EDGE ( 'NONE', *, *, #13276, .T. ) ;
#6524=ORIENTED_EDGE ( 'NONE', *, *, #14724, .T. ) ;
#6526=EDGE_CURVE ( 'NONE', #11900, #16762, #4970, .T. ) ;
#6530=ORIENTED_EDGE ( 'NONE', *, *, #9032, .T. ) ;
#6531=EDGE_LOOP ( 'NONE', ( #5201, #2281, #21691, #24953 ) ) ;
#6532=AXIS2_PLACEMENT_3D ( 'NONE', #2555, #623, #10283 ) ;
#6536=DIRECTION ( 'NONE',  ( 1.000000000000000000, -0.000000000000000000, -0.000000000000000000 ) ) ;
#6539=EDGE_CURVE ( 'NONE', #6201, #6507, #21456, .T. ) ;
#6540=CARTESIAN_POINT ( 'NONE',  ( -36.72207054450174724, 4.892019442464198953, -2.306425897665967728 ) ) ;
#6543=CARTESIAN_POINT ( 'NONE',  ( -35.85663232820584057, 3.056483311920803025, 4.206888370749761741 ) ) ;
#6544=CARTESIAN_POINT ( 'NONE',  ( 15.61033468494287391, 5.277035221755904892, -1.205525476379225136 ) ) ;
#6545=DIRECTION ( 'NONE',  ( -1.000000000000000000, -0.000000000000000000, -0.000000000000000000 ) ) ;
#6546=CARTESIAN_POINT ( 'NONE',  ( 48.40000000000001990, 2.428612866367529932E-14, 0.000000000000000000 ) ) ;
#6550=ORIENTED_EDGE ( 'NONE', *, *, #25868, .T. ) ;
#6563=CIRCLE ( 'NONE', #13606, 1.000000000000000000 ) ;
#6566=ORIENTED_EDGE ( 'NONE', *, *, #9072, .F. ) ;
#6567=CARTESIAN_POINT ( 'NONE',  ( 51.70000000000001705, -3.826179070414207573, -1.000000000000000000 ) ) ;
#6569=DIRECTION ( 'NONE',  ( -0.9977167620779626711, 0.06753712067201277092, 8.270911865460929665E-18 ) ) ;
#6571=EDGE_LOOP ( 'NONE', ( #2028, #8639, #1491, #20747, #4328, #10607, #22377, #5105, #28423, #19541 ) ) ;
#6572=( BOUNDED_SURFACE ( )  B_SPLINE_SURFACE ( 3, 2, ( 
 ( #29607, #13144, #10923 ),
 ( #3027, #20304, #25012 ),
 ( #12671, #22352, #15833 ),
 ( #13282, #27401, #25341 ),
 ( #8095, #3340, #20615 ),
 ( #18078, #22971, #27722 ),
 ( #17604, #12819, #643 ),
 ( #17907, #17762, #8551 ),
 ( #29933, #5711, #15691 ),
 ( #27547, #15363, #19972 ),
 ( #10303, #27248, #5565 ),
 ( #12992, #3502, #1260 ),
 ( #1120, #10625, #30245 ),
 ( #6041, #18235, #27870 ),
 ( #15214, #24860, #22831 ),
 ( #22677, #6188, #974 ) ),
 .UNSPECIFIED., .F., .F., .F. ) 
 B_SPLINE_SURFACE_WITH_KNOTS ( ( 4, 2, 2, 2, 2, 2, 2, 4 ),
 ( 3, 3 ),
 ( 0.001780502285214199260, 0.002558945925323781977, 0.002753556835351177439, 0.002948167745378572902, 0.003337389565433364260, 0.003726611385488155619, 0.004115833205542946543, 0.004894276845652529261 ),
 ( 0.000000000000000000, 1.000000000000000000 ),
 .UNSPECIFIED. ) 
 GEOMETRIC_REPRESENTATION_ITEM ( )  RATIONAL_B_SPLINE_SURFACE ( (
 ( 1.000000000000000000, 0.9418517008537227175, 1.000000000000000000),
 ( 1.000000000000000000, 0.9417987965884856427, 1.000000000000000000),
 ( 1.000000000000000000, 0.9418198861734362604, 1.000000000000000000),
 ( 1.000000000000000000, 0.9434060303845490658, 1.000000000000000000),
 ( 1.000000000000000000, 0.9437939819948191200, 1.000000000000000000),
 ( 1.000000000000000000, 0.9445989566712758023, 1.000000000000000000),
 ( 1.000000000000000000, 0.9450169930049898692, 1.000000000000000000),
 ( 1.000000000000000000, 0.9461610507673464676, 1.000000000000000000),
 ( 1.000000000000000000, 0.9467217966427202702, 1.000000000000000000),
 ( 1.000000000000000000, 0.9467345476124352510, 1.000000000000000000),
 ( 1.000000000000000000, 0.9461964028052861631, 1.000000000000000000),
 ( 1.000000000000000000, 0.9446801822473912535, 1.000000000000000000),
 ( 1.000000000000000000, 0.9437582546536892325, 1.000000000000000000),
 ( 1.000000000000000000, 0.9418129560294941083, 1.000000000000000000),
 ( 1.000000000000000000, 0.9418016889778025869, 1.000000000000000000),
 ( 1.000000000000000000, 0.9418517008537231616, 1.000000000000000000) ) ) 
 REPRESENTATION_ITEM ( '' )  SURFACE ( )  );
#6573=CARTESIAN_POINT ( 'NONE',  ( 46.92075145057400931, -4.254543194710153742, -1.020305229671234937 ) ) ;
#6578=DIRECTION ( 'NONE',  ( 0.000000000000000000, -1.000000000000000000, 0.000000000000000000 ) ) ;
#6580=VECTOR ( 'NONE', #28443, 1000.000000000000000 ) ;
#6583=CARTESIAN_POINT ( 'NONE',  ( 57.04037853559506743, 0.7490840064628494499, -1.779165039991060571 ) ) ;
#6589=LINE ( 'NONE', #6902, #2653 ) ;
#6593=ORIENTED_EDGE ( 'NONE', *, *, #8216, .F. ) ;
#6599=FACE_OUTER_BOUND ( 'NONE', #21055, .T. ) ;
#6600=ORIENTED_EDGE ( 'NONE', *, *, #7794, .T. ) ;
#6605=CARTESIAN_POINT ( 'NONE',  ( 58.45000000000001705, -0.8000000000000000444, 2.421260002560649660 ) ) ;
#6606=DIRECTION ( 'NONE',  ( 2.459562394685744772E-16, -0.9510565162951523099, -0.3090169943749515591 ) ) ;
#6607=ORIENTED_EDGE ( 'NONE', *, *, #21461, .T. ) ;
#6608=CARTESIAN_POINT ( 'NONE',  ( -35.85663232820584057, 0.9159215771380343485, -4.311190327365813424 ) ) ;
#6610=AXIS2_PLACEMENT_3D ( 'NONE', #2534, #17105, #2678 ) ;
#6614=LINE ( 'NONE', #9308, #10951 ) ;
#6615=EDGE_CURVE ( 'NONE', #11900, #21791, #1008, .T. ) ;
#6616=EDGE_CURVE ( 'NONE', #13291, #25147, #26793, .T. ) ;
#6617=CARTESIAN_POINT ( 'NONE',  ( 57.05000000000001847, 0.8000000000000000444, 2.421260002560649660 ) ) ;
#6618=CARTESIAN_POINT ( 'NONE',  ( 50.49738912176885464, 0.9335627837658418970, -3.994936164801341061 ) ) ;
#6623=CARTESIAN_POINT ( 'NONE',  ( 46.90000000000001279, 1.734723475976807094E-15, 0.000000000000000000 ) ) ;
#6625=CARTESIAN_POINT ( 'NONE',  ( -36.56390771145571961, -0.2088129849843483599, 5.405094643512490471 ) ) ;
#6626=CARTESIAN_POINT ( 'NONE',  ( 48.40000000000002700, 0.6304760106459513791, -3.950000000000022826 ) ) ;
#6628=EDGE_CURVE ( 'NONE', #18794, #11503, #28829, .T. ) ;
#6630=DIRECTION ( 'NONE',  ( -2.459562394685737870E-16, 0.9510565162951500895, 0.3090169943749582204 ) ) ;
#6635=CYLINDRICAL_SURFACE ( 'NONE', #8801, 3.625000000000000444 ) ;
#6637=DIRECTION ( 'NONE',  ( 0.000000000000000000, 0.000000000000000000, -1.000000000000000000 ) ) ;
#6639=ORIENTED_EDGE ( 'NONE', *, *, #16474, .F. ) ;
#6646=DIRECTION ( 'NONE',  ( -1.000000000000000000, 0.000000000000000000, -0.000000000000000000 ) ) ;
#6648=EDGE_CURVE ( 'NONE', #12844, #29437, #15171, .T. ) ;
#6649=CARTESIAN_POINT ( 'NONE',  ( 57.00000000000001421, -0.7059996929583092218, 1.815412393553804460 ) ) ;
#6650=CARTESIAN_POINT ( 'NONE',  ( -36.56390771145525775, 3.345968172200181279, -4.250076229745598511 ) ) ;
#6655=CARTESIAN_POINT ( 'NONE',  ( 58.45000000000001705, 0.8156862745098041323, 2.468735688885368873 ) ) ;
#6657=DIRECTION ( 'NONE',  ( -0.000000000000000000, -0.000000000000000000, -1.000000000000000000 ) ) ;
#6658=CARTESIAN_POINT ( 'NONE',  ( 34.50000000000001421, 0.000000000000000000, 0.000000000000000000 ) ) ;
#6665=CARTESIAN_POINT ( 'NONE',  ( -36.30424252565904197, 4.911231426340481931, 1.712337380313478707 ) ) ;
#6666=CARTESIAN_POINT ( 'NONE',  ( 15.56401610563846027, -4.735424960531449123, 2.618558234550369956 ) ) ;
#6668=VERTEX_POINT ( 'NONE', #19848 ) ;
#6669=CARTESIAN_POINT ( 'NONE',  ( -36.48821680285229974, -5.256402525809805049, 1.287848407636970061 ) ) ;
#6673=VERTEX_POINT ( 'NONE', #25213 ) ;
#6679=ORIENTED_EDGE ( 'NONE', *, *, #26346, .F. ) ;
#6680=CIRCLE ( 'NONE', #24378, 0.04999999999999969746 ) ;
#6681=ORIENTED_EDGE ( 'NONE', *, *, #12126, .F. ) ;
#6684=EDGE_CURVE ( 'NONE', #25704, #2692, #20751, .T. ) ;
#6685=CARTESIAN_POINT ( 'NONE',  ( 58.45000000000001705, -0.7794871794871796045, 1.732743413496389939 ) ) ;
#6688=EDGE_CURVE ( 'NONE', #247, #23319, #20232, .T. ) ;
#6694=DIRECTION ( 'NONE',  ( 0.000000000000000000, 0.000000000000000000, -1.000000000000000000 ) ) ;
#6695=LINE ( 'NONE', #14289, #31170 ) ;
#6696=CARTESIAN_POINT ( 'NONE',  ( 56.95606009725792518, 0.7486802684473473635, 2.489875068279050918 ) ) ;
#6698=DIRECTION ( 'NONE',  ( 1.000000000000000000, -0.000000000000000000, -0.000000000000000000 ) ) ;
#6701=DIRECTION ( 'NONE',  ( 0.000000000000000000, 0.000000000000000000, -1.000000000000000000 ) ) ;
#6702=CARTESIAN_POINT ( 'NONE',  ( 48.43364830228694018, -1.250438735127598955, -3.874838289045730910 ) ) ;
#6704=ORIENTED_EDGE ( 'NONE', *, *, #7271, .F. ) ;
#6708=ADVANCED_FACE ( 'NONE', ( #27748 ), #18570, .T. ) ;
#6711=VERTEX_POINT ( 'NONE', #23315 ) ;
#6720=VERTEX_POINT ( 'NONE', #11259 ) ;
#6722=DIRECTION ( 'NONE',  ( -1.000000000000000000, 0.000000000000000000, 0.000000000000000000 ) ) ;
#6723=ADVANCED_FACE ( 'NONE', ( #24835 ), #10969, .T. ) ;
#6727=LINE ( 'NONE', #14167, #1771 ) ;
#6729=CARTESIAN_POINT ( 'NONE',  ( 56.95000000000001705, 0.6917305289283675052, 1.769637370168020141 ) ) ;
#6732=CARTESIAN_POINT ( 'NONE',  ( -36.21152527658241382, -2.821511581828405557, 4.377605326016305476 ) ) ;
#6734=DIRECTION ( 'NONE',  ( 0.000000000000000000, 0.000000000000000000, 1.000000000000000000 ) ) ;
#6737=VECTOR ( 'NONE', #9169, 1000.000000000000000 ) ;
#6738=VERTEX_POINT ( 'NONE', #30032 ) ;
#6748=EDGE_CURVE ( 'NONE', #30343, #3572, #9612, .T. ) ;
#6749=DIRECTION ( 'NONE',  ( 1.000000000000000000, 0.000000000000000000, 0.000000000000000000 ) ) ;
#6750=ORIENTED_EDGE ( 'NONE', *, *, #1110, .F. ) ;
#6755=PLANE ( 'NONE',  #25149 ) ;
#6756=EDGE_CURVE ( 'NONE', #22777, #7189, #15938, .T. ) ;
#6761=CARTESIAN_POINT ( 'NONE',  ( 56.99137905793185155, 0.7079296279778910517, -1.763407125847052725 ) ) ;
#6765=EDGE_CURVE ( 'NONE', #20590, #17963, #6563, .T. ) ;
#6766=CARTESIAN_POINT ( 'NONE',  ( -35.85663232820583346, -4.383220986679497777, 0.4611378927914391301 ) ) ;
#6770=ORIENTED_EDGE ( 'NONE', *, *, #21112, .F. ) ;
#6773=CARTESIAN_POINT ( 'NONE',  ( -36.89250464418362441, -0.3169205264059772320, 5.400007398663888125 ) ) ;
#6774=DIRECTION ( 'NONE',  ( 0.000000000000000000, 0.3589743589743593088, -0.9333474217026304087 ) ) ;
#6775=EDGE_LOOP ( 'NONE', ( #28527, #19278, #13329, #25635 ) ) ;
#6780=DIRECTION ( 'NONE',  ( 0.000000000000000000, 0.9663289263986323263, -0.2573099415204678220 ) ) ;
#6784=ORIENTED_EDGE ( 'NONE', *, *, #304, .T. ) ;
#6785=B_SPLINE_CURVE_WITH_KNOTS ( 'NONE', 3,
 ( #24559, #26645, #3186, #12827, #4949, #14605, #2581, #10160, #15067, #651, #7946, #24270, #17611, #9853, #27256, #19525 ),
 .UNSPECIFIED., .F., .F.,
 ( 4, 2, 2, 2, 2, 2, 2, 4 ),
 ( 1.734723475976806902E-18, 0.0004351083927046452463, 0.0008702167854092887579, 0.001740433570818576648, 0.002175541963523220865, 0.002610650356227864864, 0.003045758748932509297, 0.003480867141637153730 ),
 .UNSPECIFIED. ) ;
#6786=LINE ( 'NONE', #30699, #30542 ) ;
#6788=CARTESIAN_POINT ( 'NONE',  ( 51.90000000000001279, 1.734723475976807094E-15, 0.000000000000000000 ) ) ;
#6794=CARTESIAN_POINT ( 'NONE',  ( 15.03925126672133139, -4.683225679163337318, -2.703237727951242508 ) ) ;
#6800=CARTESIAN_POINT ( 'NONE',  ( 57.00529107662529782, -0.7231510886217332734, 1.801575813826951533 ) ) ;
#6801=CARTESIAN_POINT ( 'NONE',  ( -36.92443669619591873, 3.305069970238394994, -4.282766538619357632 ) ) ;
#6805=DIRECTION ( 'NONE',  ( 0.000000000000000000, -0.000000000000000000, 1.000000000000000000 ) ) ;
#6806=DIRECTION ( 'NONE',  ( 0.000000000000000000, 0.000000000000000000, 1.000000000000000000 ) ) ;
#6810=LINE ( 'NONE', #2064, #28669 ) ;
#6815=CARTESIAN_POINT ( 'NONE',  ( 15.86395258069112835, -2.563573972737278606, -4.761506352252398599 ) ) ;
#6816=CARTESIAN_POINT ( 'NONE',  ( -36.63359589171323449, 5.330414537250494966, 0.9106291984479393253 ) ) ;
#6817=CARTESIAN_POINT ( 'NONE',  ( 15.48686146417454523, -4.911231426340524564, 1.712337380313389001 ) ) ;
#6821=ORIENTED_EDGE ( 'NONE', *, *, #13887, .T. ) ;
#6822=CARTESIAN_POINT ( 'NONE',  ( -36.22818246778668083, -4.895960019030552779, 2.323379425334354043 ) ) ;
#6823=DIRECTION ( 'NONE',  ( -2.459562394685738363E-16, 0.9510565162951500895, 0.3090169943749582759 ) ) ;
#6836=ORIENTED_EDGE ( 'NONE', *, *, #1905, .T. ) ;
#6841=CARTESIAN_POINT ( 'NONE',  ( 56.95000000000001705, -0.7137254901960785602, 2.500119182087999548 ) ) ;
#6847=DIRECTION ( 'NONE',  ( 0.000000000000000000, 1.000000000000000000, -8.673617379884030739E-15 ) ) ;
#6849=CARTESIAN_POINT ( 'NONE',  ( 47.07338444802540778, -4.179189466084497262, 0.9999999999999988898 ) ) ;
#6852=CARTESIAN_POINT ( 'NONE',  ( 15.81621483022862407, 5.330414537250522500, -0.9106291984478636081 ) ) ;
#6854=DIRECTION ( 'NONE',  ( 0.000000000000000000, 0.000000000000000000, 1.000000000000000000 ) ) ;
#6863=ADVANCED_FACE ( 'NONE', ( #110 ), #5889, .T. ) ;
#6868=ORIENTED_EDGE ( 'NONE', *, *, #4153, .T. ) ;
#6869=ORIENTED_EDGE ( 'NONE', *, *, #26722, .T. ) ;
#6878=LINE ( 'NONE', #11786, #24290 ) ;
#6881=ORIENTED_EDGE ( 'NONE', *, *, #24152, .F. ) ;
#6884=DIRECTION ( 'NONE',  ( 1.000000000000000000, 0.000000000000000000, 0.000000000000000000 ) ) ;
#6887=CARTESIAN_POINT ( 'NONE',  ( 56.96003682719288008, -0.7597908294545935304, -2.486534234876009553 ) ) ;
#6888=ORIENTED_EDGE ( 'NONE', *, *, #22226, .T. ) ;
#6896=PLANE ( 'NONE',  #10856 ) ;
#6897=EDGE_CURVE ( 'NONE', #25072, #6720, #26538, .T. ) ;
#6902=CARTESIAN_POINT ( 'NONE',  ( 58.50000000000001421, -0.8156862745098042433, -2.468735688885369317 ) ) ;
#6909=DIRECTION ( 'NONE',  ( -1.000000000000000000, -0.000000000000000000, -0.000000000000000000 ) ) ;
#6910=ORIENTED_EDGE ( 'NONE', *, *, #23146, .F. ) ;
#6911=ADVANCED_FACE ( 'NONE', ( #26072 ), #4381, .F. ) ;
#6916=CARTESIAN_POINT ( 'NONE',  ( -35.85663232820581925, 3.779372838781723587, 3.883777296072584484 ) ) ;
#6920=VERTEX_POINT ( 'NONE', #29520 ) ;
#6922=ORIENTED_EDGE ( 'NONE', *, *, #21431, .F. ) ;
#6923=CARTESIAN_POINT ( 'NONE',  ( 50.42159256128543632, 1.310166284604407760, 3.885185101012171849 ) ) ;
#6931=AXIS2_PLACEMENT_3D ( 'NONE', #25492, #27555, #20459 ) ;
#6932=CARTESIAN_POINT ( 'NONE',  ( 57.05000000000001137, 0.7500000000000001110, -1.778341924377885963 ) ) ;
#6943=EDGE_CURVE ( 'NONE', #26007, #10689, #27163, .T. ) ;
#6945=CIRCLE ( 'NONE', #30187, 3.200000000000000178 ) ;
#6946=CARTESIAN_POINT ( 'NONE',  ( -35.85663232820584057, 1.123735532908267665, -5.289358697221546279 ) ) ;
#6949=CARTESIAN_POINT ( 'NONE',  ( 48.38568300895507690, 1.130504494894958745, -3.941663789486467895 ) ) ;
#6951=CARTESIAN_POINT ( 'NONE',  ( -35.85663232820583346, -4.683225679163361299, 2.703237727951226077 ) ) ;
#6955=DIRECTION ( 'NONE',  ( 1.000000000000000000, 0.000000000000000000, 0.000000000000000000 ) ) ;
#6957=ORIENTED_EDGE ( 'NONE', *, *, #7264, .F. ) ;
#6962=AXIS2_PLACEMENT_3D ( 'NONE', #903, #26440, #2381 ) ;
#6966=ORIENTED_EDGE ( 'NONE', *, *, #31098, .F. ) ;
#6968=CARTESIAN_POINT ( 'NONE',  ( 15.03925126672132961, 4.018128179617565188, -3.618665901676623164 ) ) ;
#6974=AXIS2_PLACEMENT_3D ( 'NONE', #27831, #6140, #5994 ) ;
#6978=AXIS2_PLACEMENT_3D ( 'NONE', #11281, #8908, #18905 ) ;
#6979=CARTESIAN_POINT ( 'NONE',  ( -36.48174642953001978, 2.847679722116494005, -4.601476325142689561 ) ) ;
#6980=CARTESIAN_POINT ( 'NONE',  ( 48.40000000000001279, 0.7619326981554777056, 3.939508824314740032 ) ) ;
#6997=CARTESIAN_POINT ( 'NONE',  ( -36.56242893520595061, 5.206628483174555733, 1.466363261642575466 ) ) ;
#6998=CARTESIAN_POINT ( 'NONE',  ( 15.68751737981894578, -5.244794032782597704, 1.329291831544269664 ) ) ;
#7001=DIRECTION ( 'NONE',  ( 1.000000000000000000, 0.000000000000000000, 0.000000000000000000 ) ) ;
#7005=CARTESIAN_POINT ( 'NONE',  ( 56.99229849798533820, -0.7794861535680733811, -1.732743875013533108 ) ) ;
#7007=ORIENTED_EDGE ( 'NONE', *, *, #4821, .F. ) ;
#7013=ORIENTED_EDGE ( 'NONE', *, *, #8735, .T. ) ;
#7016=FACE_OUTER_BOUND ( 'NONE', #29348, .T. ) ;
#7020=AXIS2_PLACEMENT_3D ( 'NONE', #13815, #17175, #29481 ) ;
#7026=DIRECTION ( 'NONE',  ( -1.000000000000000000, 0.000000000000000000, 0.000000000000000000 ) ) ;
#7033=CARTESIAN_POINT ( 'NONE',  ( 50.33290990662630549, -1.365599538210731767, 3.854893000251053081 ) ) ;
#7036=EDGE_CURVE ( 'NONE', #14986, #1995, #29341, .T. ) ;
#7042=ORIENTED_EDGE ( 'NONE', *, *, #15952, .F. ) ;
#7043=FACE_OUTER_BOUND ( 'NONE', #27892, .T. ) ;
#7045=CARTESIAN_POINT ( 'NONE',  ( 48.43966969621122587, -1.282137971188096914, 3.869545987293864453 ) ) ;
#7049=ORIENTED_EDGE ( 'NONE', *, *, #18215, .F. ) ;
#7052=DIRECTION ( 'NONE',  ( 0.000000000000000000, 0.000000000000000000, -1.000000000000000000 ) ) ;
#7060=DIRECTION ( 'NONE',  ( -1.000000000000000000, -0.000000000000000000, -0.000000000000000000 ) ) ;
#7064=DIRECTION ( 'NONE',  ( 1.000000000000000000, 0.000000000000000000, -0.000000000000000000 ) ) ;
#7067=AXIS2_PLACEMENT_3D ( 'NONE', #12800, #16959, #14577 ) ;
#7068=DIRECTION ( 'NONE',  ( 0.000000000000000000, 0.000000000000000000, 1.000000000000000000 ) ) ;
#7075=CARTESIAN_POINT ( 'NONE',  ( -36.11122220296839203, 3.378548217643384977, 3.972894518062678237 ) ) ;
#7081=VERTEX_POINT ( 'NONE', #15283 ) ;
#7082=CARTESIAN_POINT ( 'NONE',  ( -36.52757395963740095, 5.349060760730894870, 0.7993770229879135769 ) ) ;
#7083=ORIENTED_EDGE ( 'NONE', *, *, #14371, .T. ) ;
#7095=CARTESIAN_POINT ( 'NONE',  ( 17.21035195517769267, -24.59258869922087243, -3.011723503324820852E-15 ) ) ;
#7100=CARTESIAN_POINT ( 'NONE',  ( -36.52679053911622020, -0.8934212604923426060, 5.334164326942878454 ) ) ;
#7102=CARTESIAN_POINT ( 'NONE',  ( 57.03821272586434787, -0.7500000328843418052, -2.490438846756156899 ) ) ;
#7103=CARTESIAN_POINT ( 'NONE',  ( -54.45495050826418293, 1.499999999999999112, 3.300094695611021756 ) ) ;
#7105=ORIENTED_EDGE ( 'NONE', *, *, #28039, .F. ) ;
#7106=ADVANCED_FACE ( 'NONE', ( #1182 ), #3558, .F. ) ;
#7107=CARTESIAN_POINT ( 'NONE',  ( -54.46895629856896903, 1.503487923075246480, 4.032311158269683560 ) ) ;
#7109=CARTESIAN_POINT ( 'NONE',  ( 15.29954477411491354, 1.123735554575626461, -5.289358692618272073 ) ) ;
#7111=FACE_OUTER_BOUND ( 'NONE', #10832, .T. ) ;
#7116=DIRECTION ( 'NONE',  ( 0.000000000000000000, 0.000000000000000000, -1.000000000000000000 ) ) ;
#7121=DIRECTION ( 'NONE',  ( 1.000000000000000000, -0.000000000000000000, -0.000000000000000000 ) ) ;
#7122=CARTESIAN_POINT ( 'NONE',  ( 46.90000000000001990, -4.241638912518125082, -1.073342218585543684 ) ) ;
#7124=FACE_OUTER_BOUND ( 'NONE', #7188, .T. ) ;
#7127=EDGE_CURVE ( 'NONE', #30388, #25072, #17218, .T. ) ;
#7128=CARTESIAN_POINT ( 'NONE',  ( -54.49853245345825314, 1.536420219664552667, -4.055116445457033869 ) ) ;
#7131=FACE_OUTER_BOUND ( 'NONE', #14913, .T. ) ;
#7146=CARTESIAN_POINT ( 'NONE',  ( -35.85663232820583346, -4.817150320980530864, 2.203324261490539282 ) ) ;
#7147=CARTESIAN_POINT ( 'NONE',  ( -36.38139716712352367, 4.735424960531724459, 2.618558234549792196 ) ) ;
#7148=CARTESIAN_POINT ( 'NONE',  ( 15.48609859788817822, -4.980680447166701441, 1.498595263773770281 ) ) ;
#7154=CARTESIAN_POINT ( 'NONE',  ( 57.00791613703923844, 0.8068646677135199452, -2.471635681327667644 ) ) ;
#7157=ADVANCED_FACE ( 'NONE', ( #17978 ), #10692, .T. ) ;
#7159=ORIENTED_EDGE ( 'NONE', *, *, #19405, .T. ) ;
#7167=ORIENTED_EDGE ( 'NONE', *, *, #10819, .F. ) ;
#7170=DIRECTION ( 'NONE',  ( 0.000000000000000000, 0.000000000000000000, -1.000000000000000000 ) ) ;
#7173=VECTOR ( 'NONE', #113, 1000.000000000000000 ) ;
#7176=CARTESIAN_POINT ( 'NONE',  ( 47.04702152735704601, -4.174452932061539556, 1.011256013762273698 ) ) ;
#7177=CARTESIAN_POINT ( 'NONE',  ( 57.00000000000001421, 0.000000000000000000, 0.000000000000000000 ) ) ;
#7178=DIRECTION ( 'NONE',  ( 0.000000000000000000, 0.000000000000000000, -1.000000000000000000 ) ) ;
#7181=DIRECTION ( 'NONE',  ( 0.000000000000000000, 0.000000000000000000, -1.000000000000000000 ) ) ;
#7182=CARTESIAN_POINT ( 'NONE',  ( 50.32622512580982033, 1.373801017329653762, -3.853344662332955473 ) ) ;
#7183=DIRECTION ( 'NONE',  ( 1.000000000000000000, -0.000000000000000000, -0.000000000000000000 ) ) ;
#7188=EDGE_LOOP ( 'NONE', ( #12875, #7583, #4218, #14700 ) ) ;
#7189=VERTEX_POINT ( 'NONE', #11297 ) ;
#7192=ORIENTED_EDGE ( 'NONE', *, *, #20116, .F. ) ;
#7195=CARTESIAN_POINT ( 'NONE',  ( 48.40000000000001990, -4.899999999999999467, -3.850000000000022737 ) ) ;
#7196=AXIS2_PLACEMENT_3D ( 'NONE', #11642, #6884, #14314 ) ;
#7208=CARTESIAN_POINT ( 'NONE',  ( 57.05000000000001847, 0.7794871794871796045, 1.732743413496389939 ) ) ;
#7210=FACE_OUTER_BOUND ( 'NONE', #22263, .T. ) ;
#7211=CARTESIAN_POINT ( 'NONE',  ( 51.70000000000001705, -4.276948333784443612, 0.9210526315789470120 ) ) ;
#7216=ORIENTED_EDGE ( 'NONE', *, *, #16363, .T. ) ;
#7219=ORIENTED_EDGE ( 'NONE', *, *, #20376, .T. ) ;
#7223=DIRECTION ( 'NONE',  ( 0.000000000000000000, 0.000000000000000000, -1.000000000000000000 ) ) ;
#7224=ORIENTED_EDGE ( 'NONE', *, *, #6684, .F. ) ;
#7231=CARTESIAN_POINT ( 'NONE',  ( -35.85663232820584767, 4.683225679163309785, 2.703237727951257607 ) ) ;
#7234=DIRECTION ( 'NONE',  ( 1.000000000000000000, -0.000000000000000000, -0.000000000000000000 ) ) ;
#7236=CARTESIAN_POINT ( 'NONE',  ( 57.00000000000001421, 0.6999999999999996225, -1.820027472320129736 ) ) ;
#7239=DIRECTION ( 'NONE',  ( 0.000000000000000000, 0.000000000000000000, 1.000000000000000000 ) ) ;
#7240=AXIS2_PLACEMENT_3D ( 'NONE', #27492, #5812, #2972 ) ;
#7250=CARTESIAN_POINT ( 'NONE',  ( 15.74504787372188730, 0.2143423494564743459, -5.404929114625646847 ) ) ;
#7254=CARTESIAN_POINT ( 'NONE',  ( 50.50000000000002132, 2.428612866367529932E-14, 0.000000000000000000 ) ) ;
#7261=VECTOR ( 'NONE', #7286, 1000.000000000000000 ) ;
#7263=FACE_OUTER_BOUND ( 'NONE', #3363, .T. ) ;
#7264=EDGE_CURVE ( 'NONE', #17419, #7270, #30860, .T. ) ;
#7266=CARTESIAN_POINT ( 'NONE',  ( 16.00221665700883733, -3.629052419422202913, -4.014440194077229407 ) ) ;
#7270=VERTEX_POINT ( 'NONE', #18615 ) ;
#7271=EDGE_CURVE ( 'NONE', #10898, #13515, #6878, .T. ) ;
#7273=CARTESIAN_POINT ( 'NONE',  ( 15.49702763512084580, -3.012234853004051693, 4.239036759381619390 ) ) ;
#7275=DIRECTION ( 'NONE',  ( 0.000000000000000000, 0.000000000000000000, 1.000000000000000000 ) ) ;
#7278=LINE ( 'NONE', #24066, #18579 ) ;
#7286=DIRECTION ( 'NONE',  ( 1.000000000000000000, -0.000000000000000000, -0.000000000000000000 ) ) ;
#7289=CARTESIAN_POINT ( 'NONE',  ( -44.49999999999999289, -6.938893903907228378E-14, 0.000000000000000000 ) ) ;
#7291=CARTESIAN_POINT ( 'NONE',  ( 15.03925126672132961, -1.123735532908297863, -5.289358697221544503 ) ) ;
#7297=ORIENTED_EDGE ( 'NONE', *, *, #5716, .T. ) ;
#7298=DIRECTION ( 'NONE',  ( 0.000000000000000000, 0.000000000000000000, -1.000000000000000000 ) ) ;
#7301=ORIENTED_EDGE ( 'NONE', *, *, #3707, .T. ) ;
#7302=ADVANCED_FACE ( 'NONE', ( #14159 ), #30946, .T. ) ;
#7305=( NAMED_UNIT ( * ) SI_UNIT ( $, .STERADIAN. ) SOLID_ANGLE_UNIT ( ) );
#7307=EDGE_LOOP ( 'NONE', ( #14058, #17165, #8718, #20081, #907, #2778, #29188, #21372, #16617, #26481, #6149, #26206, #1408, #24960, #3268, #15644, #13782 ) ) ;
#7311=ORIENTED_EDGE ( 'NONE', *, *, #19157, .F. ) ;
#7315=DIRECTION ( 'NONE',  ( 0.000000000000000000, 0.000000000000000000, -1.000000000000000000 ) ) ;
#7318=CARTESIAN_POINT ( 'NONE',  ( -36.26369610968609436, 0.2166734227622153230, -5.199999998324989825 ) ) ;
#7322=CARTESIAN_POINT ( 'NONE',  ( 48.45862863613067617, 1.344608935533184946, -3.858631320448700386 ) ) ;
#7329=CARTESIAN_POINT ( 'NONE',  ( -36.52757395963739384, -5.349060760730933062, -0.7993770229878666145 ) ) ;
#7330=CARTESIAN_POINT ( 'NONE',  ( 48.41280093284956365, -1.295960864328790541, 3.889961360030774973 ) ) ;
#7331=CARTESIAN_POINT ( 'NONE',  ( 50.30000000000001847, -1.426739617975179675, 3.843750000000022649 ) ) ;
#7341=CARTESIAN_POINT ( 'NONE',  ( 15.45522337368514343, 4.885888067249533506, 1.790336215468755654 ) ) ;
#7346=FACE_OUTER_BOUND ( 'NONE', #14535, .T. ) ;
#7357=DIRECTION ( 'NONE',  ( 1.000000000000000000, -0.000000000000000000, -0.000000000000000000 ) ) ;
#7368=CARTESIAN_POINT ( 'NONE',  ( 51.87895135909221267, 0.03408243259258914720, -4.372659797885439126 ) ) ;
#7373=CARTESIAN_POINT ( 'NONE',  ( 51.80000000000001847, -3.726179070414207928, -1.100000000000000089 ) ) ;
#7376=ORIENTED_EDGE ( 'NONE', *, *, #21836, .F. ) ;
#7377=CYLINDRICAL_SURFACE ( 'NONE', #1748, 0.05000000000000143219 ) ;
#7381=CARTESIAN_POINT ( 'NONE',  ( 47.10000000000002274, -4.179189514726506793, -1.000000000000000000 ) ) ;
#7388=DIRECTION ( 'NONE',  ( -8.673617379883787770E-15, 0.000000000000000000, -1.000000000000000000 ) ) ;
#7406=LINE ( 'NONE', #7706, #13038 ) ;
#7407=CARTESIAN_POINT ( 'NONE',  ( -54.48167032960165557, 1.510995100284905579, 3.307167554963766243 ) ) ;
#7410=CARTESIAN_POINT ( 'NONE',  ( -36.92405921417686443, -5.098435263432280706, 1.807398698456160302 ) ) ;
#7411=ORIENTED_EDGE ( 'NONE', *, *, #10551, .T. ) ;
#7413=CARTESIAN_POINT ( 'NONE',  ( 15.03925126672127810, 0.4576450603547064233, -5.200000000000000178 ) ) ;
#7414=CARTESIAN_POINT ( 'NONE',  ( -36.92362342067168868, -5.092377074781566648, 1.825725187625063972 ) ) ;
#7416=DIRECTION ( 'NONE',  ( 0.000000000000000000, 0.000000000000000000, -1.000000000000000000 ) ) ;
#7422=CARTESIAN_POINT ( 'NONE',  ( 50.30000000000001847, -1.409787217987148233, -3.850000000000022737 ) ) ;
#7424=CARTESIAN_POINT ( 'NONE',  ( -54.49131719536980967, -1.521332553059528081, -4.044684194243342468 ) ) ;
#7430=CARTESIAN_POINT ( 'NONE',  ( 15.97944027357902463, -2.710596767400041518, -4.680923748383032823 ) ) ;
#7436=CARTESIAN_POINT ( 'NONE',  ( -54.49999999999997868, 4.900000000000003020, 0.000000000000000000 ) ) ;
#7439=AXIS2_PLACEMENT_3D ( 'NONE', #13270, #18064, #25633 ) ;
#7443=ADVANCED_FACE ( 'NONE', ( #7512 ), #7656, .T. ) ;
#7444=AXIS2_PLACEMENT_3D ( 'NONE', #21979, #2658, #9488 ) ;
#7447=CARTESIAN_POINT ( 'NONE',  ( 56.95000000000001705, 0.7137254901960785602, -2.500119182087999548 ) ) ;
#7449=EDGE_LOOP ( 'NONE', ( #4839, #25390, #9499, #27267 ) ) ;
#7450=CIRCLE ( 'NONE', #29195, 0.05000000000000143219 ) ;
#7452=AXIS2_PLACEMENT_3D ( 'NONE', #24503, #25137, #2814 ) ;
#7455=CARTESIAN_POINT ( 'NONE',  ( 15.94709373951305764, -2.670851142931433664, -4.702170608191262424 ) ) ;
#7457=DIRECTION ( 'NONE',  ( 0.000000000000000000, 0.000000000000000000, -1.000000000000000000 ) ) ;
#7462=CARTESIAN_POINT ( 'NONE',  ( 51.76980060221182356, -4.166995010554928491, 1.027517533905028868 ) ) ;
#7466=CARTESIAN_POINT ( 'NONE',  ( -36.50489844130356687, -5.244794032782665205, -1.329291831544206381 ) ) ;
#7467=ORIENTED_EDGE ( 'NONE', *, *, #18154, .F. ) ;
#7468=( LENGTH_UNIT ( ) NAMED_UNIT ( * ) SI_UNIT ( .MILLI., .METRE. ) );
#7471=TOROIDAL_SURFACE ( 'NONE', #2428, 2.549999999999999822, 0.05000000000000000278 ) ;
#7472=ORIENTED_EDGE ( 'NONE', *, *, #8113, .F. ) ;
#7475=AXIS2_PLACEMENT_3D ( 'NONE', #14024, #23714, #1674 ) ;
#7480=CARTESIAN_POINT ( 'NONE',  ( 51.76237124553680502, -4.256129153948959853, -1.015733033895005688 ) ) ;
#7490=CARTESIAN_POINT ( 'NONE',  ( 54.43308742068420969, -0.0001827659102894963578, -4.369367483123359541 ) ) ;
#7496=CARTESIAN_POINT ( 'NONE',  ( 48.38568300895507690, -1.130504494894903456, 3.941663789486468339 ) ) ;
#7498=CARTESIAN_POINT ( 'NONE',  ( 57.00000000000000711, 0.7137254901960808917, 2.500119182088006209 ) ) ;
#7512=FACE_OUTER_BOUND ( 'NONE', #12613, .T. ) ;
#7514=AXIS2_PLACEMENT_3D ( 'NONE', #23925, #11406, #3972 ) ;
#7522=DIRECTION ( 'NONE',  ( 0.000000000000000000, -1.000000000000000000, 0.000000000000000000 ) ) ;
#7525=CARTESIAN_POINT ( 'NONE',  ( -36.04581030752770943, -3.779372845003824644, 3.883777290285136186 ) ) ;
#7526=DIRECTION ( 'NONE',  ( -0.000000000000000000, -2.168404344971007882E-16, -1.000000000000000000 ) ) ;
#7527=EDGE_CURVE ( 'NONE', #29305, #7081, #20791, .T. ) ;
#7537=CARTESIAN_POINT ( 'NONE',  ( 47.00000000000002132, 1.391941090707534023, -3.750000000000022649 ) ) ;
#7548=VERTEX_POINT ( 'NONE', #21935 ) ;
#7552=EDGE_CURVE ( 'NONE', #17419, #25469, #15249, .T. ) ;
#7553=CARTESIAN_POINT ( 'NONE',  ( 15.49676243306307732, -4.927920137446233362, -1.660974799722084061 ) ) ;
#7562=DIRECTION ( 'NONE',  ( 0.000000000000000000, -0.1576190026614809614, 0.9875000000000001554 ) ) ;
#7568=DIRECTION ( 'NONE',  ( 0.000000000000000000, -0.4102564102564100201, 0.9119702176296790030 ) ) ;
#7569=AXIS2_PLACEMENT_3D ( 'NONE', #16700, #23969, #17587 ) ;
#7579=DIRECTION ( 'NONE',  ( 0.000000000000000000, 0.000000000000000000, -1.000000000000000000 ) ) ;
#7580=AXIS2_PLACEMENT_3D ( 'NONE', #11905, #16507, #7170 ) ;
#7582=DIRECTION ( 'NONE',  ( 0.000000000000000000, -1.000000000000000000, 0.000000000000000000 ) ) ;
#7583=ORIENTED_EDGE ( 'NONE', *, *, #23686, .T. ) ;
#7590=CARTESIAN_POINT ( 'NONE',  ( 58.50000000000001421, 0.000000000000000000, 0.000000000000000000 ) ) ;
#7593=CARTESIAN_POINT ( 'NONE',  ( 15.41080140630215922, -3.722599991951294207, 3.938370952810156478 ) ) ;
#7594=B_SPLINE_CURVE_WITH_KNOTS ( 'NONE', 3,
 ( #21550, #15138, #19330, #14085, #30875, #28966, #4589, #11569, #9344, #19899, #4, #12600 ),
 .UNSPECIFIED., .F., .F.,
 ( 4, 2, 2, 2, 2, 4 ),
 ( 0.000000000000000000, 5.522938194211708289E-05, 0.0001104587638842341658, 0.0002209175277684793091, 0.0004418350555369705986, 0.0008836701110739516056 ),
 .UNSPECIFIED. ) ;
#7603=ORIENTED_EDGE ( 'NONE', *, *, #4082, .F. ) ;
#7607=FACE_OUTER_BOUND ( 'NONE', #23453, .T. ) ;
#7608=CARTESIAN_POINT ( 'NONE',  ( 57.01173390802158991, 0.7326096616897963543, -2.432492958759772783 ) ) ;
#7609=DIRECTION ( 'NONE',  ( 0.000000000000000000, -2.168404344971008868E-16, -1.000000000000000000 ) ) ;
#7614=DIRECTION ( 'NONE',  ( 0.000000000000000000, 0.000000000000000000, -1.000000000000000000 ) ) ;
#7615=VERTEX_POINT ( 'NONE', #3953 ) ;
#7617=CARTESIAN_POINT ( 'NONE',  ( 50.40000000000003411, 0.7618928438397208902, 3.939512004971702730 ) ) ;
#7620=EDGE_CURVE ( 'NONE', #23640, #28800, #20181, .T. ) ;
#7626=CARTESIAN_POINT ( 'NONE',  ( 48.37884656342667711, -0.9200365198983474491, -3.998286360709680576 ) ) ;
#7627=CARTESIAN_POINT ( 'NONE',  ( -54.44999999999997442, -1.500000000000000000, 3.300094695611020867 ) ) ;
#7628=CARTESIAN_POINT ( 'NONE',  ( 54.40000000000001990, -1.084202172485504434E-16, 4.374999999999999112 ) ) ;
#7634=CARTESIAN_POINT ( 'NONE',  ( 48.43359507746255588, 1.250162886418204389, -3.874884102585954171 ) ) ;
#7639=CARTESIAN_POINT ( 'NONE',  ( -36.79682133506354091, -5.289443499204832477, -1.131445731060801707 ) ) ;
#7645=VERTEX_POINT ( 'NONE', #6491 ) ;
#7646=CARTESIAN_POINT ( 'NONE',  ( -37.18272003341174070, -1.653865106024005477E-14, 0.000000000000000000 ) ) ;
#7650=ORIENTED_EDGE ( 'NONE', *, *, #11832, .T. ) ;
#7651=CARTESIAN_POINT ( 'NONE',  ( 48.43359507746254877, -1.250162886418155761, 3.874884102585953727 ) ) ;
#7652=ADVANCED_FACE ( 'NONE', ( #26114 ), #10659, .F. ) ;
#7656=CYLINDRICAL_SURFACE ( 'NONE', #25313, 1.000000000000000000 ) ;
#7660=VECTOR ( 'NONE', #17371, 1000.000000000000000 ) ;
#7665=CARTESIAN_POINT ( 'NONE',  ( 57.00875904852982501, -0.7282698412063691729, 2.435189460583063514 ) ) ;
#7667=CARTESIAN_POINT ( 'NONE',  ( -36.92362342067078629, -3.046685255238732459, 4.470266847515959263 ) ) ;
#7675=EDGE_LOOP ( 'NONE', ( #13633, #2807, #15571, #31226 ) ) ;
#7676=CIRCLE ( 'NONE', #18312, 0.05000000000000017625 ) ;
#7690=EDGE_CURVE ( 'NONE', #7270, #8110, #39, .T. ) ;
#7692=DIRECTION ( 'NONE',  ( 1.000000000000000000, -0.000000000000000000, -0.000000000000000000 ) ) ;
#7693=EDGE_CURVE ( 'NONE', #23272, #25117, #30879, .T. ) ;
#7694=CARTESIAN_POINT ( 'NONE',  ( 57.02474788916244108, 0.7434350531339385393, 1.784201504348416067 ) ) ;
#7695=CARTESIAN_POINT ( 'NONE',  ( 15.30042582489636160, -5.377732434016963659, -0.5657657146875257892 ) ) ;
#7698=DIRECTION ( 'NONE',  ( -0.000000000000000000, 0.9875000000000001554, 0.1576190026614806561 ) ) ;
#7699=CARTESIAN_POINT ( 'NONE',  ( 50.46953806735880477, 1.143620537822834349, -3.937943076466140724 ) ) ;
#7702=CIRCLE ( 'NONE', #16310, 0.05000000000000012768 ) ;
#7706=CARTESIAN_POINT ( 'NONE',  ( 57.05000000000001847, 0.7500000000000000000, 1.745709025009609228 ) ) ;
#7709=CARTESIAN_POINT ( 'NONE',  ( 50.36673905152862574, 1.398826622412688403, -3.854114288381606190 ) ) ;
#7712=CARTESIAN_POINT ( 'NONE',  ( -35.98994760229852830, -5.086913989684993531, 1.171642050077752462 ) ) ;
#7718=FACE_OUTER_BOUND ( 'NONE', #31084, .T. ) ;
#7721=DIRECTION ( 'NONE',  ( 0.000000000000000000, 1.532429380227445212E-15, -1.000000000000000000 ) ) ;
#7725=DIRECTION ( 'NONE',  ( 0.000000000000000000, -1.000000000000000000, 0.000000000000000000 ) ) ;
#7729=DIRECTION ( 'NONE',  ( -1.000000000000000000, -2.586136946169074517E-16, 0.000000000000000000 ) ) ;
#7731=VERTEX_POINT ( 'NONE', #17797 ) ;
#7732=CARTESIAN_POINT ( 'NONE',  ( 15.03925126672127810, -3.426725943139564912, 3.937891353488730317 ) ) ;
#7738=CARTESIAN_POINT ( 'NONE',  ( 50.40000000000001990, -0.7618928438396727065, -3.939512004971702730 ) ) ;
#7740=ORIENTED_EDGE ( 'NONE', *, *, #7850, .T. ) ;
#7741=ORIENTED_EDGE ( 'NONE', *, *, #28819, .T. ) ;
#7745=CARTESIAN_POINT ( 'NONE',  ( 15.56401610563845672, -3.953723660658770900, -3.694477770903854541 ) ) ;
#7747=LINE ( 'NONE', #14868, #29719 ) ;
#7749=EDGE_LOOP ( 'NONE', ( #22078, #7192, #3484, #18607, #31156 ) ) ;
#7750=ORIENTED_EDGE ( 'NONE', *, *, #24316, .T. ) ;
#7751=DIRECTION ( 'NONE',  ( 0.000000000000000000, 0.000000000000000000, 1.000000000000000000 ) ) ;
#7753=ORIENTED_EDGE ( 'NONE', *, *, #29471, .T. ) ;
#7755=LINE ( 'NONE', #17421, #1239 ) ;
#7757=ORIENTED_EDGE ( 'NONE', *, *, #30680, .F. ) ;
#7759=ADVANCED_FACE ( 'NONE', ( #6 ), #17237, .T. ) ;
#7760=CARTESIAN_POINT ( 'NONE',  ( 50.30000000000001847, -4.899999999999999467, -3.950000000000022826 ) ) ;
#7768=FACE_OUTER_BOUND ( 'NONE', #26461, .T. ) ;
#7769=CARTESIAN_POINT ( 'NONE',  ( 51.70000000000001705, -4.259946800035232073, -1.000000000000000222 ) ) ;
#7770=DIRECTION ( 'NONE',  ( 0.000000000000000000, 0.000000000000000000, -1.000000000000000000 ) ) ;
#7772=CARTESIAN_POINT ( 'NONE',  ( -36.76447480099743359, -0.6031025731806715084, -5.374022845360705958 ) ) ;
#7776=CARTESIAN_POINT ( 'NONE',  ( 16.10624235918716352, 5.192953935288670664, -1.516181439821520538 ) ) ;
#7780=CARTESIAN_POINT ( 'NONE',  ( 50.41431699104521158, -1.130504494894903900, -3.941663789486498093 ) ) ;
#7786=VECTOR ( 'NONE', #21851, 1000.000000000000000 ) ;
#7790=CARTESIAN_POINT ( 'NONE',  ( 15.18459684427939749, 4.683225679163376398, -2.703237727951164793 ) ) ;
#7791=EDGE_LOOP ( 'NONE', ( #15775, #12960, #15240, #6246 ) ) ;
#7794=EDGE_CURVE ( 'NONE', #4056, #17666, #22002, .T. ) ;
#7808=CARTESIAN_POINT ( 'NONE',  ( 57.00797408584070070, 0.7277374606022131154, 2.435538690626270597 ) ) ;
#7809=CARTESIAN_POINT ( 'NONE',  ( -36.11187263677871329, -3.378578820314678488, 3.972872285093159483 ) ) ;
#7814=ADVANCED_FACE ( 'NONE', ( #21541 ), #24368, .F. ) ;
#7815=CARTESIAN_POINT ( 'NONE',  ( -54.49999999999997868, 1.549999999999999600, -3.332135201338624952 ) ) ;
#7817=CIRCLE ( 'NONE', #9868, 4.100000000000022737 ) ;
#7827=AXIS2_PLACEMENT_3D ( 'NONE', #25890, #26367, #16874 ) ;
#7837=CARTESIAN_POINT ( 'NONE',  ( 15.94709373951294573, -4.924630501335173882, -2.234249019593651742 ) ) ;
#7850=EDGE_CURVE ( 'NONE', #5429, #25588, #22306, .T. ) ;
#7851=ORIENTED_EDGE ( 'NONE', *, *, #19116, .T. ) ;
#7853=VECTOR ( 'NONE', #6805, 1000.000000000000000 ) ;
#7858=ORIENTED_EDGE ( 'NONE', *, *, #12665, .F. ) ;
#7859=CARTESIAN_POINT ( 'NONE',  ( 50.40746642207052730, 1.341874354110782486, -3.874311046529112623 ) ) ;
#7860=ORIENTED_EDGE ( 'NONE', *, *, #11047, .T. ) ;
#7868=CARTESIAN_POINT ( 'NONE',  ( -53.99999999999997868, 0.000000000000000000, 4.700000000000000178 ) ) ;
#7870=EDGE_CURVE ( 'NONE', #30422, #26099, #20274, .T. ) ;
#7877=CIRCLE ( 'NONE', #29609, 3.299999999999999822 ) ;
#7881=CYLINDRICAL_SURFACE ( 'NONE', #29055, 0.9999999999999997780 ) ;
#7886=AXIS2_PLACEMENT_3D ( 'NONE', #2755, #10050, #7522 ) ;
#7888=CONICAL_SURFACE ( 'NONE', #23596, 4.375000000000000000, 0.06758856876739828545 ) ;
#7890=CARTESIAN_POINT ( 'NONE',  ( 16.10624235918716707, 3.046685255238750667, 4.470266847515931730 ) ) ;
#7896=CIRCLE ( 'NONE', #11960, 4.700000000000000178 ) ;
#7909=EDGE_LOOP ( 'NONE', ( #16096, #6216, #13480, #27106 ) ) ;
#7911=CARTESIAN_POINT ( 'NONE',  ( 51.80000000000001847, -0.1421112804877788793, -7.888760782825513275E-16 ) ) ;
#7912=AXIS2_PLACEMENT_3D ( 'NONE', #14523, #14202, #21829 ) ;
#7920=CARTESIAN_POINT ( 'NONE',  ( 50.38701762163459819, 1.088467210617599656, 3.899823238510140122 ) ) ;
#7921=CARTESIAN_POINT ( 'NONE',  ( -36.77443515226921278, -4.926689578693618898, -2.233438676318209470 ) ) ;
#7927=CIRCLE ( 'NONE', #25613, 1.000000000000000000 ) ;
#7929=CIRCLE ( 'NONE', #21083, 1.000000000000000000 ) ;
#7933=EDGE_CURVE ( 'NONE', #30886, #29305, #5673, .T. ) ;
#7939=TOROIDAL_SURFACE ( 'NONE', #10471, 2.549999999999999822, 0.05000000000000000278 ) ;
#7943=CARTESIAN_POINT ( 'NONE',  ( -36.39645873810206211, -0.5233326973448176878, -5.388419908789483515 ) ) ;
#7946=CARTESIAN_POINT ( 'NONE',  ( 15.90468948301723628, -3.705258523861264752, 3.939862169952856874 ) ) ;
#7947=FACE_OUTER_BOUND ( 'NONE', #13889, .T. ) ;
#7948=CARTESIAN_POINT ( 'NONE',  ( -35.85663232820584057, -3.426725943139567576, 3.937891353488737423 ) ) ;
#7949=EDGE_LOOP ( 'NONE', ( #519, #17011, #24384, #10045 ) ) ;
#7950=CARTESIAN_POINT ( 'NONE',  ( 54.50000000000002132, 4.041334437186265510E-16, 3.299999999999999822 ) ) ;
#7953=CARTESIAN_POINT ( 'NONE',  ( 16.10624235918717062, 3.309998894527902635, -4.278958290368501949 ) ) ;
#7957=DIRECTION ( 'NONE',  ( 0.000000000000000000, -1.000000000000000000, 0.000000000000000000 ) ) ;
#7958=CARTESIAN_POINT ( 'NONE',  ( 47.01640678142056373, -4.158733306197476942, 1.045116725612200037 ) ) ;
#7962=ORIENTED_EDGE ( 'NONE', *, *, #6748, .T. ) ;
#7966=CARTESIAN_POINT ( 'NONE',  ( 15.70940947763170570, 4.797009389500183296, -2.498041539401762101 ) ) ;
#7967=VERTEX_POINT ( 'NONE', #17389 ) ;
#7970=CIRCLE ( 'NONE', #15029, 0.09999999999999986677 ) ;
#7972=ORIENTED_EDGE ( 'NONE', *, *, #28613, .T. ) ;
#7973=CARTESIAN_POINT ( 'NONE',  ( 54.49754940158101846, -0.002530889200285349212, 4.297001851131137862 ) ) ;
#7978=VERTEX_POINT ( 'NONE', #933 ) ;
#7980=DIRECTION ( 'NONE',  ( 0.000000000000000000, 0.000000000000000000, -1.000000000000000000 ) ) ;
#7982=DIRECTION ( 'NONE',  ( 0.000000000000000000, 0.4102564102564100201, 0.9119702176296790030 ) ) ;
#7984=CARTESIAN_POINT ( 'NONE',  ( 56.96274124341056222, -0.7308628367038140228, -1.753832840855930719 ) ) ;
#7987=AXIS2_PLACEMENT_3D ( 'NONE', #4748, #19347, #26910 ) ;
#7991=CARTESIAN_POINT ( 'NONE',  ( 15.03925126672132784, 4.804073783693472599, -2.042134687550301919 ) ) ;
#7992=EDGE_CURVE ( 'NONE', #19238, #3444, #12189, .T. ) ;
#7993=DIRECTION ( 'NONE',  ( 0.000000000000000000, 0.000000000000000000, 1.000000000000000000 ) ) ;
#7999=CARTESIAN_POINT ( 'NONE',  ( 50.40000000000001990, 0.6304760106459513791, 3.950000000000022826 ) ) ;
#8001=CARTESIAN_POINT ( 'NONE',  ( 15.90468948301722385, 4.892019442464165202, 2.306425897666068980 ) ) ;
#8004=VERTEX_POINT ( 'NONE', #3141 ) ;
#8006=CIRCLE ( 'NONE', #20154, 4.384222560975607585 ) ;
#8013=CARTESIAN_POINT ( 'NONE',  ( 15.03925126672132961, 2.199885893005915527, 4.939696249117695892 ) ) ;
#8014=EDGE_CURVE ( 'NONE', #7978, #17227, #4087, .T. ) ;
#8015=CARTESIAN_POINT ( 'NONE',  ( 15.17256654081426248, -5.086913989685139192, -1.171642050077601249 ) ) ;
#8018=CARTESIAN_POINT ( 'NONE',  ( 51.75427322675442809, -4.276948333784438283, -0.9210526315789454577 ) ) ;
#8019=CYLINDRICAL_SURFACE ( 'NONE', #9598, 2.600000000000000089 ) ;
#8021=CARTESIAN_POINT ( 'NONE',  ( -36.11692583559977976, -4.018128194441230150, -3.618665885216601819 ) ) ;
#8026=VECTOR ( 'NONE', #27608, 1000.000000000000000 ) ;
#8027=ADVANCED_FACE ( 'NONE', ( #14847 ), #25833, .T. ) ;
#8028=ORIENTED_EDGE ( 'NONE', *, *, #26516, .F. ) ;
#8029=CARTESIAN_POINT ( 'NONE',  ( -35.98994760229851408, -2.686240678227972190, -4.475885392924968897 ) ) ;
#8031=ORIENTED_EDGE ( 'NONE', *, *, #8875, .T. ) ;
#8035=CARTESIAN_POINT ( 'NONE',  ( 48.34316787720665332, -1.211455355144519297, -3.917539841352833285 ) ) ;
#8037=ADVANCED_FACE ( 'NONE', ( #24507 ), #29418, .F. ) ;
#8039=CARTESIAN_POINT ( 'NONE',  ( 54.50000000000002132, 0.000000000000000000, 0.000000000000000000 ) ) ;
#8040=CARTESIAN_POINT ( 'NONE',  ( 57.00221072626734298, -0.7147032416868923654, -1.808443027029684291 ) ) ;
#8043=CARTESIAN_POINT ( 'NONE',  ( 51.80000000000001847, 4.100000000000047606, 2.275957200481583214E-14 ) ) ;
#8056=ADVANCED_FACE ( 'NONE', ( #13246 ), #26137, .T. ) ;
#8058=ORIENTED_EDGE ( 'NONE', *, *, #30999, .T. ) ;
#8059=CARTESIAN_POINT ( 'NONE',  ( 15.03925126672132784, -2.525801270006312382, 4.794550352686321126 ) ) ;
#8062=EDGE_CURVE ( 'NONE', #9539, #2309, #13566, .T. ) ;
#8065=COLOUR_RGB ( '', 0.40784314, 0.44705882, 0.49803922) ;
#8066=CARTESIAN_POINT ( 'NONE',  ( -36.04518387042617888, 0.7747498539026829167, 5.363501450340917742 ) ) ;
#8073=CARTESIAN_POINT ( 'NONE',  ( 57.01550456668461209, 0.7366124869942373143, -2.429953032873097829 ) ) ;
#8076=VERTEX_POINT ( 'NONE', #21029 ) ;
#8078=PLANE ( 'NONE',  #4242 ) ;
#8084=CARTESIAN_POINT ( 'NONE',  ( 50.30848954602731027, 1.391941090707534689, 3.850000000000023181 ) ) ;
#8093=CARTESIAN_POINT ( 'NONE',  ( 47.08691981199204690, -4.178911716362186723, -1.000646358242008205 ) ) ;
#8095=CARTESIAN_POINT ( 'NONE',  ( 15.86395258069112124, -0.7247683022689926924, 5.358970532132270925 ) ) ;
#8100=FACE_OUTER_BOUND ( 'NONE', #10395, .T. ) ;
#8101=DIRECTION ( 'NONE',  ( 0.000000000000000000, 0.000000000000000000, -1.000000000000000000 ) ) ;
#8104=CARTESIAN_POINT ( 'NONE',  ( -44.49999999999997868, 1.499999999999999556, 4.029888335921975262 ) ) ;
#8106=CARTESIAN_POINT ( 'NONE',  ( 15.87128154250932610, 2.562020839648826431, -4.763023844700913223 ) ) ;
#8110=VERTEX_POINT ( 'NONE', #4077 ) ;
#8113=EDGE_CURVE ( 'NONE', #1709, #30274, #1103, .T. ) ;
#8119=DIRECTION ( 'NONE',  ( -1.000000000000000000, -0.000000000000000000, 0.000000000000000000 ) ) ;
#8120=VERTEX_POINT ( 'NONE', #28306 ) ;
#8124=ORIENTED_EDGE ( 'NONE', *, *, #4153, .F. ) ;
#8126=CARTESIAN_POINT ( 'NONE',  ( 48.40000000000001990, -4.899999999999999467, 4.100000000000022737 ) ) ;
#8128=ORIENTED_EDGE ( 'NONE', *, *, #2418, .T. ) ;
#8132=DIRECTION ( 'NONE',  ( 0.000000000000000000, 0.000000000000000000, -1.000000000000000000 ) ) ;
#8134=DIRECTION ( 'NONE',  ( 1.000000000000000000, 0.000000000000000000, 0.000000000000000000 ) ) ;
#8137=AXIS2_PLACEMENT_3D ( 'NONE', #8350, #15324, #17558 ) ;
#8143=CARTESIAN_POINT ( 'NONE',  ( -54.49998431799114940, 1.548747819918198987, 3.331336553795240185 ) ) ;
#8144=EDGE_CURVE ( 'NONE', #29040, #23306, #2623, .T. ) ;
#8154=ORIENTED_EDGE ( 'NONE', *, *, #4524, .T. ) ;
#8156=AXIS2_PLACEMENT_3D ( 'NONE', #21953, #4529, #4833 ) ;
#8157=ORIENTED_EDGE ( 'NONE', *, *, #9126, .F. ) ;
#8158=LINE ( 'NONE', #5780, #2018 ) ;
#8161=VERTEX_POINT ( 'NONE', #11526 ) ;
#8164=ORIENTED_EDGE ( 'NONE', *, *, #19725, .F. ) ;
#8166=CARTESIAN_POINT ( 'NONE',  ( 15.76675455518220303, -5.174628573245093399, -1.572974725650858385 ) ) ;
#8178=CIRCLE ( 'NONE', #27881, 1.000000000000000000 ) ;
#8184=EDGE_CURVE ( 'NONE', #18396, #14402, #8178, .T. ) ;
#8185=CARTESIAN_POINT ( 'NONE',  ( 48.30000000000001847, 2.428612866367529932E-14, 0.000000000000000000 ) ) ;
#8187=CARTESIAN_POINT ( 'NONE',  ( 15.03925126672132961, -1.123735532908281431, -5.289358697221548056 ) ) ;
#8188=CARTESIAN_POINT ( 'NONE',  ( -36.11187263677951620, -5.068523420888918274, 1.228242390833657049 ) ) ;
#8190=CARTESIAN_POINT ( 'NONE',  ( 50.50000000000002132, -0.6304760106459033064, -3.950000000000021938 ) ) ;
#8191=ORIENTED_EDGE ( 'NONE', *, *, #27718, .T. ) ;
#8193=CARTESIAN_POINT ( 'NONE',  ( 57.01635142493560693, -0.7373792903891465134, -1.789496335369930025 ) ) ;
#8194=ORIENTED_EDGE ( 'NONE', *, *, #17120, .F. ) ;
#8196=CYLINDRICAL_SURFACE ( 'NONE', #386, 1.000000000000000000 ) ;
#8204=CARTESIAN_POINT ( 'NONE',  ( -36.89831264271880684, -2.941172302009062545, 4.539591111929643041 ) ) ;
#8208=CARTESIAN_POINT ( 'NONE',  ( 15.03925126672122836, 2.199885893005901316, 4.939696249117701221 ) ) ;
#8216=EDGE_CURVE ( 'NONE', #13291, #17296, #15798, .T. ) ;
#8223=ORIENTED_EDGE ( 'NONE', *, *, #16848, .T. ) ;
#8240=CARTESIAN_POINT ( 'NONE',  ( 48.47204894654066010, -1.409900792624738886, -3.850000304694921827 ) ) ;
#8242=ADVANCED_FACE ( 'NONE', ( #14348 ), #23723, .F. ) ;
#8243=CARTESIAN_POINT ( 'NONE',  ( 57.04413099161754985, -0.7497394063391640273, -2.421432380119032501 ) ) ;
#8248=DIRECTION ( 'NONE',  ( 1.000000000000000000, 1.786976680021873984E-16, 2.459562394685737870E-16 ) ) ;
#8249=CARTESIAN_POINT ( 'NONE',  ( 51.80000000000001847, -3.726179070414207928, -1.100000000000000089 ) ) ;
#8250=ORIENTED_EDGE ( 'NONE', *, *, #11931, .F. ) ;
#8251=EDGE_CURVE ( 'NONE', #20165, #29437, #17066, .T. ) ;
#8252=CARTESIAN_POINT ( 'NONE',  ( 50.33814819168215138, -1.426738236278548566, -3.843750512866276559 ) ) ;
#8255=CARTESIAN_POINT ( 'NONE',  ( 15.67083574136752411, 2.849134329833903578, -4.601168830303363322 ) ) ;
#8257=CARTESIAN_POINT ( 'NONE',  ( 57.02185466405004632, 0.7499999999999981126, 2.421260014775926006 ) ) ;
#8259=ORIENTED_EDGE ( 'NONE', *, *, #2046, .T. ) ;
#8261=CARTESIAN_POINT ( 'NONE',  ( 47.03864569166055531, -4.169908074913990070, 1.021033875312352235 ) ) ;
#8263=DIRECTION ( 'NONE',  ( 0.000000000000000000, 0.000000000000000000, 1.000000000000000000 ) ) ;
#8265=CARTESIAN_POINT ( 'NONE',  ( 15.71019289815287223, 3.857619034241809075, -3.790808625283980771 ) ) ;
#8266=CARTESIAN_POINT ( 'NONE',  ( -44.49999999999999289, 0.000000000000000000, 4.299999999999998046 ) ) ;
#8268=DIRECTION ( 'NONE',  ( 0.000000000000000000, -1.517883041479702421E-14, 1.000000000000000000 ) ) ;
#8271=DIRECTION ( 'NONE',  ( 1.000000000000000000, 0.000000000000000000, 0.000000000000000000 ) ) ;
#8273=CARTESIAN_POINT ( 'NONE',  ( -35.85663232820584057, -3.056483311920853208, -4.206888370749738648 ) ) ;
#8288=LINE ( 'NONE', #4007, #26104 ) ;
#8291=VECTOR ( 'NONE', #8680, 1000.000000000000000 ) ;
#8295=ORIENTED_EDGE ( 'NONE', *, *, #19916, .F. ) ;
#8301=ORIENTED_EDGE ( 'NONE', *, *, #8777, .F. ) ;
#8303=AXIS2_PLACEMENT_3D ( 'NONE', #27184, #5494, #10091 ) ;
#8317=ADVANCED_FACE ( 'NONE', ( #21358 ), #14203, .T. ) ;
#8318=CARTESIAN_POINT ( 'NONE',  ( 48.50000000000002132, 1.391941090707534023, 3.850000000000022737 ) ) ;
#8319=EDGE_CURVE ( 'NONE', #13545, #29070, #27386, .T. ) ;
#8323=DIRECTION ( 'NONE',  ( 0.000000000000000000, 0.2745098039215673746, 0.9615843008030769967 ) ) ;
#8330=EDGE_LOOP ( 'NONE', ( #4294, #1028, #11886, #9103 ) ) ;
#8332=DIRECTION ( 'NONE',  ( 0.000000000000000000, 1.000000000000000000, 0.000000000000000000 ) ) ;
#8334=CARTESIAN_POINT ( 'NONE',  ( 15.56401610563845850, -1.027070083875938566, -5.312835761376674348 ) ) ;
#8338=CARTESIAN_POINT ( 'NONE',  ( -54.49999999999997868, 1.549999999999999600, -3.300094695611021312 ) ) ;
#8339=ORIENTED_EDGE ( 'NONE', *, *, #10194, .F. ) ;
#8350=CARTESIAN_POINT ( 'NONE',  ( 48.30000000000001847, -0.6304760106459033064, -3.950000000000022826 ) ) ;
#8353=VERTEX_POINT ( 'NONE', #14036 ) ;
#8354=ADVANCED_FACE ( 'NONE', ( #30984 ), #24112, .T. ) ;
#8356=CARTESIAN_POINT ( 'NONE',  ( 15.41217651307625225, 2.840625797033981215, 4.363718033548180664 ) ) ;
#8358=CARTESIAN_POINT ( 'NONE',  ( 51.80000000000001847, 2.428612866367529932E-14, 0.000000000000000000 ) ) ;
#8361=DIRECTION ( 'NONE',  ( -1.000000000000000000, -2.586136946169074517E-16, 0.000000000000000000 ) ) ;
#8369=CARTESIAN_POINT ( 'NONE',  ( 48.43418025728714582, 1.399739523915438211, 3.853780793998481169 ) ) ;
#8373=ORIENTED_EDGE ( 'NONE', *, *, #7690, .F. ) ;
#8377=ORIENTED_EDGE ( 'NONE', *, *, #10719, .T. ) ;
#8381=AXIS2_PLACEMENT_3D ( 'NONE', #9810, #14854, #5061 ) ;
#8390=CARTESIAN_POINT ( 'NONE',  ( 47.10000000000002274, -4.179189514726506793, -1.000000000000000000 ) ) ;
#8392=CARTESIAN_POINT ( 'NONE',  ( 58.45000000000001705, 0.8000000000000000444, -1.778341924377873751 ) ) ;
#8406=VECTOR ( 'NONE', #12367, 1000.000000000000000 ) ;
#8408=( BOUNDED_SURFACE ( )  B_SPLINE_SURFACE ( 3, 2, ( 
 ( #20561, #6139, #8508 ),
 ( #13384, #18188, #4377 ),
 ( #14027, #26535, #29073 ),
 ( #16894, #11519, #30978 ),
 ( #28772, #14507, #6923 ),
 ( #9296, #23716, #2007 ),
 ( #21196, #16745, #21495 ),
 ( #2158, #24180, #16592 ),
 ( #19283, #26233, #13855 ),
 ( #30826, #26388, #11821 ) ),
 .UNSPECIFIED., .F., .F., .F. ) 
 B_SPLINE_SURFACE_WITH_KNOTS ( ( 4, 2, 2, 2, 4 ),
 ( 3, 3 ),
 ( 0.0002526260074104870901, 0.0003606909493797115550, 0.0004687558913489360741, 0.0006848857752873850581, 0.001117145543164283026 ),
 ( 0.000000000000000000, 1.000000000000000000 ),
 .UNSPECIFIED. ) 
 GEOMETRIC_REPRESENTATION_ITEM ( )  RATIONAL_B_SPLINE_SURFACE ( (
 ( 1.000000000000000000, 0.9842509842511785179, 1.000000000000000000),
 ( 1.000000000000000000, 0.9838268088398964828, 1.000000000000000000),
 ( 1.000000000000000000, 0.9731519947952215199, 1.000000000000000000),
 ( 1.000000000000000000, 0.9499473078865533493, 1.000000000000000000),
 ( 1.000000000000000000, 0.9371632344323698183, 1.000000000000000000),
 ( 1.000000000000000000, 0.8981767195495007350, 1.000000000000000000),
 ( 1.000000000000000000, 0.8714317066438488357, 1.000000000000000000),
 ( 1.000000000000000000, 0.7945716934681560373, 1.000000000000000000),
 ( 1.000000000000000000, 0.7462340517456401701, 1.000000000000000000),
 ( 1.000000000000000000, 0.7071067811865505703, 1.000000000000000000) ) ) 
 REPRESENTATION_ITEM ( '' )  SURFACE ( )  );
#8409=CARTESIAN_POINT ( 'NONE',  ( 50.36079629521400847, -1.278211010209444387, -3.870212229389975445 ) ) ;
#8411=CARTESIAN_POINT ( 'NONE',  ( -36.79682133506351960, 2.710596767400097473, -4.680923748382986638 ) ) ;
#8414=CARTESIAN_POINT ( 'NONE',  ( 15.03925126672123369, -5.377732432866647372, 0.5657657256215353758 ) ) ;
#8417=CARTESIAN_POINT ( 'NONE',  ( 47.00000000000002132, -4.131056160354152240, 1.099999999999999867 ) ) ;
#8423=FACE_OUTER_BOUND ( 'NONE', #17024, .T. ) ;
#8430=CARTESIAN_POINT ( 'NONE',  ( -35.85663232820584057, 4.945493884734801782, -1.606888370749687933 ) ) ;
#8432=ORIENTED_EDGE ( 'NONE', *, *, #261, .F. ) ;
#8440=DIRECTION ( 'NONE',  ( 1.000000000000000000, -0.000000000000000000, -0.000000000000000000 ) ) ;
#8441=EDGE_CURVE ( 'NONE', #3969, #6711, #5144, .T. ) ;
#8442=CARTESIAN_POINT ( 'NONE',  ( 47.00000000000002132, 2.428612866367529932E-14, 0.000000000000000000 ) ) ;
#8445=AXIS2_PLACEMENT_3D ( 'NONE', #20439, #30064, #25327 ) ;
#8449=FACE_OUTER_BOUND ( 'NONE', #2121, .T. ) ;
#8451=ADVANCED_FACE ( 'NONE', ( #30158 ), #15610, .T. ) ;
#8453=CARTESIAN_POINT ( 'NONE',  ( 48.37784963381696457, -1.308847734660468332, 3.885629509820973659 ) ) ;
#8455=DIRECTION ( 'NONE',  ( 1.000000000000000000, -0.000000000000000000, 0.000000000000000000 ) ) ;
#8458=AXIS2_PLACEMENT_3D ( 'NONE', #17378, #2523, #26744 ) ;
#8470=ORIENTED_EDGE ( 'NONE', *, *, #6539, .T. ) ;
#8471=DIRECTION ( 'NONE',  ( 0.000000000000000000, -1.000000000000000000, 0.000000000000000000 ) ) ;
#8486=CARTESIAN_POINT ( 'NONE',  ( -35.85663232820584057, 5.086913985776128300, 1.171642053949150331 ) ) ;
#8492=ORIENTED_EDGE ( 'NONE', *, *, #11720, .T. ) ;
#8497=EDGE_LOOP ( 'NONE', ( #19907, #4320, #607, #16893 ) ) ;
#8500=CARTESIAN_POINT ( 'NONE',  ( -35.85663232820584057, 4.018128179617486140, 3.618665901676695995 ) ) ;
#8501=CARTESIAN_POINT ( 'NONE',  ( 15.03925126672132784, 4.804073783693426414, 2.042134687550409833 ) ) ;
#8503=EDGE_CURVE ( 'NONE', #26007, #26067, #6151, .T. ) ;
#8506=CARTESIAN_POINT ( 'NONE',  ( 57.02075198358709684, -0.7405530952691583568, -1.786721332245943428 ) ) ;
#8508=CARTESIAN_POINT ( 'NONE',  ( 50.29999999999649418, 1.426739617988885822, 3.843749999997122746 ) ) ;
#8510=EDGE_CURVE ( 'NONE', #17741, #13619, #10842, .T. ) ;
#8513=CARTESIAN_POINT ( 'NONE',  ( -36.56390771145525775, 5.205077242910716606, -1.471673150993946244 ) ) ;
#8521=CARTESIAN_POINT ( 'NONE',  ( 15.17256654081426070, -2.686240678228060119, 4.475885392924785933 ) ) ;
#8523=DIRECTION ( 'NONE',  ( 1.000000000000000000, 0.000000000000000000, -0.000000000000000000 ) ) ;
#8526=CARTESIAN_POINT ( 'NONE',  ( 48.43389689255278796, 1.399562922973069057, -3.853849143137397792 ) ) ;
#8532=DIRECTION ( 'NONE',  ( 2.459562394685743786E-16, -0.9510565162951521989, -0.3090169943749515591 ) ) ;
#8533=VERTEX_POINT ( 'NONE', #3714 ) ;
#8535=DIRECTION ( 'NONE',  ( 1.000000000000000000, 2.586136946169074517E-16, -0.000000000000000000 ) ) ;
#8549=DIRECTION ( 'NONE',  ( 1.000000000000000000, 2.586136946169074517E-16, -0.000000000000000000 ) ) ;
#8551=CARTESIAN_POINT ( 'NONE',  ( 15.48609859788809473, -0.1138661108244446996, 5.199999999057606459 ) ) ;
#8556=DIRECTION ( 'NONE',  ( 0.000000000000000000, 0.000000000000000000, 1.000000000000000000 ) ) ;
#8559=DIRECTION ( 'NONE',  ( 2.586136946169074517E-16, -1.000000000000000000, 0.000000000000000000 ) ) ;
#8562=CARTESIAN_POINT ( 'NONE',  ( 50.50000000000001421, -0.6462379109120512943, -4.048750000000022276 ) ) ;
#8566=CARTESIAN_POINT ( 'NONE',  ( 57.05000000000001137, 0.7500000000000000000, 2.490438859776672231 ) ) ;
#8571=ORIENTED_EDGE ( 'NONE', *, *, #131, .F. ) ;
#8572=DIRECTION ( 'NONE',  ( -1.000000000000000000, 0.000000000000000000, 0.000000000000000000 ) ) ;
#8579=VECTOR ( 'NONE', #29757, 1000.000000000000000 ) ;
#8582=ORIENTED_EDGE ( 'NONE', *, *, #27375, .F. ) ;
#8583=CARTESIAN_POINT ( 'NONE',  ( 57.04071222441830713, 0.7791709056946051204, -1.732885792771923672 ) ) ;
#8585=ORIENTED_EDGE ( 'NONE', *, *, #23175, .T. ) ;
#8586=AXIS2_PLACEMENT_3D ( 'NONE', #27788, #8471, #12587 ) ;
#8594=CIRCLE ( 'NONE', #24784, 4.000000000000022204 ) ;
#8599=DIRECTION ( 'NONE',  ( 0.000000000000000000, 0.000000000000000000, -1.000000000000000000 ) ) ;
#8622=ORIENTED_EDGE ( 'NONE', *, *, #21117, .F. ) ;
#8623=EDGE_CURVE ( 'NONE', #27956, #30697, #7676, .T. ) ;
#8624=CARTESIAN_POINT ( 'NONE',  ( 46.99358615024069508, -4.235076411888983650, -1.097987773005456580 ) ) ;
#8630=CARTESIAN_POINT ( 'NONE',  ( 57.04306286658350444, 0.7495164233357125561, -1.778776689171566172 ) ) ;
#8634=CARTESIAN_POINT ( 'NONE',  ( 57.00000000000001421, 0.7500000000000000000, 3.499999999999999556 ) ) ;
#8637=EDGE_LOOP ( 'NONE', ( #27854, #16216, #9992, #1029 ) ) ;
#8638=DIRECTION ( 'NONE',  ( 0.000000000000000000, 0.000000000000000000, -1.000000000000000000 ) ) ;
#8639=ORIENTED_EDGE ( 'NONE', *, *, #11931, .T. ) ;
#8640=EDGE_CURVE ( 'NONE', #10683, #3969, #23837, .T. ) ;
#8648=EDGE_CURVE ( 'NONE', #22384, #9517, #26399, .T. ) ;
#8653=ORIENTED_EDGE ( 'NONE', *, *, #1134, .F. ) ;
#8654=PLANE ( 'NONE',  #17609 ) ;
#8657=ORIENTED_EDGE ( 'NONE', *, *, #16190, .T. ) ;
#8658=CARTESIAN_POINT ( 'NONE',  ( -36.56242893520593640, 5.074157625981714048, -1.874066637979897143 ) ) ;
#8665=ADVANCED_FACE ( 'NONE', ( #16716 ), #18930, .T. ) ;
#8670=CARTESIAN_POINT ( 'NONE',  ( 58.50000000000001421, 0.8000000000000000444, 2.471260002560649927 ) ) ;
#8672=CIRCLE ( 'NONE', #3130, 0.09999999999999982514 ) ;
#8676=CARTESIAN_POINT ( 'NONE',  ( 48.42250533816334013, 1.328329461116622090, 3.879000873601222477 ) ) ;
#8677=DIRECTION ( 'NONE',  ( -0.9977167620779625601, -0.06753712067201329827, 0.000000000000000000 ) ) ;
#8680=DIRECTION ( 'NONE',  ( -1.000000000000000000, -5.172273892338149033E-16, 0.000000000000000000 ) ) ;
#8681=AXIS2_PLACEMENT_3D ( 'NONE', #28490, #23430, #16147 ) ;
#8687=CARTESIAN_POINT ( 'NONE',  ( 58.45000000000001705, 0.8000000000000001554, 1.778341924377873973 ) ) ;
#8694=DIRECTION ( 'NONE',  ( 0.000000000000000000, 1.000000000000000000, 0.000000000000000000 ) ) ;
#8700=DIRECTION ( 'NONE',  ( -0.000000000000000000, 1.000000000000000000, 1.532429380227459806E-15 ) ) ;
#8706=FACE_OUTER_BOUND ( 'NONE', #13374, .T. ) ;
#8707=LINE ( 'NONE', #18392, #19413 ) ;
#8709=DIRECTION ( 'NONE',  ( 0.000000000000000000, 0.000000000000000000, -1.000000000000000000 ) ) ;
#8711=PLANE ( 'NONE',  #6450 ) ;
#8714=DIRECTION ( 'NONE',  ( 0.000000000000000000, -1.000000000000000000, -1.532429380227459806E-15 ) ) ;
#8715=EDGE_CURVE ( 'NONE', #4862, #16826, #18773, .T. ) ;
#8716=ORIENTED_EDGE ( 'NONE', *, *, #14220, .F. ) ;
#8718=ORIENTED_EDGE ( 'NONE', *, *, #147, .T. ) ;
#8719=CARTESIAN_POINT ( 'NONE',  ( 16.08093158123429234, 3.408535483610603656, -4.200031884472213761 ) ) ;
#8729=( BOUNDED_SURFACE ( )  B_SPLINE_SURFACE ( 3, 2, ( 
 ( #2515, #29099, #7413 ),
 ( #7109, #278, #19158 ),
 ( #27018, #31160, #24038 ),
 ( #14690, #29259, #26738 ),
 ( #14831, #5032, #2347 ),
 ( #5327, #14990, #2180 ),
 ( #24350, #4874, #2663 ),
 ( #21695, #7250, #21984 ),
 ( #9945, #9495, #28797 ),
 ( #16769, #12013, #28942 ),
 ( #16918, #26561, #14539 ),
 ( #19621, #24204, #30018 ),
 ( #25281, #20243, #12766 ),
 ( #8334, #27491, #18008 ),
 ( #739, #27657, #6130 ),
 ( #8187, #17700, #5985 ) ),
 .UNSPECIFIED., .F., .F., .F. ) 
 B_SPLINE_SURFACE_WITH_KNOTS ( ( 4, 2, 2, 2, 2, 2, 2, 4 ),
 ( 3, 3 ),
 ( 0.001780502285214203163, 0.002558945925323785446, 0.002753556835351180909, 0.002948167745378576371, 0.003337389565433367296, 0.003726611385488158654, 0.004115833205542950013, 0.004894276845652531863 ),
 ( 0.000000000000000000, 1.000000000000000000 ),
 .UNSPECIFIED. ) 
 GEOMETRIC_REPRESENTATION_ITEM ( )  RATIONAL_B_SPLINE_SURFACE ( (
 ( 1.000000000000000000, 0.9418517008537237167, 1.000000000000000000),
 ( 1.000000000000000000, 0.9417987965885079582, 1.000000000000000000),
 ( 1.000000000000000000, 0.9418198861734077276, 1.000000000000000000),
 ( 1.000000000000000000, 0.9434060303845566153, 1.000000000000000000),
 ( 1.000000000000000000, 0.9437939819948232278, 1.000000000000000000),
 ( 1.000000000000000000, 0.9445989566712728047, 1.000000000000000000),
 ( 1.000000000000000000, 0.9450169930049754363, 1.000000000000000000),
 ( 1.000000000000000000, 0.9461610507673754444, 1.000000000000000000),
 ( 1.000000000000000000, 0.9467217966427202702, 1.000000000000000000),
 ( 1.000000000000000000, 0.9467345476124352510, 1.000000000000000000),
 ( 1.000000000000000000, 0.9461964028052860520, 1.000000000000000000),
 ( 1.000000000000000000, 0.9446801822473911425, 1.000000000000000000),
 ( 1.000000000000000000, 0.9437582546536744665, 1.000000000000000000),
 ( 1.000000000000000000, 0.9418129560295230851, 1.000000000000000000),
 ( 1.000000000000000000, 0.9418016889777798273, 1.000000000000000000),
 ( 1.000000000000000000, 0.9418517008537228286, 1.000000000000000000) ) ) 
 REPRESENTATION_ITEM ( '' )  SURFACE ( )  );
#8732=CIRCLE ( 'NONE', #7240, 30.00000000000000000 ) ;
#8733=LINE ( 'NONE', #25692, #9423 ) ;
#8734=FACE_OUTER_BOUND ( 'NONE', #22474, .T. ) ;
#8735=EDGE_CURVE ( 'NONE', #15593, #616, #1978, .T. ) ;
#8741=DIRECTION ( 'NONE',  ( 0.000000000000000000, -1.000000000000000000, -1.224646799147352961E-16 ) ) ;
#8747=( NAMED_UNIT ( * ) SI_UNIT ( $, .STERADIAN. ) SOLID_ANGLE_UNIT ( ) );
#8748=AXIS2_PLACEMENT_3D ( 'NONE', #11693, #21373, #14536 ) ;
#8749=DIRECTION ( 'NONE',  ( 1.000000000000000000, 0.000000000000000000, 0.000000000000000000 ) ) ;
#8761=DIRECTION ( 'NONE',  ( 1.000000000000000000, 0.000000000000000000, 0.000000000000000000 ) ) ;
#8763=DIRECTION ( 'NONE',  ( 0.000000000000000000, -0.000000000000000000, 1.000000000000000000 ) ) ;
#8767=CARTESIAN_POINT ( 'NONE',  ( 36.50000000000002132, 0.7794871794871797155, -1.732743413496390161 ) ) ;
#8777=EDGE_CURVE ( 'NONE', #7978, #4176, #14508, .T. ) ;
#8789=CARTESIAN_POINT ( 'NONE',  ( 51.80000000000001847, 2.478823385132571406E-14, 4.100000000000022737 ) ) ;
#8792=DIRECTION ( 'NONE',  ( 0.000000000000000000, 0.000000000000000000, -1.000000000000000000 ) ) ;
#8795=ORIENTED_EDGE ( 'NONE', *, *, #12665, .T. ) ;
#8798=PLANE ( 'NONE',  #11005 ) ;
#8801=AXIS2_PLACEMENT_3D ( 'NONE', #25628, #16299, #4246 ) ;
#8802=CARTESIAN_POINT ( 'NONE',  ( -36.38139716712170468, 5.370189181195062389, -0.6649548426257293476 ) ) ;
#8803=ADVANCED_FACE ( 'NONE', ( #26965, #22089 ), #681, .T. ) ;
#8810=DIRECTION ( 'NONE',  ( 1.000000000000000000, 2.586136946169074517E-16, -0.000000000000000000 ) ) ;
#8818=CARTESIAN_POINT ( 'NONE',  ( -35.98994760229916068, -0.4576450652446866219, 5.200000002521323772 ) ) ;
#8819=CARTESIAN_POINT ( 'NONE',  ( 15.03925126672132961, 3.426725943139601327, -3.937891353488703228 ) ) ;
#8820=ORIENTED_EDGE ( 'NONE', *, *, #29245, .T. ) ;
#8826=CARTESIAN_POINT ( 'NONE',  ( 56.99999999998442490, 0.7044205509462206916, -2.449516039469794570 ) ) ;
#8830=FACE_BOUND ( 'NONE', #28418, .T. ) ;
#8831=FACE_OUTER_BOUND ( 'NONE', #18144, .T. ) ;
#8835=EDGE_CURVE ( 'NONE', #616, #6201, #21324, .T. ) ;
#8844=CARTESIAN_POINT ( 'NONE',  ( 57.02678890911435872, -0.7442859487862443224, 1.783438914669892128 ) ) ;
#8863=CARTESIAN_POINT ( 'NONE',  ( 47.00000000000002132, -3.726179070414207928, -1.710435481158852467 ) ) ;
#8866=CARTESIAN_POINT ( 'NONE',  ( 15.44259799936803468, -5.012895491272645998, 1.399447560527413925 ) ) ;
#8867=VECTOR ( 'NONE', #29532, 1000.000000000000000 ) ;
#8868=ORIENTED_EDGE ( 'NONE', *, *, #23755, .T. ) ;
#8872=ORIENTED_EDGE ( 'NONE', *, *, #13024, .T. ) ;
#8875=EDGE_CURVE ( 'NONE', #1101, #27607, #603, .T. ) ;
#8882=ORIENTED_EDGE ( 'NONE', *, *, #24868, .T. ) ;
#8884=EDGE_LOOP ( 'NONE', ( #10902, #26807, #5141, #7105 ) ) ;
#8886=VERTEX_POINT ( 'NONE', #21075 ) ;
#8888=VECTOR ( 'NONE', #5574, 1000.000000000000000 ) ;
#8889=CARTESIAN_POINT ( 'NONE',  ( 57.02825620192501077, -0.8138444489294278661, 2.469346200785457413 ) ) ;
#8895=AXIS2_PLACEMENT_3D ( 'NONE', #18270, #13320, #27442 ) ;
#8899=CARTESIAN_POINT ( 'NONE',  ( 47.00000000000002132, 1.426739617975221641, 3.843750000000023093 ) ) ;
#8902=CARTESIAN_POINT ( 'NONE',  ( 15.03925126672122303, 5.377732432866646484, -0.5657657256215100627 ) ) ;
#8904=CARTESIAN_POINT ( 'NONE',  ( 57.05000000000001847, 0.7500000000000000000, -2.421260002560650104 ) ) ;
#8908=DIRECTION ( 'NONE',  ( 1.000000000000000000, 0.000000000000000000, 0.000000000000000000 ) ) ;
#8909=CARTESIAN_POINT ( 'NONE',  ( 50.40000000000001279, -0.6304760106459028624, 3.950000000000022826 ) ) ;
#8913=VERTEX_POINT ( 'NONE', #9025 ) ;
#8917=EDGE_LOOP ( 'NONE', ( #30908, #4664, #20107, #2395 ) ) ;
#8921=ORIENTED_EDGE ( 'NONE', *, *, #29386, .T. ) ;
#8922=TOROIDAL_SURFACE ( 'NONE', #19054, 4.000000000000022204, 0.1000000000000000056 ) ;
#8934=CARTESIAN_POINT ( 'NONE',  ( 47.00000000000002132, -4.227689052994015206, -1.125730994152046582 ) ) ;
#8936=CARTESIAN_POINT ( 'NONE',  ( 56.95206911348624601, -0.7375298837344119729, -2.493227876267903653 ) ) ;
#8942=DIRECTION ( 'NONE',  ( -1.000000000000000000, 0.000000000000000000, 0.000000000000000000 ) ) ;
#8943=CIRCLE ( 'NONE', #26659, 0.4576450603546982632 ) ;
#8949=CARTESIAN_POINT ( 'NONE',  ( 15.03925126672132961, 4.018128179617565188, -3.618665901676623164 ) ) ;
#8951=CARTESIAN_POINT ( 'NONE',  ( -35.85663232820583346, -3.817150320980684075, 2.203324261490539282 ) ) ;
#8955=VERTEX_POINT ( 'NONE', #4260 ) ;
#8957=ORIENTED_EDGE ( 'NONE', *, *, #12313, .T. ) ;
#8963=CARTESIAN_POINT ( 'NONE',  ( -36.30424252565907750, 2.966783028120403731, 4.272059443775344079 ) ) ;
#8966=CARTESIAN_POINT ( 'NONE',  ( 51.80000000000001847, -0.2842225609755594795, -1.577752156565102655E-15 ) ) ;
#8967=AXIS2_PLACEMENT_3D ( 'NONE', #30862, #9793, #28483 ) ;
#8972=CIRCLE ( 'NONE', #22646, 0.05000000000000009298 ) ;
#8974=CARTESIAN_POINT ( 'NONE',  ( 15.03925126672132784, 4.683225679163323996, 2.703237727951258051 ) ) ;
#8976=CARTESIAN_POINT ( 'NONE',  ( -35.85663232820584057, 3.056483311920880297, -4.206888370749704897 ) ) ;
#8977=ORIENTED_EDGE ( 'NONE', *, *, #31061, .F. ) ;
#8978=CARTESIAN_POINT ( 'NONE',  ( -36.76447480099743359, 4.924630501335110822, -2.234249019593746333 ) ) ;
#8981=AXIS2_PLACEMENT_3D ( 'NONE', #4374, #16110, #9142 ) ;
#8982=CARTESIAN_POINT ( 'NONE',  ( 46.90000000000001990, -4.131056160354152240, 1.099999999999999867 ) ) ;
#9001=VERTEX_POINT ( 'NONE', #14081 ) ;
#9003=ORIENTED_EDGE ( 'NONE', *, *, #25259, .F. ) ;
#9004=FACE_OUTER_BOUND ( 'NONE', #13257, .T. ) ;
#9011=CARTESIAN_POINT ( 'NONE',  ( 54.40000000000001990, 1.734723475976807094E-15, 0.000000000000000000 ) ) ;
#9012=CARTESIAN_POINT ( 'NONE',  ( -35.85663232820583346, -4.683225679163361299, 2.703237727951226077 ) ) ;
#9013=ORIENTED_EDGE ( 'NONE', *, *, #18150, .F. ) ;
#9015=EDGE_CURVE ( 'NONE', #20639, #3532, #1902, .T. ) ;
#9018=AXIS2_PLACEMENT_3D ( 'NONE', #25987, #9060, #11596 ) ;
#9021=CARTESIAN_POINT ( 'NONE',  ( -54.46895629856896903, 1.503487923075246480, -4.032311158269683560 ) ) ;
#9022=ORIENTED_EDGE ( 'NONE', *, *, #20264, .F. ) ;
#9024=EDGE_CURVE ( 'NONE', #13995, #26742, #20196, .T. ) ;
#9025=CARTESIAN_POINT ( 'NONE',  ( 50.50000000000002132, 2.428612866367529932E-14, -4.100000000000022737 ) ) ;
#9026=CARTESIAN_POINT ( 'NONE',  ( -36.68133364217572989, 2.563573972737328788, -4.761506352252359520 ) ) ;
#9029=CARTESIAN_POINT ( 'NONE',  ( 16.00221665700883378, -0.5763363385013805518, -5.380853831843025681 ) ) ;
#9030=DIRECTION ( 'NONE',  ( -1.000000000000000000, -2.586136946169074517E-16, 0.000000000000000000 ) ) ;
#9032=EDGE_CURVE ( 'NONE', #28342, #17261, #22637, .T. ) ;
#9036=CARTESIAN_POINT ( 'NONE',  ( 50.32627973729707094, -1.373706569044463199, -3.853361913240786141 ) ) ;
#9037=ORIENTED_EDGE ( 'NONE', *, *, #27945, .F. ) ;
#9043=CARTESIAN_POINT ( 'NONE',  ( -36.42771574642716104, 5.277035221755925321, 1.205525476379240679 ) ) ;
#9044=CARTESIAN_POINT ( 'NONE',  ( 16.10624235918717773, -5.192953935288615597, 1.516181439821707500 ) ) ;
#9047=CARTESIAN_POINT ( 'NONE',  ( 48.30000000000001847, 0.6462379109121000331, 4.048750000000023164 ) ) ;
#9060=DIRECTION ( 'NONE',  ( 0.000000000000000000, 0.000000000000000000, 1.000000000000000000 ) ) ;
#9072=EDGE_CURVE ( 'NONE', #28914, #17227, #6205, .T. ) ;
#9074=DIRECTION ( 'NONE',  ( -1.000000000000000000, -0.000000000000000000, -0.000000000000000000 ) ) ;
#9075=CARTESIAN_POINT ( 'NONE',  ( 57.03253626007334987, 0.8141194241917997232, 2.469252834999610791 ) ) ;
#9077=AXIS2_PLACEMENT_3D ( 'NONE', #5382, #26188, #7614 ) ;
#9079=CARTESIAN_POINT ( 'NONE',  ( 50.38147505302058704, 1.153996415704716449, -3.890257736381618869 ) ) ;
#9082=CARTESIAN_POINT ( 'NONE',  ( 48.48449022203101322, -1.386241252175273608, -3.851058308531627450 ) ) ;
#9083=CARTESIAN_POINT ( 'NONE',  ( 47.00000000000002132, 2.428612866367529932E-14, -4.100000000000022737 ) ) ;
#9087=ORIENTED_EDGE ( 'NONE', *, *, #261, .T. ) ;
#9089=CARTESIAN_POINT ( 'NONE',  ( 15.03925126672132961, -3.056483311920865642, 4.206888370749720885 ) ) ;
#9092=EDGE_LOOP ( 'NONE', ( #16111, #15743 ) ) ;
#9102=CARTESIAN_POINT ( 'NONE',  ( -37.18272003341174781, 5.407411300779116914, 0.000000000000000000 ) ) ;
#9103=ORIENTED_EDGE ( 'NONE', *, *, #6348, .F. ) ;
#9105=DIRECTION ( 'NONE',  ( -1.000000000000000000, -2.586136946169074517E-16, 0.000000000000000000 ) ) ;
#9113=CARTESIAN_POINT ( 'NONE',  ( 15.03925126672132961, -3.275050215668582787, -2.949461045527606462 ) ) ;
#9114=CARTESIAN_POINT ( 'NONE',  ( 57.01256279823148532, 0.7331429619035759737, -1.793127402884417965 ) ) ;
#9117=VECTOR ( 'NONE', #6569, 1000.000000000000227 ) ;
#9121=FACE_OUTER_BOUND ( 'NONE', #20480, .T. ) ;
#9122=EDGE_CURVE ( 'NONE', #17229, #18794, #2879, .T. ) ;
#9123=LINE ( 'NONE', #16396, #30726 ) ;
#9126=EDGE_CURVE ( 'NONE', #6920, #1141, #29261, .T. ) ;
#9130=CARTESIAN_POINT ( 'NONE',  ( 51.82407985978792198, 0.5160799604426919984, -4.312591426429957409 ) ) ;
#9137=ORIENTED_EDGE ( 'NONE', *, *, #27340, .T. ) ;
#9138=ORIENTED_EDGE ( 'NONE', *, *, #14738, .F. ) ;
#9139=DIRECTION ( 'NONE',  ( 1.000000000000000000, 0.000000000000000000, 0.000000000000000000 ) ) ;
#9142=DIRECTION ( 'NONE',  ( 0.000000000000000000, 0.000000000000000000, 1.000000000000000000 ) ) ;
#9149=DIRECTION ( 'NONE',  ( 0.000000000000000000, 1.000000000000000000, 0.000000000000000000 ) ) ;
#9150=AXIS2_PLACEMENT_3D ( 'NONE', #14778, #10335, #3062 ) ;
#9151=CARTESIAN_POINT ( 'NONE',  ( -36.00197790576392265, 1.123735532908270329, -5.289358697221547168 ) ) ;
#9157=CARTESIAN_POINT ( 'NONE',  ( 15.03925126672132961, 0.9159215771349776825, 4.311190327366002606 ) ) ;
#9160=CARTESIAN_POINT ( 'NONE',  ( -35.85663232820584057, 5.086913985776128300, 1.171642053949150331 ) ) ;
#9163=ORIENTED_EDGE ( 'NONE', *, *, #711, .F. ) ;
#9166=CARTESIAN_POINT ( 'NONE',  ( -36.27260443516980359, 0.1928884786867368362, 5.200000000471248107 ) ) ;
#9167=CARTESIAN_POINT ( 'NONE',  ( 48.34311953187607003, 1.211457450596386209, -3.917546004217189015 ) ) ;
#9169=DIRECTION ( 'NONE',  ( 1.000000000000000000, -0.000000000000000000, -0.000000000000000000 ) ) ;
#9170=VERTEX_POINT ( 'NONE', #14319 ) ;
#9178=DIRECTION ( 'NONE',  ( 1.000000000000000000, 0.000000000000000000, 0.000000000000000000 ) ) ;
#9184=CARTESIAN_POINT ( 'NONE',  ( -36.52679053911622731, 2.412550141807381809, 4.840569432287361806 ) ) ;
#9186=DIRECTION ( 'NONE',  ( 0.000000000000000000, 0.000000000000000000, 1.000000000000000000 ) ) ;
#9188=CARTESIAN_POINT ( 'NONE',  ( -54.48478889579405404, 1.513794642953540270, -4.039462313877657529 ) ) ;
#9190=VERTEX_POINT ( 'NONE', #12116 ) ;
#9191=CARTESIAN_POINT ( 'NONE',  ( 57.00108727371435435, -0.7119914823645937529, 1.810661949215600863 ) ) ;
#9193=CARTESIAN_POINT ( 'NONE',  ( -36.58361892166062290, 3.091683853622045230, -4.437651790015090469 ) ) ;
#9194=CARTESIAN_POINT ( 'NONE',  ( -39.16187796471576377, 5.407411300779124019, 0.000000000000000000 ) ) ;
#9197=ADVANCED_FACE ( 'NONE', ( #2613 ), #226, .F. ) ;
#9203=DIRECTION ( 'NONE',  ( -1.000000000000000000, -2.586136946169074517E-16, 0.000000000000000000 ) ) ;
#9208=CARTESIAN_POINT ( 'NONE',  ( 15.81621483022851926, -2.513248512186159633, -4.788125582312100725 ) ) ;
#9209=CARTESIAN_POINT ( 'NONE',  ( -36.22909104983326500, 4.895911367891157440, 2.323639554370136917 ) ) ;
#9210=CARTESIAN_POINT ( 'NONE',  ( 15.41080140630216988, -5.326563020867278730, 0.9981196555233698975 ) ) ;
#9212=ORIENTED_EDGE ( 'NONE', *, *, #24799, .T. ) ;
#9214=CARTESIAN_POINT ( 'NONE',  ( -39.16187796471576377, -5.407411300779158658, 6.622168941172401012E-16 ) ) ;
#9220=ORIENTED_EDGE ( 'NONE', *, *, #21151, .T. ) ;
#9230=DIRECTION ( 'NONE',  ( 0.000000000000000000, 0.000000000000000000, 1.000000000000000000 ) ) ;
#9233=EDGE_CURVE ( 'NONE', #16594, #2692, #28748, .T. ) ;
#9238=EDGE_CURVE ( 'NONE', #3627, #3082, #2056, .T. ) ;
#9240=CARTESIAN_POINT ( 'NONE',  ( -36.52757395963738674, -3.857619034241774880, -3.790808625284033617 ) ) ;
#9242=CARTESIAN_POINT ( 'NONE',  ( 57.03820272507597622, 0.7500000014582769436, -2.490438835250821992 ) ) ;
#9243=CARTESIAN_POINT ( 'NONE',  ( 50.36635169771310672, 1.250438735127648027, -3.874838289045730910 ) ) ;
#9246=CARTESIAN_POINT ( 'NONE',  ( 50.45647961155643912, -1.212999249975888816, 3.917061424767716904 ) ) ;
#9255=CARTESIAN_POINT ( 'NONE',  ( -35.85663232820584767, 4.383220986679468467, 0.4611378927914916992 ) ) ;
#9256=ORIENTED_EDGE ( 'NONE', *, *, #25991, .T. ) ;
#9266=ORIENTED_EDGE ( 'NONE', *, *, #20783, .T. ) ;
#9268=EDGE_CURVE ( 'NONE', #19424, #2253, #30177, .T. ) ;
#9270=CARTESIAN_POINT ( 'NONE',  ( 56.99032252660322939, -0.7964187825544630783, -2.475026498169530687 ) ) ;
#9273=CARTESIAN_POINT ( 'NONE',  ( 56.99976900444080030, 0.7668859551697654320, 1.738368808232523044 ) ) ;
#9276=CARTESIAN_POINT ( 'NONE',  ( -36.11122220296840624, -2.734418404389801438, 4.440882220947544923 ) ) ;
#9285=DIRECTION ( 'NONE',  ( 0.000000000000000000, 0.000000000000000000, 1.000000000000000000 ) ) ;
#9290=CARTESIAN_POINT ( 'NONE',  ( -36.04518387042616467, 3.779372851355696117, 3.883777284341113134 ) ) ;
#9295=ORIENTED_EDGE ( 'NONE', *, *, #18332, .T. ) ;
#9296=CARTESIAN_POINT ( 'NONE',  ( 50.37844020491943553, 1.181909706220234613, 3.885998080850100234 ) ) ;
#9299=CARTESIAN_POINT ( 'NONE',  ( 57.05000000000001847, 0.6999999999999999556, 0.000000000000000000 ) ) ;
#9302=EDGE_CURVE ( 'NONE', #25704, #8120, #24330, .T. ) ;
#9303=CARTESIAN_POINT ( 'NONE',  ( -54.46926330052497178, -1.503605180550108944, -3.302415457191589354 ) ) ;
#9304=CARTESIAN_POINT ( 'NONE',  ( 57.00000000000002132, 0.6820512820512792951, -1.773360101234991770 ) ) ;
#9306=VECTOR ( 'NONE', #14104, 1000.000000000000227 ) ;
#9308=CARTESIAN_POINT ( 'NONE',  ( 48.40000000000001990, -1.391941090707485618, 3.850000000000022737 ) ) ;
#9313=CARTESIAN_POINT ( 'NONE',  ( -54.49999999999997868, 0.000000000000000000, 4.650000000000000355 ) ) ;
#9317=CARTESIAN_POINT ( 'NONE',  ( 48.38952526309124380, 0.7808213810456217097, -4.027268569370236584 ) ) ;
#9333=DIRECTION ( 'NONE',  ( 1.000000000000000000, 0.000000000000000000, 0.000000000000000000 ) ) ;
#9340=CARTESIAN_POINT ( 'NONE',  ( -54.49999516060625382, 1.549196738101655368, -4.063926895246979143 ) ) ;
#9343=CARTESIAN_POINT ( 'NONE',  ( -36.63359589171323449, 2.513248512186358141, -4.788125582311988815 ) ) ;
#9344=CARTESIAN_POINT ( 'NONE',  ( 48.33000880451179881, 1.140870969100562293, -3.938727831757874664 ) ) ;
#9355=CARTESIAN_POINT ( 'NONE',  ( 34.55000000000001847, 3.245314017740485962E-16, 2.649999999999999911 ) ) ;
#9359=DIRECTION ( 'NONE',  ( 1.000000000000000000, 0.000000000000000000, 0.000000000000000000 ) ) ;
#9360=CARTESIAN_POINT ( 'NONE',  ( -36.11692583559979397, 5.377732435184220172, 0.5657657035923049360 ) ) ;
#9365=CARTESIAN_POINT ( 'NONE',  ( 50.33036399986577436, -1.366688880095578318, 3.854642372925541682 ) ) ;
#9366=ORIENTED_EDGE ( 'NONE', *, *, #15692, .F. ) ;
#9367=CARTESIAN_POINT ( 'NONE',  ( 57.02114944868134216, -0.7500000000000000000, -1.778342400449481442 ) ) ;
#9369=LINE ( 'NONE', #30, #19479 ) ;
#9372=ORIENTED_EDGE ( 'NONE', *, *, #14341, .T. ) ;
#9376=AXIS2_PLACEMENT_3D ( 'NONE', #24053, #14556, #23756 ) ;
#9381=CARTESIAN_POINT ( 'NONE',  ( 54.40000000000001990, 1.734723475976807094E-15, 0.000000000000000000 ) ) ;
#9383=AXIS2_PLACEMENT_3D ( 'NONE', #2246, #1613, #13957 ) ;
#9384=DIRECTION ( 'NONE',  ( 1.000000000000000000, 4.678365685400793326E-16, -1.520093157366863638E-16 ) ) ;
#9385=AXIS2_PLACEMENT_3D ( 'NONE', #25532, #6698, #21440 ) ;
#9387=CARTESIAN_POINT ( 'NONE',  ( -36.52679053911622731, 5.349174094756181219, -0.7986533162260476271 ) ) ;
#9392=CARTESIAN_POINT ( 'NONE',  ( -36.92398358572908990, -2.945786441214556017, -4.543674732827765794 ) ) ;
#9394=CARTESIAN_POINT ( 'NONE',  ( -35.85663232820584057, -3.275050215670988418, 2.949461045525626268 ) ) ;
#9397=VERTEX_POINT ( 'NONE', #29822 ) ;
#9398=LINE ( 'NONE', #17158, #30165 ) ;
#9399=CARTESIAN_POINT ( 'NONE',  ( 50.36059168657180862, -1.279117291415099000, 3.870058441400160198 ) ) ;
#9408=VERTEX_POINT ( 'NONE', #5755 ) ;
#9409=AXIS2_PLACEMENT_3D ( 'NONE', #16950, #12640, #29125 ) ;
#9410=CARTESIAN_POINT ( 'NONE',  ( 15.22780280894162885, 4.861582133259942928, 2.394243994563265421 ) ) ;
#9418=DIRECTION ( 'NONE',  ( 1.000000000000000000, 1.786976680021908743E-16, -2.459562394685749209E-16 ) ) ;
#9421=DIRECTION ( 'NONE',  ( 1.000000000000000000, 0.000000000000000000, 0.000000000000000000 ) ) ;
#9423=VECTOR ( 'NONE', #30582, 1000.000000000000000 ) ;
#9427=CARTESIAN_POINT ( 'NONE',  ( 57.05000000000001847, -0.7500000000000000000, 2.489477856900920383 ) ) ;
#9432=EDGE_CURVE ( 'NONE', #9911, #17666, #10738, .T. ) ;
#9434=CARTESIAN_POINT ( 'NONE',  ( 56.95000000000001705, 0.000000000000000000, 0.000000000000000000 ) ) ;
#9439=CARTESIAN_POINT ( 'NONE',  ( 46.92031786090804957, -4.254331549871407603, 1.021189760102710231 ) ) ;
#9444=AXIS2_PLACEMENT_3D ( 'NONE', #19439, #24190, #2497 ) ;
#9449=ORIENTED_EDGE ( 'NONE', *, *, #22977, .T. ) ;
#9452=DIRECTION ( 'NONE',  ( 1.000000000000000000, 0.000000000000000000, 0.000000000000000000 ) ) ;
#9454=CARTESIAN_POINT ( 'NONE',  ( -36.58361892166060869, 3.265074799938700867, 4.311675893545017679 ) ) ;
#9457=FACE_OUTER_BOUND ( 'NONE', #1741, .T. ) ;
#9465=DIRECTION ( 'NONE',  ( -1.000000000000000000, 0.000000000000000000, 0.000000000000000000 ) ) ;
#9469=AXIS2_PLACEMENT_3D ( 'NONE', #14405, #9359, #31208 ) ;
#9475=CARTESIAN_POINT ( 'NONE',  ( 51.81792662072884781, 0.6442955068957180176, 4.286808768127969849 ) ) ;
#9481=VERTEX_POINT ( 'NONE', #3999 ) ;
#9483=ORIENTED_EDGE ( 'NONE', *, *, #12450, .F. ) ;
#9487=CARTESIAN_POINT ( 'NONE',  ( -36.43290890416756866, -0.4851603899458980518, 5.391500295856537228 ) ) ;
#9488=DIRECTION ( 'NONE',  ( 0.000000000000000000, 0.000000000000000000, 1.000000000000000000 ) ) ;
#9491=CARTESIAN_POINT ( 'NONE',  ( -54.48779575765000516, 1.517266520141196118, 4.041867453639656382 ) ) ;
#9492=CIRCLE ( 'NONE', #29694, 0.05000000000000012768 ) ;
#9493=ORIENTED_EDGE ( 'NONE', *, *, #29244, .T. ) ;
#9495=CARTESIAN_POINT ( 'NONE',  ( 15.76623786017542272, 0.1071614981650652471, -5.407381887150171984 ) ) ;
#9497=DIRECTION ( 'NONE',  ( 0.000000000000000000, 0.000000000000000000, 1.000000000000000000 ) ) ;
#9499=ORIENTED_EDGE ( 'NONE', *, *, #8510, .T. ) ;
#9504=LINE ( 'NONE', #141, #2404 ) ;
#9517=VERTEX_POINT ( 'NONE', #23013 ) ;
#9518=AXIS2_PLACEMENT_3D ( 'NONE', #9011, #3778, #6637 ) ;
#9521=CARTESIAN_POINT ( 'NONE',  ( 16.10624235918717773, -3.309998894527983904, 4.278958290368447770 ) ) ;
#9524=DIRECTION ( 'NONE',  ( 1.000000000000000000, -0.000000000000000000, -0.000000000000000000 ) ) ;
#9526=CYLINDRICAL_SURFACE ( 'NONE', #27584, 0.9999999999999997780 ) ;
#9531=ADVANCED_FACE ( 'NONE', ( #8734 ), #25227, .T. ) ;
#9532=ORIENTED_EDGE ( 'NONE', *, *, #2584, .F. ) ;
#9535=CARTESIAN_POINT ( 'NONE',  ( 33.47623932017462778, -5.407411300779132013, 6.622168941172392137E-16 ) ) ;
#9537=CARTESIAN_POINT ( 'NONE',  ( -36.22818246778579976, 5.326563020867125964, 0.9981196555233160517 ) ) ;
#9538=CARTESIAN_POINT ( 'NONE',  ( 15.03925126672133139, -4.804073783693453947, 2.042134687550334338 ) ) ;
#9539=VERTEX_POINT ( 'NONE', #18123 ) ;
#9544=FACE_OUTER_BOUND ( 'NONE', #3111, .T. ) ;
#9545=DIRECTION ( 'NONE',  ( 1.000000000000000000, -0.000000000000000000, -0.000000000000000000 ) ) ;
#9558=DIRECTION ( 'NONE',  ( 1.000000000000000000, 0.000000000000000000, 4.738179285253022937E-16 ) ) ;
#9563=AXIS2_PLACEMENT_3D ( 'NONE', #11117, #8271, #13634 ) ;
#9568=CARTESIAN_POINT ( 'NONE',  ( -35.85663232820584057, -4.018128179617548312, -3.618665901676662244 ) ) ;
#9573=CARTESIAN_POINT ( 'NONE',  ( 48.44629147628577215, -1.309359793766436519, 3.864871860988134955 ) ) ;
#9574=CARTESIAN_POINT ( 'NONE',  ( 48.40000000000001279, -0.7619326981554292999, -3.939508824314740032 ) ) ;
#9575=CARTESIAN_POINT ( 'NONE',  ( 58.45000000000001705, 0.8000000000000000444, -2.421260002560649660 ) ) ;
#9581=EDGE_LOOP ( 'NONE', ( #22919, #3498, #7972, #9874 ) ) ;
#9582=CARTESIAN_POINT ( 'NONE',  ( 15.68751737981905592, 5.024465639092023928, 2.007392901578218147 ) ) ;
#9586=AXIS2_PLACEMENT_3D ( 'NONE', #1479, #20506, #13800 ) ;
#9587=EDGE_CURVE ( 'NONE', #7615, #11967, #27911, .T. ) ;
#9589=ORIENTED_EDGE ( 'NONE', *, *, #17593, .F. ) ;
#9598=AXIS2_PLACEMENT_3D ( 'NONE', #18164, #27803, #15449 ) ;
#9602=CARTESIAN_POINT ( 'NONE',  ( -36.68133364217528225, -2.563573972737447360, 4.761506352252311558 ) ) ;
#9604=( GEOMETRIC_REPRESENTATION_CONTEXT ( 3 ) GLOBAL_UNCERTAINTY_ASSIGNED_CONTEXT ( ( #26602 ) ) GLOBAL_UNIT_ASSIGNED_CONTEXT ( ( #7468, #4461, #28695 ) ) REPRESENTATION_CONTEXT ( 'NONE', 'WORKASPACE' ) );
#9608=EDGE_CURVE ( 'NONE', #13576, #17229, #20621, .T. ) ;
#9612=CIRCLE ( 'NONE', #13126, 1.000000000000000000 ) ;
#9617=CARTESIAN_POINT ( 'NONE',  ( 48.50000000000002132, -1.391941090707485396, 3.850000000000022737 ) ) ;
#9618=CARTESIAN_POINT ( 'NONE',  ( -35.85663232820596846, 2.525801270006243548, 4.794550352686347772 ) ) ;
#9621=DIRECTION ( 'NONE',  ( -0.000000000000000000, -0.9333474217026306308, 0.3589743589743588648 ) ) ;
#9622=ORIENTED_EDGE ( 'NONE', *, *, #12914, .F. ) ;
#9624=EDGE_CURVE ( 'NONE', #7081, #28342, #26325, .T. ) ;
#9626=CARTESIAN_POINT ( 'NONE',  ( 47.00000000000002132, 2.428612866367529932E-14, 0.000000000000000000 ) ) ;
#9639=FACE_OUTER_BOUND ( 'NONE', #19306, .T. ) ;
#9641=( BOUNDED_SURFACE ( )  B_SPLINE_SURFACE ( 3, 2, ( 
 ( #23783, #26739, #22150 ),
 ( #438, #10100, #28517 ),
 ( #9786, #6822, #2516 ),
 ( #16486, #16332, #2664 ),
 ( #12167, #4283, #26144 ),
 ( #21847, #21103, #19769 ),
 ( #14691, #19454, #13930 ),
 ( #29401, #29100, #23626 ),
 ( #7414, #5033, #16176 ),
 ( #12301, #21986, #30741 ),
 ( #25824, #279, #18721 ),
 ( #28364, #6669, #30898 ),
 ( #25282, #27345, #20244 ),
 ( #24955, #10714, #8188 ),
 ( #27020, #15309, #7712 ),
 ( #5328, #15466, #20553 ) ),
 .UNSPECIFIED., .F., .F., .F. ) 
 B_SPLINE_SURFACE_WITH_KNOTS ( ( 4, 2, 2, 2, 2, 2, 2, 4 ),
 ( 3, 3 ),
 ( 0.001780502285214263011, 0.002558945925323794120, 0.002753556835351177005, 0.002948167745378559457, 0.003337389565433324795, 0.003726611385488090566, 0.004115833205542856338, 0.004894276845652387013 ),
 ( 0.000000000000000000, 1.000000000000000000 ),
 .UNSPECIFIED. ) 
 GEOMETRIC_REPRESENTATION_ITEM ( )  RATIONAL_B_SPLINE_SURFACE ( (
 ( 1.000000000000000000, 0.9418517008537224955, 1.000000000000000000),
 ( 1.000000000000000000, 0.9417987965884832002, 1.000000000000000000),
 ( 1.000000000000000000, 0.9418198861734355942, 1.000000000000000000),
 ( 1.000000000000000000, 0.9434060303845482887, 1.000000000000000000),
 ( 1.000000000000000000, 0.9437939819948070186, 1.000000000000000000),
 ( 1.000000000000000000, 0.9445989566712852392, 1.000000000000000000),
 ( 1.000000000000000000, 0.9450169930049781009, 1.000000000000000000),
 ( 1.000000000000000000, 0.9461610507673672288, 1.000000000000000000),
 ( 1.000000000000000000, 0.9467217966427039499, 1.000000000000000000),
 ( 1.000000000000000000, 0.9467345476124477965, 1.000000000000000000),
 ( 1.000000000000000000, 0.9461964028052843867, 1.000000000000000000),
 ( 1.000000000000000000, 0.9446801822473894772, 1.000000000000000000),
 ( 1.000000000000000000, 0.9437582546537259809, 1.000000000000000000),
 ( 1.000000000000000000, 0.9418129560294213887, 1.000000000000000000),
 ( 1.000000000000000000, 0.9418016889778539902, 1.000000000000000000),
 ( 1.000000000000000000, 0.9418517008537212742, 1.000000000000000000) ) ) 
 REPRESENTATION_ITEM ( '' )  SURFACE ( )  );
#9642=VECTOR ( 'NONE', #20055, 1000.000000000000000 ) ;
#9648=CARTESIAN_POINT ( 'NONE',  ( -54.45996984137642727, 1.500763111530253990, 3.300586169551324556 ) ) ;
#9650=ORIENTED_EDGE ( 'NONE', *, *, #14084, .F. ) ;
#9651=CARTESIAN_POINT ( 'NONE',  ( -54.49131719536980967, 1.521332553059528081, 4.044684194243341580 ) ) ;
#9655=ORIENTED_EDGE ( 'NONE', *, *, #14738, .T. ) ;
#9658=CARTESIAN_POINT ( 'NONE',  ( 15.03925126672132961, 1.793057972834833924, -4.026191436120374334 ) ) ;
#9661=ORIENTED_EDGE ( 'NONE', *, *, #20992, .F. ) ;
#9664=CARTESIAN_POINT ( 'NONE',  ( 15.32752150720754081, -3.997744010329692177, -3.641645661657128219 ) ) ;
#9666=DIRECTION ( 'NONE',  ( 0.000000000000000000, -1.000000000000000000, 0.000000000000000000 ) ) ;
#9668=ORIENTED_EDGE ( 'NONE', *, *, #14371, .F. ) ;
#9669=CARTESIAN_POINT ( 'NONE',  ( 51.87968213909199733, -4.254331549871407603, -1.021189760102710675 ) ) ;
#9670=EDGE_CURVE ( 'NONE', #8110, #25975, #21593, .T. ) ;
#9671=DIRECTION ( 'NONE',  ( 0.000000000000000000, 1.000000000000000000, 0.000000000000000000 ) ) ;
#9679=DIRECTION ( 'NONE',  ( 0.000000000000000000, -1.000000000000000000, 1.224646799147352961E-16 ) ) ;
#9683=CARTESIAN_POINT ( 'NONE',  ( 15.41217651307626291, -2.840625797034020295, -4.363718033548148689 ) ) ;
#9684=CARTESIAN_POINT ( 'NONE',  ( -35.85663232820596136, 4.861582140531585772, 2.394243978978369825 ) ) ;
#9691=DIRECTION ( 'NONE',  ( 1.000000000000000000, 0.000000000000000000, 0.000000000000000000 ) ) ;
#9695=ORIENTED_EDGE ( 'NONE', *, *, #19855, .T. ) ;
#9704=CARTESIAN_POINT ( 'NONE',  ( 50.42215036618306812, 1.308847734660516071, 3.885629509820973659 ) ) ;
#9705=DIRECTION ( 'NONE',  ( 0.000000000000000000, 1.000000000000000000, 0.000000000000000000 ) ) ;
#9706=CARTESIAN_POINT ( 'NONE',  ( -54.48167032960165557, -1.510995100284906023, 3.307167554963765799 ) ) ;
#9710=CARTESIAN_POINT ( 'NONE',  ( -36.11122220296835650, -0.3980941177579191970, -5.199999998461563244 ) ) ;
#9713=CARTESIAN_POINT ( 'NONE',  ( 54.41118797001386298, 1.001877184765262739E-15, -4.375000000000000888 ) ) ;
#9714=CARTESIAN_POINT ( 'NONE',  ( 47.00000000000002132, -3.726179070414207928, 1.000000000000002220 ) ) ;
#9719=CARTESIAN_POINT ( 'NONE',  ( 48.46694841591348535, -1.365427245289796199, 3.854926352964885172 ) ) ;
#9721=ORIENTED_EDGE ( 'NONE', *, *, #2137, .T. ) ;
#9724=AXIS2_PLACEMENT_3D ( 'NONE', #19599, #256, #24471 ) ;
#9727=ORIENTED_EDGE ( 'NONE', *, *, #14651, .T. ) ;
#9729=CARTESIAN_POINT ( 'NONE',  ( 15.56274145962601274, 4.735538777079207229, 2.618062770414690821 ) ) ;
#9731=CARTESIAN_POINT ( 'NONE',  ( 48.45862863613069749, -1.344608935533137206, 3.858631320448701718 ) ) ;
#9734=CARTESIAN_POINT ( 'NONE',  ( 58.45000000000001705, -0.8000000000000000444, -2.421260002560650104 ) ) ;
#9737=EDGE_LOOP ( 'NONE', ( #6073, #2268, #1328, #24117, #2143, #16536 ) ) ;
#9740=CARTESIAN_POINT ( 'NONE',  ( -54.49131719536980967, -1.521332553059527859, 4.044684194243341580 ) ) ;
#9753=ORIENTED_EDGE ( 'NONE', *, *, #24882, .T. ) ;
#9756=CARTESIAN_POINT ( 'NONE',  ( 15.59055531549693541, 5.360541651686752118, 0.7128348320084746392 ) ) ;
#9769=ADVANCED_FACE ( 'NONE', ( #24861 ), #18849, .T. ) ;
#9779=CARTESIAN_POINT ( 'NONE',  ( 51.80000000000001847, 2.428612866367529932E-14, -4.100000000000022737 ) ) ;
#9780=CARTESIAN_POINT ( 'NONE',  ( -36.31414349454748702, -3.102491976071088065, -4.173461118157653971 ) ) ;
#9781=CARTESIAN_POINT ( 'NONE',  ( -54.49999999999997868, 1.549582583372307809, 3.331868970650947226 ) ) ;
#9784=CARTESIAN_POINT ( 'NONE',  ( -36.81959771849335539, -5.295593823078834639, 1.114646847977607935 ) ) ;
#9785=VERTEX_POINT ( 'NONE', #7628 ) ;
#9786=CARTESIAN_POINT ( 'NONE',  ( -36.38012252111052902, -4.735538777079435491, 2.618062770414280926 ) ) ;
#9790=ORIENTED_EDGE ( 'NONE', *, *, #25669, .T. ) ;
#9793=DIRECTION ( 'NONE',  ( 1.000000000000000000, 5.570239943078568709E-15, -9.650165233619991632E-15 ) ) ;
#9794=CARTESIAN_POINT ( 'NONE',  ( -54.44999999999997442, -1.499999999999999556, -4.029888335921975262 ) ) ;
#9797=AXIS2_PLACEMENT_3D ( 'NONE', #12454, #736, #7568 ) ;
#9800=DIRECTION ( 'NONE',  ( 0.000000000000000000, 0.000000000000000000, 1.000000000000000000 ) ) ;
#9804=CARTESIAN_POINT ( 'NONE',  ( -54.44999999999997442, 0.000000000000000000, 0.000000000000000000 ) ) ;
#9808=CARTESIAN_POINT ( 'NONE',  ( 36.55000000000001847, 0.000000000000000000, 0.000000000000000000 ) ) ;
#9810=CARTESIAN_POINT ( 'NONE',  ( -54.49999999999997868, 0.000000000000000000, 0.000000000000000000 ) ) ;
#9821=CARTESIAN_POINT ( 'NONE',  ( 15.56274145962692046, -2.292272662153287399, -4.901537128431941781 ) ) ;
#9823=CARTESIAN_POINT ( 'NONE',  ( 58.50000000000001421, 0.000000000000000000, 0.000000000000000000 ) ) ;
#9830=EDGE_CURVE ( 'NONE', #31046, #4702, #19647, .T. ) ;
#9831=CARTESIAN_POINT ( 'NONE',  ( 51.71945504228668966, -4.178364716350985830, 1.001910748144234864 ) ) ;
#9833=ORIENTED_EDGE ( 'NONE', *, *, #29184, .F. ) ;
#9834=CARTESIAN_POINT ( 'NONE',  ( -36.76447480099743359, -5.297368390263450522, -1.087079755157686289 ) ) ;
#9846=CARTESIAN_POINT ( 'NONE',  ( 56.95000000000001705, 0.000000000000000000, 0.000000000000000000 ) ) ;
#9847=CARTESIAN_POINT ( 'NONE',  ( 51.75323112273434845, -4.276948283761179859, -0.9210528638641413135 ) ) ;
#9849=CARTESIAN_POINT ( 'NONE',  ( -35.98952425903316055, -0.4576450703117335150, -5.200000005133903258 ) ) ;
#9853=CARTESIAN_POINT ( 'NONE',  ( 15.32766723174652945, -3.997758138077576628, 3.641634024966071692 ) ) ;
#9854=CARTESIAN_POINT ( 'NONE',  ( 15.29449157529478320, 4.822464347458993217, -1.985534350301433326 ) ) ;
#9860=DIRECTION ( 'NONE',  ( 1.000000000000000000, 2.586136946169074517E-16, -0.000000000000000000 ) ) ;
#9866=ADVANCED_FACE ( 'NONE', ( #4887 ), #9986, .T. ) ;
#9867=ORIENTED_EDGE ( 'NONE', *, *, #30812, .F. ) ;
#9868=AXIS2_PLACEMENT_3D ( 'NONE', #17931, #27571, #21106 ) ;
#9873=CARTESIAN_POINT ( 'NONE',  ( 15.59055531549693363, 4.755763096844290772, -2.574151833883746576 ) ) ;
#9874=ORIENTED_EDGE ( 'NONE', *, *, #12813, .T. ) ;
#9875=CARTESIAN_POINT ( 'NONE',  ( 48.40000000000001990, -0.7618928438396727065, 3.939512004971702730 ) ) ;
#9882=ORIENTED_EDGE ( 'NONE', *, *, #12606, .F. ) ;
#9883=CIRCLE ( 'NONE', #21034, 1.000000000000000000 ) ;
#9887=CARTESIAN_POINT ( 'NONE',  ( 48.50000000000002132, 1.426739617975221641, -3.843750000000023093 ) ) ;
#9891=CARTESIAN_POINT ( 'NONE',  ( -36.89250464418362441, -3.430438802933830189, 4.182416543699121192 ) ) ;
#9897=AXIS2_PLACEMENT_3D ( 'NONE', #13561, #3745, #27832 ) ;
#9901=VERTEX_POINT ( 'NONE', #6794 ) ;
#9905=CARTESIAN_POINT ( 'NONE',  ( 15.32752150720753725, 5.374748457514294309, 0.5963382560600952731 ) ) ;
#9911=VERTEX_POINT ( 'NONE', #2360 ) ;
#9920=ADVANCED_FACE ( 'NONE', ( #7263 ), #27681, .T. ) ;
#9927=CIRCLE ( 'NONE', #25073, 0.09999999999999986677 ) ;
#9937=CARTESIAN_POINT ( 'NONE',  ( -36.25997906085250122, -3.232943006030368327, -4.078682900256746180 ) ) ;
#9938=CARTESIAN_POINT ( 'NONE',  ( 54.40000000000001990, 3.918869757271530460E-16, 3.200000000000000178 ) ) ;
#9941=CARTESIAN_POINT ( 'NONE',  ( -54.48118151432741030, 1.510613940323803916, 4.037256667234631280 ) ) ;
#9943=CIRCLE ( 'NONE', #12034, 4.375000000000000000 ) ;
#9945=CARTESIAN_POINT ( 'NONE',  ( 16.10624235918717417, 0.1627367787820844514, -5.407318510437580272 ) ) ;
#9947=CARTESIAN_POINT ( 'NONE',  ( -35.85663232820584057, 2.686240680702182804, -4.475885388010699018 ) ) ;
#9948=CARTESIAN_POINT ( 'NONE',  ( 50.50000000000002132, 2.428612866367529932E-14, 0.000000000000000000 ) ) ;
#9956=ORIENTED_EDGE ( 'NONE', *, *, #13610, .T. ) ;
#9958=CARTESIAN_POINT ( 'NONE',  ( 15.03925126672132961, 3.426725943139508512, 3.937891353488783164 ) ) ;
#9959=CARTESIAN_POINT ( 'NONE',  ( 57.02478278053006022, -0.7769964508979760875, 1.733862565638740305 ) ) ;
#9965=AXIS2_PLACEMENT_3D ( 'NONE', #27913, #13491, #13322 ) ;
#9968=CYLINDRICAL_SURFACE ( 'NONE', #6294, 1.899999999999999911 ) ;
#9970=CARTESIAN_POINT ( 'NONE',  ( 15.44259799936805955, -3.232943006030354560, 4.078682900256773713 ) ) ;
#9971=AXIS2_PLACEMENT_3D ( 'NONE', #28166, #1413, #1563 ) ;
#9974=DIRECTION ( 'NONE',  ( -2.964772755551650383E-16, 0.9875000000000001554, 0.1576190026614809614 ) ) ;
#9980=VERTEX_POINT ( 'NONE', #17102 ) ;
#9984=AXIS2_PLACEMENT_3D ( 'NONE', #28191, #4440, #6806 ) ;
#9985=ORIENTED_EDGE ( 'NONE', *, *, #12479, .T. ) ;
#9986=TOROIDAL_SURFACE ( 'NONE', #13510, -24.59258869922086888, 30.00000000000000000 ) ;
#9989=DIRECTION ( 'NONE',  ( 0.000000000000000000, -1.000000000000000000, 2.168404344971008868E-16 ) ) ;
#9990=CARTESIAN_POINT ( 'NONE',  ( 58.45000000000001705, -0.7500000000000000000, -2.489477856900920383 ) ) ;
#9991=EDGE_CURVE ( 'NONE', #10898, #19112, #20032, .T. ) ;
#9992=ORIENTED_EDGE ( 'NONE', *, *, #3799, .F. ) ;
#10000=DIRECTION ( 'NONE',  ( 1.000000000000000000, 0.000000000000000000, -4.738179285253022937E-16 ) ) ;
#10018=CARTESIAN_POINT ( 'NONE',  ( -36.38139716712170468, 1.027070083876471474, -5.312835761376594412 ) ) ;
#10019=AXIS2_PLACEMENT_3D ( 'NONE', #28565, #12107, #14309 ) ;
#10021=CARTESIAN_POINT ( 'NONE',  ( 54.50000000000002132, -0.003244837758069130020, -4.274998768541101057 ) ) ;
#10032=EDGE_CURVE ( 'NONE', #18916, #10683, #18603, .T. ) ;
#10038=VERTEX_POINT ( 'NONE', #26885 ) ;
#10045=ORIENTED_EDGE ( 'NONE', *, *, #18205, .T. ) ;
#10048=CARTESIAN_POINT ( 'NONE',  ( -54.48478889579405404, -1.513794642953540048, 4.039462313877656641 ) ) ;
#10050=DIRECTION ( 'NONE',  ( -1.000000000000000000, -2.586136946169074517E-16, 0.000000000000000000 ) ) ;
#10052=CARTESIAN_POINT ( 'NONE',  ( 57.00303004862897183, 0.7171412854886025645, 2.441992855427530085 ) ) ;
#10056=CARTESIAN_POINT ( 'NONE',  ( 15.03925126672133139, -3.817150320980667200, 2.203324261490537062 ) ) ;
#10058=ORIENTED_EDGE ( 'NONE', *, *, #26681, .T. ) ;
#10062=ORIENTED_EDGE ( 'NONE', *, *, #3473, .F. ) ;
#10063=CYLINDRICAL_SURFACE ( 'NONE', #11863, 0.1000000000000000472 ) ;
#10067=ORIENTED_EDGE ( 'NONE', *, *, #29901, .T. ) ;
#10068=ORIENTED_EDGE ( 'NONE', *, *, #13354, .F. ) ;
#10072=ORIENTED_EDGE ( 'NONE', *, *, #24374, .T. ) ;
#10078=CARTESIAN_POINT ( 'NONE',  ( 15.57907767661739840, -4.962973169597029610, -2.162832296644437768 ) ) ;
#10081=ADVANCED_FACE ( 'NONE', ( #27031 ), #12495, .F. ) ;
#10082=MECHANICAL_DESIGN_GEOMETRIC_PRESENTATION_REPRESENTATION('',(#29806),#9604);
#10085=ADVANCED_FACE ( 'NONE', ( #16687 ), #2251, .T. ) ;
#10088=CARTESIAN_POINT ( 'NONE',  ( 16.10660252424457894, -5.231589534716065693, -1.397536681175223228 ) ) ;
#10089=CARTESIAN_POINT ( 'NONE',  ( 50.50000000000002132, 0.6304760106459519342, -3.950000000000022826 ) ) ;
#10090=ORIENTED_EDGE ( 'NONE', *, *, #19886, .F. ) ;
#10091=DIRECTION ( 'NONE',  ( 0.000000000000000000, 1.776356839400250465E-15, 1.000000000000000000 ) ) ;
#10092=CARTESIAN_POINT ( 'NONE',  ( -36.30424252565893539, -2.966783028120398846, -4.272059443775234833 ) ) ;
#10093=FACE_OUTER_BOUND ( 'NONE', #11894, .T. ) ;
#10096=CARTESIAN_POINT ( 'NONE',  ( 50.50000000000002132, 0.7901969350670130510, -4.025772098418840983 ) ) ;
#10100=CARTESIAN_POINT ( 'NONE',  ( -36.04518387042616467, -4.861582133259191529, 2.394243994563265865 ) ) ;
#10105=AXIS2_PLACEMENT_3D ( 'NONE', #27997, #8532, #18218 ) ;
#10106=DIRECTION ( 'NONE',  ( 0.000000000000000000, 0.1576190026614809614, 0.9875000000000001554 ) ) ;
#10109=DIRECTION ( 'NONE',  ( 0.000000000000000000, 0.000000000000000000, -1.000000000000000000 ) ) ;
#10110=DIRECTION ( 'NONE',  ( 0.000000000000000000, -0.9663289263986323263, -0.2573099415204678220 ) ) ;
#10113=CARTESIAN_POINT ( 'NONE',  ( 15.18463186935388087, -2.199885893005466553, -4.939696249117980997 ) ) ;
#10130=ADVANCED_FACE ( 'NONE', ( #30921 ), #21601, .T. ) ;
#10135=CARTESIAN_POINT ( 'NONE',  ( 57.00174889577907322, 0.7131084301676396953, -2.444403622924161912 ) ) ;
#10142=VERTEX_POINT ( 'NONE', #19060 ) ;
#10145=CARTESIAN_POINT ( 'NONE',  ( 58.45000000000001705, -0.8000000000000000444, -2.471260002560650371 ) ) ;
#10146=CARTESIAN_POINT ( 'NONE',  ( -36.58361892166016816, -5.175840503946164795, -1.569056257078813355 ) ) ;
#10147=ORIENTED_EDGE ( 'NONE', *, *, #6616, .T. ) ;
#10150=B_SPLINE_CURVE_WITH_KNOTS ( 'NONE', 3,
 ( #27453, #7103, #9648, #22404, #14533, #28792, #5619, #7407, #10529, #24770, #19301, #20202, #13048, #28937, #29833, #8143, #10354, #9781, #20030 ),
 .UNSPECIFIED., .F., .F.,
 ( 4, 3, 3, 3, 3, 3, 4 ),
 ( 0.000000000000000000, 1.485152479261661559E-05, 2.963899638137941126E-05, 4.531421101975836217E-05, 6.339282692920784022E-05, 8.412900350910327988E-05, 8.561427748423850544E-05 ),
 .UNSPECIFIED. ) ;
#10153=CARTESIAN_POINT ( 'NONE',  ( 48.46244267249164039, -1.426738769040753363, -3.843750315111145621 ) ) ;
#10154=DIRECTION ( 'NONE',  ( -1.000000000000000000, 0.000000000000000000, 0.000000000000000000 ) ) ;
#10155=CARTESIAN_POINT ( 'NONE',  ( 51.80639759064268191, -4.235057606083633353, -1.098058400101913357 ) ) ;
#10158=DIRECTION ( 'NONE',  ( -1.000000000000000000, -4.939082069373447378E-17, -1.520093157366847861E-16 ) ) ;
#10160=CARTESIAN_POINT ( 'NONE',  ( 16.10667815269232861, -3.294441450831202101, 4.290383166762130607 ) ) ;
#10165=CARTESIAN_POINT ( 'NONE',  ( 50.45688046812396976, -1.211457450596347352, -3.917546004217186351 ) ) ;
#10167=CARTESIAN_POINT ( 'NONE',  ( 15.03925126672132961, 2.199885893006009674, -4.939696249117653259 ) ) ;
#10169=CARTESIAN_POINT ( 'NONE',  ( 56.95000000000001705, 0.7137254901960795594, 2.500119182087999103 ) ) ;
#10170=ORIENTED_EDGE ( 'NONE', *, *, #17913, .T. ) ;
#10175=ORIENTED_EDGE ( 'NONE', *, *, #21836, .T. ) ;
#10176=EDGE_CURVE ( 'NONE', #1297, #8161, #18034, .T. ) ;
#10180=CARTESIAN_POINT ( 'NONE',  ( -35.85663232820583346, -3.817150320980530864, 2.203324261490918090 ) ) ;
#10182=ORIENTED_EDGE ( 'NONE', *, *, #23686, .F. ) ;
#10183=CARTESIAN_POINT ( 'NONE',  ( 54.49508724208691746, -0.002176679993770252661, 4.307918145378301311 ) ) ;
#10189=CARTESIAN_POINT ( 'NONE',  ( 51.73251178704410336, -4.176834854957373722, -1.005432649909180576 ) ) ;
#10191=CARTESIAN_POINT ( 'NONE',  ( -54.47710365256552478, -1.507983431629474014, 4.035431478432993657 ) ) ;
#10192=CYLINDRICAL_SURFACE ( 'NONE', #2619, 0.05000000000000143219 ) ;
#10193=CARTESIAN_POINT ( 'NONE',  ( 50.30000000000001847, 1.391941090707534023, 3.750000000000022649 ) ) ;
#10194=EDGE_CURVE ( 'NONE', #9911, #11417, #13449, .T. ) ;
#10198=CARTESIAN_POINT ( 'NONE',  ( 51.80000000000001847, 1.521694824349982378, -3.995005614707754393 ) ) ;
#10199=CARTESIAN_POINT ( 'NONE',  ( 36.50000000000002132, 0.000000000000000000, 0.000000000000000000 ) ) ;
#10210=CARTESIAN_POINT ( 'NONE',  ( 15.03925126672133139, -4.383220986679489783, 0.4611378927914256409 ) ) ;
#10216=VERTEX_POINT ( 'NONE', #12085 ) ;
#10220=ADVANCED_FACE ( 'NONE', ( #49 ), #4157, .T. ) ;
#10222=DIRECTION ( 'NONE',  ( -1.000000000000000000, 0.000000000000000000, 0.000000000000000000 ) ) ;
#10224=ORIENTED_EDGE ( 'NONE', *, *, #13059, .F. ) ;
#10225=CARTESIAN_POINT ( 'NONE',  ( 15.03925126672132961, -5.340403872473328484, -0.9205822173396246422 ) ) ;
#10229=EDGE_CURVE ( 'NONE', #16545, #24817, #22055, .T. ) ;
#10236=DIRECTION ( 'NONE',  ( -1.000000000000000000, -1.293068473084537258E-16, -0.000000000000000000 ) ) ;
#10238=ORIENTED_EDGE ( 'NONE', *, *, #1348, .F. ) ;
#10240=LINE ( 'NONE', #26732, #23162 ) ;
#10250=EDGE_CURVE ( 'NONE', #31043, #19303, #27587, .T. ) ;
#10258=DIRECTION ( 'NONE',  ( -1.000000000000000000, -0.000000000000000000, -0.000000000000000000 ) ) ;
#10260=CARTESIAN_POINT ( 'NONE',  ( 56.95000000000001705, -0.6937162836135747357, 1.768873629894432975 ) ) ;
#10266=DIRECTION ( 'NONE',  ( 1.000000000000000000, -0.000000000000000000, -0.000000000000000000 ) ) ;
#10269=CARTESIAN_POINT ( 'NONE',  ( 15.76623786017564832, 3.091683853622046119, 4.437651790014722764 ) ) ;
#10274=CARTESIAN_POINT ( 'NONE',  ( -36.11122220296836360, 4.822476035523766136, -1.985498375066671262 ) ) ;
#10277=ORIENTED_EDGE ( 'NONE', *, *, #9991, .T. ) ;
#10281=AXIS2_PLACEMENT_3D ( 'NONE', #6164, #3626, #13258 ) ;
#10282=CARTESIAN_POINT ( 'NONE',  ( 15.22842924604238313, -3.779372845004303372, -3.883777290284644579 ) ) ;
#10283=DIRECTION ( 'NONE',  ( 0.000000000000000000, -1.000000000000000000, 0.000000000000000000 ) ) ;
#10285=ORIENTED_EDGE ( 'NONE', *, *, #28454, .F. ) ;
#10292=CARTESIAN_POINT ( 'NONE',  ( 56.99139336475067807, -0.7078862301243328270, -1.763423818528686349 ) ) ;
#10294=CARTESIAN_POINT ( 'NONE',  ( -36.30424252565903487, -4.911231426340521011, -1.712337380313407209 ) ) ;
#10296=CARTESIAN_POINT ( 'NONE',  ( -54.44999999999997442, 0.000000000000000000, 2.168404344971008868E-14 ) ) ;
#10297=VERTEX_POINT ( 'NONE', #19687 ) ;
#10302=AXIS2_PLACEMENT_3D ( 'NONE', #21338, #6909, #2145 ) ;
#10303=CARTESIAN_POINT ( 'NONE',  ( 16.07512358269906372, 0.3169205264062135985, 5.400007398663869473 ) ) ;
#10307=CARTESIAN_POINT ( 'NONE',  ( -36.50489844130334660, -0.3564988296781614885, -5.398869307934827333 ) ) ;
#10317=CARTESIAN_POINT ( 'NONE',  ( 15.94709373951304698, 3.646691605040303763, -3.993181011920754475 ) ) ;
#10327=CARTESIAN_POINT ( 'NONE',  ( 15.61552784268241822, 5.277544294472392927, 1.204650266290664407 ) ) ;
#10328=ORIENTED_EDGE ( 'NONE', *, *, #20916, .F. ) ;
#10332=VERTEX_POINT ( 'NONE', #10021 ) ;
#10333=DIRECTION ( 'NONE',  ( 1.000000000000000000, 0.000000000000000000, 0.000000000000000000 ) ) ;
#10335=DIRECTION ( 'NONE',  ( 1.000000000000000000, 3.125586771759065906E-16, 0.000000000000000000 ) ) ;
#10338=EDGE_CURVE ( 'NONE', #17296, #17741, #6785, .T. ) ;
#10341=CARTESIAN_POINT ( 'NONE',  ( 58.45000000000001705, -0.8000000000000001554, -1.778341924377873973 ) ) ;
#10342=DIRECTION ( 'NONE',  ( 0.000000000000000000, 0.000000000000000000, -1.000000000000000000 ) ) ;
#10352=CIRCLE ( 'NONE', #750, 0.05000000000000015543 ) ;
#10354=CARTESIAN_POINT ( 'NONE',  ( -54.49999477219272848, 1.549165129012789466, 3.331602747802265174 ) ) ;
#10355=EDGE_LOOP ( 'NONE', ( #22574, #1955, #28445, #2216 ) ) ;
#10361=CARTESIAN_POINT ( 'NONE',  ( 15.97944027357900687, 4.944296796129566296, 2.193698057025775583 ) ) ;
#10363=ORIENTED_EDGE ( 'NONE', *, *, #18713, .T. ) ;
#10365=VECTOR ( 'NONE', #20384, 1000.000000000000000 ) ;
#10369=ORIENTED_EDGE ( 'NONE', *, *, #20074, .T. ) ;
#10375=CARTESIAN_POINT ( 'NONE',  ( 15.67083574136775681, -5.256402525809859227, -1.287848407636900117 ) ) ;
#10386=VECTOR ( 'NONE', #29327, 1000.000000000000000 ) ;
#10392=CARTESIAN_POINT ( 'NONE',  ( -36.48174642953001978, -3.496282614933922783, -4.130238739723587571 ) ) ;
#10394=AXIS2_PLACEMENT_3D ( 'NONE', #13359, #15763, #13068 ) ;
#10395=EDGE_LOOP ( 'NONE', ( #19168, #11816, #24769, #4683 ) ) ;
#10396=ADVANCED_FACE ( 'NONE', ( #8100 ), #23592, .T. ) ;
#10398=ORIENTED_EDGE ( 'NONE', *, *, #3009, .T. ) ;
#10403=CARTESIAN_POINT ( 'NONE',  ( 58.50000000000001421, 0.000000000000000000, 0.000000000000000000 ) ) ;
#10408=CARTESIAN_POINT ( 'NONE',  ( 57.00965563974653350, -0.7295352771400042124, -1.796193723857490321 ) ) ;
#10411=CARTESIAN_POINT ( 'NONE',  ( -54.46895629856896903, -1.503487923075246480, -4.032311158269683560 ) ) ;
#10412=DIRECTION ( 'NONE',  ( -1.000000000000000000, -0.000000000000000000, -0.000000000000000000 ) ) ;
#10420=CARTESIAN_POINT ( 'NONE',  ( 51.90000000000001279, 1.734723475976807094E-15, 0.000000000000000000 ) ) ;
#10422=CARTESIAN_POINT ( 'NONE',  ( 16.00221665700883378, 0.5763363385013873241, 5.380853831843024793 ) ) ;
#10425=AXIS2_PLACEMENT_3D ( 'NONE', #29354, #2918, #12115 ) ;
#10430=EDGE_CURVE ( 'NONE', #3555, #12911, #22578, .T. ) ;
#10432=DIRECTION ( 'NONE',  ( 0.000000000000000000, 0.000000000000000000, -1.000000000000000000 ) ) ;
#10435=CARTESIAN_POINT ( 'NONE',  ( -36.04518387042480043, 4.861582133260092142, -2.394243994563964417 ) ) ;
#10439=CYLINDRICAL_SURFACE ( 'NONE', #24940, 0.1000000000000000472 ) ;
#10441=ORIENTED_EDGE ( 'NONE', *, *, #28770, .T. ) ;
#10450=CIRCLE ( 'NONE', #3868, 0.09999999999999986677 ) ;
#10456=CARTESIAN_POINT ( 'NONE',  ( 51.79412664516154763, -4.148449925053760090, 1.066233527417929539 ) ) ;
#10457=CARTESIAN_POINT ( 'NONE',  ( 50.31565037626138803, 1.386108502191577108, 3.851082811767820413 ) ) ;
#10458=CARTESIAN_POINT ( 'NONE',  ( -35.85663232820584057, -4.804073783693461941, 2.042134687550347216 ) ) ;
#10461=TOROIDAL_SURFACE ( 'NONE', #28146, 2.649999999999999911, 0.05000000000000000278 ) ;
#10463=VECTOR ( 'NONE', #14182, 1000.000000000000000 ) ;
#10466=FACE_OUTER_BOUND ( 'NONE', #28280, .T. ) ;
#10471=AXIS2_PLACEMENT_3D ( 'NONE', #9434, #1987, #22050 ) ;
#10476=DIRECTION ( 'NONE',  ( -1.000000000000000000, -0.000000000000000000, -0.000000000000000000 ) ) ;
#10479=CARTESIAN_POINT ( 'NONE',  ( 51.90000000000001990, -4.131056160354152240, -1.100000000000000089 ) ) ;
#10481=DIRECTION ( 'NONE',  ( 1.000000000000000000, 8.626663965456221796E-17, 1.494526870159859873E-16 ) ) ;
#10483=ORIENTED_EDGE ( 'NONE', *, *, #20072, .F. ) ;
#10485=DIRECTION ( 'NONE',  ( 1.000000000000000000, -0.000000000000000000, -0.000000000000000000 ) ) ;
#10487=CARTESIAN_POINT ( 'NONE',  ( 15.29954477411490465, 4.018128194441618284, -3.618665885216152400 ) ) ;
#10492=CARTESIAN_POINT ( 'NONE',  ( 51.80000000000001847, 1.521694824349982378, -3.995005614707754393 ) ) ;
#10494=EDGE_CURVE ( 'NONE', #16074, #26012, #15492, .T. ) ;
#10497=CARTESIAN_POINT ( 'NONE',  ( -45.15971931043468146, 0.000000000000000000, 0.000000000000000000 ) ) ;
#10500=CARTESIAN_POINT ( 'NONE',  ( 51.70000000000001705, -4.179189514726507682, 0.8999999999999998002 ) ) ;
#10508=AXIS2_PLACEMENT_3D ( 'NONE', #2140, #11962, #1990 ) ;
#10515=CARTESIAN_POINT ( 'NONE',  ( 17.21035195517769267, 5.407411300779131125, 0.000000000000000000 ) ) ;
#10517=CARTESIAN_POINT ( 'NONE',  ( -35.85663232820584057, 0.9159215771353744762, 4.311190327365977737 ) ) ;
#10529=CARTESIAN_POINT ( 'NONE',  ( -54.48531357662248809, 1.514292094527452504, 3.309285685900293927 ) ) ;
#10540=AXIS2_PLACEMENT_3D ( 'NONE', #8430, #27434, #27751 ) ;
#10543=EDGE_LOOP ( 'NONE', ( #2346, #15145, #16290, #11763 ) ) ;
#10551=EDGE_CURVE ( 'NONE', #18572, #2009, #4442, .T. ) ;
#10552=CARTESIAN_POINT ( 'NONE',  ( 48.43975240335598897, 1.282505688586122572, 3.869483523004607406 ) ) ;
#10553=CARTESIAN_POINT ( 'NONE',  ( -35.85663232820584057, -0.9159215771349861202, -4.311190327366008823 ) ) ;
#10558=CIRCLE ( 'NONE', #30251, 4.299999999999998046 ) ;
#10567=DIRECTION ( 'NONE',  ( -1.000000000000000000, 0.000000000000000000, 0.000000000000000000 ) ) ;
#10572=DIRECTION ( 'NONE',  ( 1.000000000000000000, 4.939082069373669245E-17, -1.520093157366878429E-16 ) ) ;
#10575=PLANE ( 'NONE',  #20617 ) ;
#10576=ORIENTED_EDGE ( 'NONE', *, *, #28431, .F. ) ;
#10578=CYLINDRICAL_SURFACE ( 'NONE', #6974, 1.000000000000000000 ) ;
#10579=ORIENTED_EDGE ( 'NONE', *, *, #13276, .F. ) ;
#10582=CARTESIAN_POINT ( 'NONE',  ( 56.95641943120798345, -0.7163990203283279179, 1.759764883066090801 ) ) ;
#10584=AXIS2_PLACEMENT_3D ( 'NONE', #19953, #17583, #27227 ) ;
#10587=ORIENTED_EDGE ( 'NONE', *, *, #2806, .F. ) ;
#10589=CARTESIAN_POINT ( 'NONE',  ( 15.56401610563845672, -2.291889356119292120, 4.901871067649883784 ) ) ;
#10607=ORIENTED_EDGE ( 'NONE', *, *, #10229, .T. ) ;
#10621=AXIS2_PLACEMENT_3D ( 'NONE', #2479, #29510, #14657 ) ;
#10625=CARTESIAN_POINT ( 'NONE',  ( 15.61552784268242000, 0.4851603899461020553, 5.391500295856302749 ) ) ;
#10627=VECTOR ( 'NONE', #7692, 1000.000000000000000 ) ;
#10632=CARTESIAN_POINT ( 'NONE',  ( 51.80000000000001847, 2.428612866367529932E-14, 0.000000000000000000 ) ) ;
#10642=ORIENTED_EDGE ( 'NONE', *, *, #21675, .F. ) ;
#10645=ORIENTED_EDGE ( 'NONE', *, *, #4981, .T. ) ;
#10646=FACE_OUTER_BOUND ( 'NONE', #16336, .T. ) ;
#10654=CARTESIAN_POINT ( 'NONE',  ( 58.45000000000001705, 0.8000000000000002665, -2.421260002560650104 ) ) ;
#10659=PLANE ( 'NONE',  #14196 ) ;
#10663=DIRECTION ( 'NONE',  ( 0.000000000000000000, 0.000000000000000000, 1.000000000000000000 ) ) ;
#10664=CARTESIAN_POINT ( 'NONE',  ( 58.45000000000001705, 0.8000000000000000444, -2.421260002560649660 ) ) ;
#10665=CARTESIAN_POINT ( 'NONE',  ( 34.50000000000001421, 0.000000000000000000, 0.000000000000000000 ) ) ;
#10667=EDGE_CURVE ( 'NONE', #29070, #2569, #27755, .T. ) ;
#10669=CIRCLE ( 'NONE', #25828, 4.375000000000000000 ) ;
#10670=DIRECTION ( 'NONE',  ( 1.000000000000000000, 0.000000000000000000, 0.000000000000000000 ) ) ;
#10673=CARTESIAN_POINT ( 'NONE',  ( -54.47754877553799702, 1.508273929415538062, -3.305418158118663907 ) ) ;
#10683=VERTEX_POINT ( 'NONE', #29127 ) ;
#10685=CIRCLE ( 'NONE', #12206, 0.4576450603546982632 ) ;
#10686=EDGE_LOOP ( 'NONE', ( #2519, #9138, #234, #8250, #10224 ) ) ;
#10688=DIRECTION ( 'NONE',  ( 0.000000000000000000, 0.000000000000000000, 1.000000000000000000 ) ) ;
#10689=VERTEX_POINT ( 'NONE', #24836 ) ;
#10692=SPHERICAL_SURFACE ( 'NONE', #26320, 0.05000000000000000278 ) ;
#10699=AXIS2_PLACEMENT_3D ( 'NONE', #26359, #26828, #2457 ) ;
#10700=DIRECTION ( 'NONE',  ( 1.000000000000000000, 0.000000000000000000, -0.000000000000000000 ) ) ;
#10706=DIRECTION ( 'NONE',  ( 1.000000000000000000, 0.000000000000000000, 0.000000000000000000 ) ) ;
#10714=CARTESIAN_POINT ( 'NONE',  ( -36.22909104983321527, -5.326676561279865219, 0.9978806102897157526 ) ) ;
#10719=EDGE_CURVE ( 'NONE', #30422, #9190, #20737, .T. ) ;
#10720=CARTESIAN_POINT ( 'NONE',  ( 57.00630022123013418, -0.7249518695496515175, -1.800067615291236711 ) ) ;
#10723=DIRECTION ( 'NONE',  ( 1.000000000000000000, 2.586136946169074517E-16, -0.000000000000000000 ) ) ;
#10727=CARTESIAN_POINT ( 'NONE',  ( -36.25997906085253675, 4.878092280899812394, -1.814329181850203865 ) ) ;
#10734=CARTESIAN_POINT ( 'NONE',  ( 15.74504787372188908, 3.003531019938586955, 4.498666779076369693 ) ) ;
#10738=B_SPLINE_CURVE_WITH_KNOTS ( 'NONE', 3,
 ( #2756, #22095, #14931, #10052, #5278, #7808, #19721, #29356, #26970, #2919, #19864, #10807, #28058, #30584, #6375, #13789 ),
 .UNSPECIFIED., .F., .F.,
 ( 4, 3, 3, 3, 3, 4 ),
 ( 0.000000000000000000, 2.009849036138677304E-05, 3.995053695856421648E-05, 5.889062715234580982E-05, 7.635198602698413037E-05, 8.503766575809868053E-05 ),
 .UNSPECIFIED. ) ;
#10739=EDGE_CURVE ( 'NONE', #8076, #3273, #3764, .T. ) ;
#10744=CYLINDRICAL_SURFACE ( 'NONE', #22432, 1.000000000000000000 ) ;
#10751=ORIENTED_EDGE ( 'NONE', *, *, #5718, .F. ) ;
#10764=ADVANCED_FACE ( 'NONE', ( #12792 ), #237, .T. ) ;
#10767=CARTESIAN_POINT ( 'NONE',  ( 48.40130545986176003, -0.9107929593199913798, -3.923749358243191043 ) ) ;
#10773=AXIS2_PLACEMENT_3D ( 'NONE', #3516, #3191, #3658 ) ;
#10782=CARTESIAN_POINT ( 'NONE',  ( -36.52757395963737963, 2.413203405699283710, -4.840238007535727860 ) ) ;
#10783=CARTESIAN_POINT ( 'NONE',  ( 15.49676243306308621, 3.102491976071176882, -4.173461118157685057 ) ) ;
#10788=CARTESIAN_POINT ( 'NONE',  ( 47.00305898648056768, -4.143816080048276618, 1.075455348895917762 ) ) ;
#10789=ORIENTED_EDGE ( 'NONE', *, *, #24374, .F. ) ;
#10794=CARTESIAN_POINT ( 'NONE',  ( 58.50000000000001421, 0.8156862745098042433, 2.468735688885369317 ) ) ;
#10801=AXIS2_PLACEMENT_3D ( 'NONE', #31042, #19030, #20782 ) ;
#10802=VERTEX_POINT ( 'NONE', #867 ) ;
#10807=CARTESIAN_POINT ( 'NONE',  ( 57.03559403007977124, 0.7482252654948684523, 2.422430812887707230 ) ) ;
#10809=DIRECTION ( 'NONE',  ( 1.387778780781445676E-14, -1.734723475976807094E-15, 1.000000000000000000 ) ) ;
#10811=B_SPLINE_CURVE_WITH_KNOTS ( 'NONE', 3,
 ( #20484, #25686, #8583, #20180, #22860, #15723, #29964, #18264, #3377, #22709, #18114, #1148, #15863, #3989, #13027, #27902 ),
 .UNSPECIFIED., .F., .F.,
 ( 4, 3, 3, 3, 3, 4 ),
 ( 0.000000000000000000, 1.391268354954338704E-05, 4.880039988305115829E-05, 8.637315450940535953E-05, 0.0001246458323646918982, 0.0001626605312951481396 ),
 .UNSPECIFIED. ) ;
#10817=CARTESIAN_POINT ( 'NONE',  ( -54.46462222424374033, 1.502185874895793694, -3.301501926143237675 ) ) ;
#10818=DIRECTION ( 'NONE',  ( 1.000000000000000000, 0.000000000000000000, 0.000000000000000000 ) ) ;
#10819=EDGE_CURVE ( 'NONE', #24615, #28796, #10150, .T. ) ;
#10820=AXIS2_PLACEMENT_3D ( 'NONE', #26609, #475, #14731 ) ;
#10829=DIRECTION ( 'NONE',  ( 1.520093157366878429E-16, -0.5877852522924742473, 0.8090169943749465631 ) ) ;
#10832=EDGE_LOOP ( 'NONE', ( #5056, #30492, #22572, #8653 ) ) ;
#10840=DIRECTION ( 'NONE',  ( 1.000000000000000000, 0.000000000000000000, 0.000000000000000000 ) ) ;
#10842=LINE ( 'NONE', #22748, #22338 ) ;
#10845=CARTESIAN_POINT ( 'NONE',  ( 15.71019289815287578, 2.413203405699197557, 4.840238007535781151 ) ) ;
#10846=FACE_OUTER_BOUND ( 'NONE', #6571, .T. ) ;
#10853=DIRECTION ( 'NONE',  ( 0.000000000000000000, 0.000000000000000000, -1.000000000000000000 ) ) ;
#10854=ORIENTED_EDGE ( 'NONE', *, *, #25138, .T. ) ;
#10856=AXIS2_PLACEMENT_3D ( 'NONE', #2136, #7064, #26042 ) ;
#10858=ORIENTED_EDGE ( 'NONE', *, *, #8251, .T. ) ;
#10864=CARTESIAN_POINT ( 'NONE',  ( -44.49999999999999289, 0.000000000000000000, 2.168404344971008868E-14 ) ) ;
#10872=DIRECTION ( 'NONE',  ( 0.000000000000000000, 0.000000000000000000, -1.000000000000000000 ) ) ;
#10875=FACE_OUTER_BOUND ( 'NONE', #4540, .T. ) ;
#10877=CARTESIAN_POINT ( 'NONE',  ( -36.42771574642738841, 4.977801270594329530, -2.126472881633125755 ) ) ;
#10879=CARTESIAN_POINT ( 'NONE',  ( -36.52757395963738674, -2.413203405699269055, 4.840238007535756282 ) ) ;
#10886=VECTOR ( 'NONE', #10266, 1000.000000000000000 ) ;
#10892=EDGE_CURVE ( 'NONE', #18214, #25246, #20187, .T. ) ;
#10898=VERTEX_POINT ( 'NONE', #2341 ) ;
#10902=ORIENTED_EDGE ( 'NONE', *, *, #17181, .F. ) ;
#10913=CARTESIAN_POINT ( 'NONE',  ( -54.49999999999997868, -4.276948333784438283, -0.9210526315789476781 ) ) ;
#10917=AXIS2_PLACEMENT_3D ( 'NONE', #25298, #15940, #16118 ) ;
#10923=CARTESIAN_POINT ( 'NONE',  ( 15.03925126672127810, -0.4576450603546984852, 5.200000000000000178 ) ) ;
#10924=AXIS2_PLACEMENT_3D ( 'NONE', #13225, #10706, #10853 ) ;
#10927=AXIS2_PLACEMENT_3D ( 'NONE', #25232, #18131, #1019 ) ;
#10929=DIRECTION ( 'NONE',  ( 1.000000000000000000, -0.000000000000000000, -0.000000000000000000 ) ) ;
#10931=TOROIDAL_SURFACE ( 'NONE', #2846, 4.275000000000000355, 0.1000000000000000056 ) ;
#10936=VERTEX_POINT ( 'NONE', #30294 ) ;
#10940=CARTESIAN_POINT ( 'NONE',  ( 15.03925126672132784, 4.383220986679478237, 0.4611378927914913661 ) ) ;
#10946=CARTESIAN_POINT ( 'NONE',  ( 50.50000000000002132, -0.6462379109120509613, 4.048750000000023164 ) ) ;
#10947=EDGE_CURVE ( 'NONE', #26911, #30652, #12575, .T. ) ;
#10948=ORIENTED_EDGE ( 'NONE', *, *, #20145, .F. ) ;
#10949=DIRECTION ( 'NONE',  ( -1.000000000000000000, -0.000000000000000000, -0.000000000000000000 ) ) ;
#10950=ORIENTED_EDGE ( 'NONE', *, *, #9830, .F. ) ;
#10951=VECTOR ( 'NONE', #16601, 1000.000000000000000 ) ;
#10952=CARTESIAN_POINT ( 'NONE',  ( 15.70940947763170570, 2.412550141807490611, -4.840569432287314733 ) ) ;
#10955=CIRCLE ( 'NONE', #2867, 1.000000000000000000 ) ;
#10969=( BOUNDED_SURFACE ( )  B_SPLINE_SURFACE ( 3, 2, ( 
 ( #1230, #768, #2998 ),
 ( #22325, #10435, #20117 ),
 ( #613, #29749, #10274 ),
 ( #27218, #13388, #11046 ),
 ( #13098, #10877, #20565 ),
 ( #8978, #23246, #10727 ),
 ( #23397, #11341, #1383 ),
 ( #27834, #8658, #22929 ),
 ( #20870, #3918, #1215 ),
 ( #22788, #30197, #20725 ),
 ( #16116, #8513, #18192 ),
 ( #1076, #6143, #28301 ),
 ( #20408, #27675, #30497 ),
 ( #8802, #18339, #3748 ),
 ( #30352, #5997, #1536 ),
 ( #23087, #18653, #27974 ) ),
 .UNSPECIFIED., .F., .F., .F. ) 
 B_SPLINE_SURFACE_WITH_KNOTS ( ( 4, 2, 2, 2, 2, 2, 2, 4 ),
 ( 3, 3 ),
 ( 0.001780502285214233520, 0.002558945925323761160, 0.002753556835351143178, 0.002948167745378525197, 0.003337389565433289233, 0.003726611385488053270, 0.004115833205542817307, 0.004894276845652345380 ),
 ( 0.000000000000000000, 1.000000000000000000 ),
 .UNSPECIFIED. ) 
 GEOMETRIC_REPRESENTATION_ITEM ( )  RATIONAL_B_SPLINE_SURFACE ( (
 ( 1.000000000000000000, 0.9418517008537252710, 1.000000000000000000),
 ( 1.000000000000000000, 0.9417987965886061019, 1.000000000000000000),
 ( 1.000000000000000000, 0.9418198861732800520, 1.000000000000000000),
 ( 1.000000000000000000, 0.9434060303845909212, 1.000000000000000000),
 ( 1.000000000000000000, 0.9437939819948288900, 1.000000000000000000),
 ( 1.000000000000000000, 0.9445989566712711394, 1.000000000000000000),
 ( 1.000000000000000000, 0.9450169930049940881, 1.000000000000000000),
 ( 1.000000000000000000, 0.9461610507673398063, 1.000000000000000000),
 ( 1.000000000000000000, 0.9467217966426996201, 1.000000000000000000),
 ( 1.000000000000000000, 0.9467345476124578996, 1.000000000000000000),
 ( 1.000000000000000000, 0.9461964028053386766, 1.000000000000000000),
 ( 1.000000000000000000, 0.9446801822473422927, 1.000000000000000000),
 ( 1.000000000000000000, 0.9437582546536400496, 1.000000000000000000),
 ( 1.000000000000000000, 0.9418129560295983582, 1.000000000000000000),
 ( 1.000000000000000000, 0.9418016889777277578, 1.000000000000000000),
 ( 1.000000000000000000, 0.9418517008537247159, 1.000000000000000000) ) ) 
 REPRESENTATION_ITEM ( '' )  SURFACE ( )  );
#10970=DIRECTION ( 'NONE',  ( 1.000000000000000000, -0.000000000000000000, -0.000000000000000000 ) ) ;
#10972=CYLINDRICAL_SURFACE ( 'NONE', #26610, 3.200000000000000178 ) ;
#10975=CARTESIAN_POINT ( 'NONE',  ( -44.49999999999998579, 4.529787229198778726E-28, -0.7500000000000185407 ) ) ;
#10978=CIRCLE ( 'NONE', #28691, 4.100000000000022737 ) ;
#10986=DIRECTION ( 'NONE',  ( 0.000000000000000000, 0.000000000000000000, -1.000000000000000000 ) ) ;
#10988=VERTEX_POINT ( 'NONE', #6387 ) ;
#10991=AXIS2_PLACEMENT_3D ( 'NONE', #1706, #21228, #25944 ) ;
#10992=EDGE_LOOP ( 'NONE', ( #19122, #4750, #28323, #28078, #5939, #8820, #19927 ) ) ;
#11002=LINE ( 'NONE', #20683, #18222 ) ;
#11003=ORIENTED_EDGE ( 'NONE', *, *, #31306, .F. ) ;
#11005=AXIS2_PLACEMENT_3D ( 'NONE', #28298, #6606, #23545 ) ;
#11006=EDGE_CURVE ( 'NONE', #20370, #28796, #3488, .T. ) ;
#11008=ORIENTED_EDGE ( 'NONE', *, *, #7036, .F. ) ;
#11011=AXIS2_PLACEMENT_3D ( 'NONE', #2646, #24337, #22290 ) ;
#11012=DIRECTION ( 'NONE',  ( 1.000000000000000000, 0.000000000000000000, 0.000000000000000000 ) ) ;
#11025=FACE_OUTER_BOUND ( 'NONE', #12088, .T. ) ;
#11036=DIRECTION ( 'NONE',  ( -2.459562394685754633E-16, 0.9510565162951565288, -0.3090169943749382919 ) ) ;
#11043=DIRECTION ( 'NONE',  ( -1.000000000000000000, 0.000000000000000000, 0.000000000000000000 ) ) ;
#11044=CARTESIAN_POINT ( 'NONE',  ( -35.85663232820584767, 3.817150320980632561, 2.203324261490556157 ) ) ;
#11046=CARTESIAN_POINT ( 'NONE',  ( -36.21152527658243514, 4.855742670514289649, -1.883114206442289218 ) ) ;
#11047=EDGE_CURVE ( 'NONE', #11901, #16322, #23339, .T. ) ;
#11048=DIRECTION ( 'NONE',  ( 1.000000000000000000, 2.586136946169074517E-16, -0.000000000000000000 ) ) ;
#11049=ADVANCED_FACE ( 'NONE', ( #11282 ), #28539, .T. ) ;
#11054=CARTESIAN_POINT ( 'NONE',  ( 57.00000000000001421, -0.6999999999999999556, 1.820027472320129736 ) ) ;
#11063=ORIENTED_EDGE ( 'NONE', *, *, #19157, .T. ) ;
#11067=ORIENTED_EDGE ( 'NONE', *, *, #24260, .F. ) ;
#11069=CARTESIAN_POINT ( 'NONE',  ( 33.47623932017462778, 1.734723475976807094E-15, 0.000000000000000000 ) ) ;
#11071=CARTESIAN_POINT ( 'NONE',  ( 56.95000000000001705, 0.000000000000000000, 0.000000000000000000 ) ) ;
#11074=ORIENTED_EDGE ( 'NONE', *, *, #30476, .F. ) ;
#11076=DIRECTION ( 'NONE',  ( 1.983166172879301074E-16, 0.9119702176296790030, -0.4102564102564101312 ) ) ;
#11081=CIRCLE ( 'NONE', #12592, 5.338914163118009704 ) ;
#11083=CARTESIAN_POINT ( 'NONE',  ( 47.09347798666725282, -4.179189514726790122, -0.9999999999996743716 ) ) ;
#11084=CARTESIAN_POINT ( 'NONE',  ( -35.85663232820579793, 2.199885893005987914, -4.939696249117657700 ) ) ;
#11089=EDGE_CURVE ( 'NONE', #3444, #24741, #29051, .T. ) ;
#11101=ORIENTED_EDGE ( 'NONE', *, *, #27242, .F. ) ;
#11103=DIRECTION ( 'NONE',  ( -1.520093157366893960E-16, 0.5877852522924802425, -0.8090169943749422332 ) ) ;
#11106=EDGE_LOOP ( 'NONE', ( #30910, #15513, #11930, #30456 ) ) ;
#11115=CIRCLE ( 'NONE', #28825, 0.05000000000000143219 ) ;
#11117=CARTESIAN_POINT ( 'NONE',  ( 36.55000000000001847, 0.000000000000000000, 0.000000000000000000 ) ) ;
#11118=ORIENTED_EDGE ( 'NONE', *, *, #28274, .T. ) ;
#11120=AXIS2_PLACEMENT_3D ( 'NONE', #17633, #22706, #17936 ) ;
#11124=CARTESIAN_POINT ( 'NONE',  ( 56.99150396717417522, -0.7610778266783598811, -1.740907964752457904 ) ) ;
#11129=DIRECTION ( 'NONE',  ( 0.000000000000000000, -0.000000000000000000, -1.000000000000000000 ) ) ;
#11137=CARTESIAN_POINT ( 'NONE',  ( -36.00201293083839005, -1.123735532908842760, -5.289358697221507200 ) ) ;
#11138=AXIS2_PLACEMENT_3D ( 'NONE', #3423, #30312, #13351 ) ;
#11140=SPHERICAL_SURFACE ( 'NONE', #22005, 0.05000000000000000278 ) ;
#11145=ORIENTED_EDGE ( 'NONE', *, *, #27012, .T. ) ;
#11158=ORIENTED_EDGE ( 'NONE', *, *, #28082, .T. ) ;
#11185=CARTESIAN_POINT ( 'NONE',  ( -36.89250464418361020, 2.917650619476140239, 4.554978966839756005 ) ) ;
#11196=CARTESIAN_POINT ( 'NONE',  ( 36.50000000000002132, -0.7794871794871797155, -1.732743413496390161 ) ) ;
#11197=ADVANCED_FACE ( 'NONE', ( #22224 ), #17159, .T. ) ;
#11202=B_SPLINE_CURVE_WITH_KNOTS ( 'NONE', 3,
 ( #28795, #14212, #4708, #31315, #4871, #23888, #26736, #28940, #9651, #9491, #19305, #9941, #16616, #2178, #7107, #28474, #132, #12010, #21692 ),
 .UNSPECIFIED., .F., .F.,
 ( 4, 3, 3, 3, 3, 3, 4 ),
 ( -1.463115107851837610E-06, -2.117582368135750848E-22, 2.244303852771090691E-05, 4.060544239443321531E-05, 5.609829020924228863E-05, 7.063629490958457896E-05, 8.524507318609980048E-05 ),
 .UNSPECIFIED. ) ;
#11208=CARTESIAN_POINT ( 'NONE',  ( 58.45000000000001705, 0.7794871794871796045, 1.732743413496389939 ) ) ;
#11216=CARTESIAN_POINT ( 'NONE',  ( 48.50000000000002132, 1.409901620910219311, 3.850000000000021849 ) ) ;
#11217=ORIENTED_EDGE ( 'NONE', *, *, #21967, .F. ) ;
#11218=FACE_OUTER_BOUND ( 'NONE', #8917, .T. ) ;
#11225=CARTESIAN_POINT ( 'NONE',  ( 58.50000000000001421, 0.000000000000000000, 0.000000000000000000 ) ) ;
#11229=CARTESIAN_POINT ( 'NONE',  ( -54.48118151432741030, 1.510613940323803916, -4.037256667234632168 ) ) ;
#11230=VERTEX_POINT ( 'NONE', #820 ) ;
#11232=CARTESIAN_POINT ( 'NONE',  ( -36.31414349454749413, 3.010474646410376653, -4.240315621469644469 ) ) ;
#11245=PLANE ( 'NONE',  #6503 ) ;
#11246=TOROIDAL_SURFACE ( 'NONE', #28960, 4.650000000000000355, 0.05000000000000000278 ) ;
#11249=CARTESIAN_POINT ( 'NONE',  ( 15.39414421509789754, -5.035245099686910031, 1.330662535294788951 ) ) ;
#11250=EDGE_LOOP ( 'NONE', ( #8124, #282, #19422, #18354 ) ) ;
#11255=ORIENTED_EDGE ( 'NONE', *, *, #5257, .F. ) ;
#11257=ORIENTED_EDGE ( 'NONE', *, *, #23836, .F. ) ;
#11259=CARTESIAN_POINT ( 'NONE',  ( 54.40000000000001990, 0.000000000000000000, -3.200000000000000178 ) ) ;
#11271=CARTESIAN_POINT ( 'NONE',  ( -36.00201293083839715, 4.683225679163155242, -2.703237727951674607 ) ) ;
#11275=DIRECTION ( 'NONE',  ( 0.000000000000000000, 0.000000000000000000, 1.000000000000000000 ) ) ;
#11277=CARTESIAN_POINT ( 'NONE',  ( 56.98109951608436319, 0.7885528131279547770, 2.477553856021609491 ) ) ;
#11281=CARTESIAN_POINT ( 'NONE',  ( 58.45000000000001705, 0.000000000000000000, 0.000000000000000000 ) ) ;
#11282=FACE_OUTER_BOUND ( 'NONE', #2262, .T. ) ;
#11297=CARTESIAN_POINT ( 'NONE',  ( 57.05000000000001847, -0.7794871794871796045, -1.732743413496389939 ) ) ;
#11299=EDGE_LOOP ( 'NONE', ( #15687, #11597, #1208, #4161 ) ) ;
#11308=CARTESIAN_POINT ( 'NONE',  ( 57.00108727371435435, 0.7119914823645937529, -1.810661949215600863 ) ) ;
#11309=CARTESIAN_POINT ( 'NONE',  ( -36.56242893520548165, -3.003531019938339597, 4.498666779076304856 ) ) ;
#11315=CARTESIAN_POINT ( 'NONE',  ( 48.30000000000001847, -0.6462379109120514054, -4.048750000000023164 ) ) ;
#11327=CARTESIAN_POINT ( 'NONE',  ( -36.77443515226919857, 2.672993279333530925, 4.702725322014869924 ) ) ;
#11328=ORIENTED_EDGE ( 'NONE', *, *, #23721, .F. ) ;
#11336=CARTESIAN_POINT ( 'NONE',  ( 51.80000000000001847, -3.726179070414207928, 1.710435481158852244 ) ) ;
#11339=ORIENTED_EDGE ( 'NONE', *, *, #19091, .F. ) ;
#11341=CARTESIAN_POINT ( 'NONE',  ( -36.50489844130380135, 5.024465639092071889, -2.007392901578094691 ) ) ;
#11343=CARTESIAN_POINT ( 'NONE',  ( -54.49999477219272848, -1.549165129012789466, -3.331602747802265174 ) ) ;
#11344=CARTESIAN_POINT ( 'NONE',  ( 56.95000053796676553, 0.7321038892619347038, 1.754109389045036771 ) ) ;
#11346=AXIS2_PLACEMENT_3D ( 'NONE', #31326, #9666, #24223 ) ;
#11348=CARTESIAN_POINT ( 'NONE',  ( 51.85600457075751990, 0.1551120032652606173, 4.362278500573884443 ) ) ;
#11350=CARTESIAN_POINT ( 'NONE',  ( 50.41049980741060921, 0.7811435014051845149, -4.027217152858574956 ) ) ;
#11351=VECTOR ( 'NONE', #29366, 1000.000000000000000 ) ;
#11360=DIRECTION ( 'NONE',  ( 1.000000000000000000, -0.000000000000000000, -0.000000000000000000 ) ) ;
#11363=CARTESIAN_POINT ( 'NONE',  ( 48.30268563551750560, 0.9333771270347341886, -3.994943142064453667 ) ) ;
#11364=ORIENTED_EDGE ( 'NONE', *, *, #8014, .F. ) ;
#11370=PRODUCT ( 'Body', 'Body', '', ( #5555 ) ) ;
#11376=DIRECTION ( 'NONE',  ( -0.000000000000000000, 0.000000000000000000, 1.000000000000000000 ) ) ;
#11380=CARTESIAN_POINT ( 'NONE',  ( -36.14490256869204643, 2.228039998204367933, 4.927410888447855797 ) ) ;
#11385=DIRECTION ( 'NONE',  ( 0.000000000000000000, 0.000000000000000000, -1.000000000000000000 ) ) ;
#11387=ORIENTED_EDGE ( 'NONE', *, *, #20324, .T. ) ;
#11389=CARTESIAN_POINT ( 'NONE',  ( 57.04534525700438508, -0.7498361808180106225, 1.778489416763646025 ) ) ;
#11390=AXIS2_PLACEMENT_3D ( 'NONE', #30069, #30711, #23432 ) ;
#11391=ADVANCED_FACE ( 'NONE', ( #21565 ), #3657, .T. ) ;
#11392=CARTESIAN_POINT ( 'NONE',  ( -36.39645873810205501, 2.743848709681631970, -4.666930520580605979 ) ) ;
#11395=CARTESIAN_POINT ( 'NONE',  ( 15.97944027357902108, 0.5584590966806891599, -5.380195666604552507 ) ) ;
#11398=ADVANCED_FACE ( 'NONE', ( #11581 ), #19346, .T. ) ;
#11401=LINE ( 'NONE', #25966, #2869 ) ;
#11402=CARTESIAN_POINT ( 'NONE',  ( 50.31565037626138803, -1.386108502191528924, -3.851082811767820413 ) ) ;
#11406=DIRECTION ( 'NONE',  ( -1.000000000000000000, -0.000000000000000000, 0.000000000000000000 ) ) ;
#11408=CARTESIAN_POINT ( 'NONE',  ( -36.58413561666694847, 5.110933801299781365, 1.769007076670967793 ) ) ;
#11409=CARTESIAN_POINT ( 'NONE',  ( 15.49702763512081560, -4.928592478218981832, 1.658905555082623717 ) ) ;
#11410=B_SPLINE_CURVE_WITH_KNOTS ( 'NONE', 3,
 ( #43, #31234, #19676, #24715, #5096, #16833, #14746, #26471, #19515, #5402, #29315, #9706, #343, #26930, #29453, #22206, #4772, #24406, #7627 ),
 .UNSPECIFIED., .F., .F.,
 ( 4, 3, 3, 3, 3, 3, 4 ),
 ( -1.485273975135398565E-06, 0.000000000000000000, 2.074191569004160408E-05, 3.882553518188197389E-05, 5.450508821808563542E-05, 6.929665250580404950E-05, 8.415228772525318584E-05 ),
 .UNSPECIFIED. ) ;
#11414=CARTESIAN_POINT ( 'NONE',  ( 48.50000000000002132, 1.426739617975221641, 3.843750000000023093 ) ) ;
#11415=CARTESIAN_POINT ( 'NONE',  ( 50.38699024846546592, -1.088846059295756286, 3.899771020632008423 ) ) ;
#11417=VERTEX_POINT ( 'NONE', #13925 ) ;
#11419=DIRECTION ( 'NONE',  ( 1.000000000000000000, 8.626663965456006092E-17, 1.494526870159786164E-16 ) ) ;
#11420=ORIENTED_EDGE ( 'NONE', *, *, #12981, .T. ) ;
#11421=CARTESIAN_POINT ( 'NONE',  ( 57.05000000000001847, 0.8000000000000000444, 2.471260002560649927 ) ) ;
#11427=ADVANCED_FACE ( 'NONE', ( #23622 ), #21881, .T. ) ;
#11442=CARTESIAN_POINT ( 'NONE',  ( -36.40793637698146767, 5.360541651686750342, -0.7128348320083691680 ) ) ;
#11446=CARTESIAN_POINT ( 'NONE',  ( -36.92405921417685732, -3.294441450831190110, -4.290383166762150147 ) ) ;
#11451=CARTESIAN_POINT ( 'NONE',  ( 50.31550977796903368, 1.386241252175322014, -3.851058308531627450 ) ) ;
#11454=CARTESIAN_POINT ( 'NONE',  ( 48.46963600013424411, -1.366688880095576319, -3.854642372925540350 ) ) ;
#11456=LINE ( 'NONE', #21141, #28117 ) ;
#11460=DIRECTION ( 'NONE',  ( 1.000000000000000000, 0.000000000000000000, 0.000000000000000000 ) ) ;
#11468=AXIS2_PLACEMENT_3D ( 'NONE', #10553, #12904, #22430 ) ;
#11473=AXIS2_PLACEMENT_3D ( 'NONE', #19567, #22721, #10809 ) ;
#11475=DIRECTION ( 'NONE',  ( 1.000000000000000000, -0.000000000000000000, -0.000000000000000000 ) ) ;
#11476=CARTESIAN_POINT ( 'NONE',  ( 33.47623932017462778, 4.375000000000001776, 5.357829746269670620E-16 ) ) ;
#11477=ORIENTED_EDGE ( 'NONE', *, *, #3503, .F. ) ;
#11489=AXIS2_PLACEMENT_3D ( 'NONE', #30260, #27564, #27886 ) ;
#11490=CARTESIAN_POINT ( 'NONE',  ( 57.05000000000001847, 0.7500000000000000000, -1.778341924377873751 ) ) ;
#11498=CARTESIAN_POINT ( 'NONE',  ( 15.03925126672132961, 2.686240680702206785, -4.475885388010691912 ) ) ;
#11503=VERTEX_POINT ( 'NONE', #27056 ) ;
#11505=VERTEX_POINT ( 'NONE', #5541 ) ;
#11509=CARTESIAN_POINT ( 'NONE',  ( -36.56242893520592219, 3.350344226587738561, 4.246692235171849461 ) ) ;
#11511=ORIENTED_EDGE ( 'NONE', *, *, #1270, .T. ) ;
#11516=DIRECTION ( 'NONE',  ( 0.000000000000000000, 0.000000000000000000, -1.000000000000000000 ) ) ;
#11518=ORIENTED_EDGE ( 'NONE', *, *, #23721, .T. ) ;
#11519=CARTESIAN_POINT ( 'NONE',  ( 50.37798322691364916, 1.327156576403631272, 3.879406274192440218 ) ) ;
#11525=CARTESIAN_POINT ( 'NONE',  ( -54.49999999999997868, -1.549582583372307809, -3.331868970650947226 ) ) ;
#11526=CARTESIAN_POINT ( 'NONE',  ( -37.18272003341174781, -5.407411300779149776, 6.622168941172400026E-16 ) ) ;
#11528=CARTESIAN_POINT ( 'NONE',  ( 51.80351136591793448, 1.029101438728343254, 4.191235921151213795 ) ) ;
#11529=CARTESIAN_POINT ( 'NONE',  ( 15.29449157529459136, 3.378578820314266817, 3.972872285093464129 ) ) ;
#11534=ADVANCED_FACE ( 'NONE', ( #5374 ), #3008, .T. ) ;
#11538=ORIENTED_EDGE ( 'NONE', *, *, #6394, .F. ) ;
#11541=CARTESIAN_POINT ( 'NONE',  ( -36.56242893520594350, 0.2143423494566060183, 5.404929114625701914 ) ) ;
#11547=PLANE ( 'NONE',  #17191 ) ;
#11548=ADVANCED_FACE ( 'NONE', ( #24241 ), #3002, .T. ) ;
#11551=B_SPLINE_CURVE_WITH_KNOTS ( 'NONE', 3,
 ( #26523, #30966, #24166, #19415, #7368, #17047, #5424, #15080, #1830, #11659, #21183, #9130, #18948, #26221, #25031, #10492 ),
 .UNSPECIFIED., .F., .F.,
 ( 4, 2, 2, 2, 2, 2, 2, 4 ),
 ( 5.358925739243605177E-21, 2.526926994603774344E-05, 5.053853989207548011E-05, 0.0001010770797841452004, 0.0002021541595682849798, 0.0004043083191365616112, 0.0008086166382731149824, 0.001617233276546221291 ),
 .UNSPECIFIED. ) ;
#11560=ADVANCED_FACE ( 'NONE', ( #15194 ), #25240, .T. ) ;
#11561=DIRECTION ( 'NONE',  ( 0.000000000000000000, 0.000000000000000000, -1.000000000000000000 ) ) ;
#11562=DIRECTION ( 'NONE',  ( -1.000000000000000000, -0.000000000000000000, 0.000000000000000000 ) ) ;
#11563=EDGE_CURVE ( 'NONE', #4137, #31086, #26767, .T. ) ;
#11568=CARTESIAN_POINT ( 'NONE',  ( -36.22818246778666662, 2.595266697484551521, -4.757426534476516089 ) ) ;
#11569=CARTESIAN_POINT ( 'NONE',  ( 48.34282069333976040, 1.210123066480781606, -3.917958458743180827 ) ) ;
#11575=CARTESIAN_POINT ( 'NONE',  ( 50.34137136386935651, -1.344608935533137206, -3.858631320448701718 ) ) ;
#11576=ORIENTED_EDGE ( 'NONE', *, *, #6628, .F. ) ;
#11579=DIRECTION ( 'NONE',  ( -0.000000000000000000, 1.000000000000000000, 0.000000000000000000 ) ) ;
#11581=FACE_OUTER_BOUND ( 'NONE', #30180, .T. ) ;
#11582=CARTESIAN_POINT ( 'NONE',  ( 15.74652664997095286, -5.076023720898155567, 1.868859051106972036 ) ) ;
#11585=ORIENTED_EDGE ( 'NONE', *, *, #10250, .F. ) ;
#11586=CARTESIAN_POINT ( 'NONE',  ( 15.03925126672132961, -2.199885893005931070, -4.939696249117691451 ) ) ;
#11587=CARTESIAN_POINT ( 'NONE',  ( 50.32622512580983454, -1.373801017329605578, 3.853344662332956361 ) ) ;
#11588=ORIENTED_EDGE ( 'NONE', *, *, #3028, .T. ) ;
#11596=DIRECTION ( 'NONE',  ( 1.000000000000000000, 0.000000000000000000, 0.000000000000000000 ) ) ;
#11597=ORIENTED_EDGE ( 'NONE', *, *, #708, .T. ) ;
#11603=CARTESIAN_POINT ( 'NONE',  ( 56.99824518417612751, -0.8016297048612398557, 2.473345119325445651 ) ) ;
#11608=CARTESIAN_POINT ( 'NONE',  ( 47.10000000000002984, -4.276948333784437395, 0.9210526315789471230 ) ) ;
#11610=CARTESIAN_POINT ( 'NONE',  ( -36.89831264271882105, -3.408535483610560579, -4.200031884472264387 ) ) ;
#11611=CARTESIAN_POINT ( 'NONE',  ( 56.95206911348624601, 0.7375298837344119729, 2.493227876267903653 ) ) ;
#11612=DIRECTION ( 'NONE',  ( 0.000000000000000000, 4.440892098500626951E-15, -1.000000000000000000 ) ) ;
#11613=VECTOR ( 'NONE', #325, 1000.000000000000000 ) ;
#11617=CARTESIAN_POINT ( 'NONE',  ( 48.40115653635459125, -0.8930148142854139603, -3.925689827643446428 ) ) ;
#11622=AXIS2_PLACEMENT_3D ( 'NONE', #9948, #5185, #12458 ) ;
#11630=VERTEX_POINT ( 'NONE', #27525 ) ;
#11631=CARTESIAN_POINT ( 'NONE',  ( 15.29954477411523506, 4.683225668089404437, 2.703237747136276070 ) ) ;
#11635=ORIENTED_EDGE ( 'NONE', *, *, #540, .F. ) ;
#11641=EDGE_CURVE ( 'NONE', #14026, #4137, #25168, .T. ) ;
#11642=CARTESIAN_POINT ( 'NONE',  ( 15.03925126672132784, 4.383220986679485343, -0.4611378927914090986 ) ) ;
#11649=CARTESIAN_POINT ( 'NONE',  ( -35.85663232820581925, -2.686240680702169481, 4.475885388010719446 ) ) ;
#11650=CARTESIAN_POINT ( 'NONE',  ( 15.03925126672132961, -4.018128179617543871, 3.618665901676652918 ) ) ;
#11655=CARTESIAN_POINT ( 'NONE',  ( 47.10000000000002274, -4.276948333784438283, 0.9210526315789470120 ) ) ;
#11657=ORIENTED_EDGE ( 'NONE', *, *, #15444, .T. ) ;
#11659=CARTESIAN_POINT ( 'NONE',  ( 51.84418490562190129, 0.2543151237804266995, -4.351520533650278466 ) ) ;
#11671=ORIENTED_EDGE ( 'NONE', *, *, #9233, .T. ) ;
#11673=CARTESIAN_POINT ( 'NONE',  ( -35.85663232820584057, -2.199885893005967041, 4.939696249117680793 ) ) ;
#11674=ORIENTED_EDGE ( 'NONE', *, *, #26865, .T. ) ;
#11678=EDGE_CURVE ( 'NONE', #15593, #4345, #20432, .T. ) ;
#11679=CARTESIAN_POINT ( 'NONE',  ( -54.46462222424374033, -1.502185874895793694, -3.301501926143236787 ) ) ;
#11687=VERTEX_POINT ( 'NONE', #20593 ) ;
#11688=CARTESIAN_POINT ( 'NONE',  ( 58.45000000000001705, 0.8000000000000000444, 2.421260002560649660 ) ) ;
#11689=CARTESIAN_POINT ( 'NONE',  ( -36.50489844130379424, 0.3564988296780842725, 5.398869307934828221 ) ) ;
#11693=CARTESIAN_POINT ( 'NONE',  ( 47.00000000000002132, 2.428612866367529932E-14, 0.000000000000000000 ) ) ;
#11695=EDGE_CURVE ( 'NONE', #20184, #25246, #18704, .T. ) ;
#11708=CARTESIAN_POINT ( 'NONE',  ( -36.00197790576392265, 2.199885893005899096, 4.939696249117698557 ) ) ;
#11714=CARTESIAN_POINT ( 'NONE',  ( -54.46439202372638277, 1.502116081466616793, -4.031358338852112588 ) ) ;
#11717=CARTESIAN_POINT ( 'NONE',  ( -36.89017861347080185, 2.910597594660179421, -4.559461819278051387 ) ) ;
#11720=EDGE_CURVE ( 'NONE', #28796, #10216, #15961, .T. ) ;
#11721=CARTESIAN_POINT ( 'NONE',  ( 57.00797408584070070, -0.7277374606022131154, -2.435538690626270597 ) ) ;
#11728=ORIENTED_EDGE ( 'NONE', *, *, #18038, .F. ) ;
#11733=FACE_OUTER_BOUND ( 'NONE', #24885, .T. ) ;
#11734=CARTESIAN_POINT ( 'NONE',  ( 15.03925126672125856, -2.525801270006271082, -4.794550352686344219 ) ) ;
#11735=CARTESIAN_POINT ( 'NONE',  ( -35.98952425903310370, 5.086913993735653783, 1.171642046065924481 ) ) ;
#11736=CARTESIAN_POINT ( 'NONE',  ( 15.61033468494287924, -5.277035221755875583, 1.205525476379309735 ) ) ;
#11739=LINE ( 'NONE', #28365, #16900 ) ;
#11741=CARTESIAN_POINT ( 'NONE',  ( 56.98981708175836758, 0.7951539052630037796, -2.475425269917271187 ) ) ;
#11742=DIRECTION ( 'NONE',  ( 0.000000000000000000, -0.2745098039215673746, -0.9615843008030769967 ) ) ;
#11749=ORIENTED_EDGE ( 'NONE', *, *, #19270, .F. ) ;
#11758=EDGE_CURVE ( 'NONE', #30450, #19424, #14061, .T. ) ;
#11760=VECTOR ( 'NONE', #9333, 1000.000000000000000 ) ;
#11761=CARTESIAN_POINT ( 'NONE',  ( 47.00000000000002132, -4.227689052994015206, 1.125730994152047026 ) ) ;
#11762=DIRECTION ( 'NONE',  ( 0.000000000000000000, 0.000000000000000000, -1.000000000000000000 ) ) ;
#11763=ORIENTED_EDGE ( 'NONE', *, *, #18125, .F. ) ;
#11764=DIRECTION ( 'NONE',  ( 0.000000000000000000, 0.000000000000000000, 1.000000000000000000 ) ) ;
#11766=CARTESIAN_POINT ( 'NONE',  ( 33.47623932017462778, 1.734723475976807094E-15, 0.000000000000000000 ) ) ;
#11769=CARTESIAN_POINT ( 'NONE',  ( 50.36581974271289397, -1.399739523915384698, 3.853780793998482945 ) ) ;
#11771=ADVANCED_FACE ( 'NONE', ( #7111 ), #14368, .F. ) ;
#11773=EDGE_LOOP ( 'NONE', ( #27705, #14338, #25948, #30270 ) ) ;
#11774=DIRECTION ( 'NONE',  ( -1.000000000000000000, 0.000000000000000000, 0.000000000000000000 ) ) ;
#11777=ORIENTED_EDGE ( 'NONE', *, *, #12126, .T. ) ;
#11780=EDGE_LOOP ( 'NONE', ( #18926, #11815, #11585, #26991 ) ) ;
#11786=CARTESIAN_POINT ( 'NONE',  ( 36.50000000000002132, -0.7794871794871797155, 1.732743413496390161 ) ) ;
#11789=ORIENTED_EDGE ( 'NONE', *, *, #324, .T. ) ;
#11795=ADVANCED_FACE ( 'NONE', ( #21377 ), #11547, .T. ) ;
#11811=CARTESIAN_POINT ( 'NONE',  ( 56.95000000000001705, 0.000000000000000000, -1.899999999999999911 ) ) ;
#11815=ORIENTED_EDGE ( 'NONE', *, *, #6365, .F. ) ;
#11816=ORIENTED_EDGE ( 'NONE', *, *, #14041, .T. ) ;
#11821=CARTESIAN_POINT ( 'NONE',  ( 50.50000000000001421, 0.6462379109120994780, 4.048750000000022276 ) ) ;
#11822=CARTESIAN_POINT ( 'NONE',  ( -35.85663232820584057, 4.945493884734801782, -1.606888370749687933 ) ) ;
#11825=CARTESIAN_POINT ( 'NONE',  ( 57.03513260258041839, 0.7477432062408043700, 1.780365573899210574 ) ) ;
#11826=CARTESIAN_POINT ( 'NONE',  ( -54.48531357662248809, -1.514292094527452504, -3.309285685900293483 ) ) ;
#11830=EDGE_CURVE ( 'NONE', #26302, #24008, #4412, .T. ) ;
#11832=EDGE_CURVE ( 'NONE', #13515, #22777, #24259, .T. ) ;
#11833=CARTESIAN_POINT ( 'NONE',  ( -54.44999999999997442, 1.499999999999999556, -4.029888335921975262 ) ) ;
#11835=CARTESIAN_POINT ( 'NONE',  ( 57.00000000000001421, -0.7500000000000000000, 3.499999999999999556 ) ) ;
#11837=CARTESIAN_POINT ( 'NONE',  ( -35.85663232820584057, -1.123735532908286316, 5.289358697221548944 ) ) ;
#11840=CARTESIAN_POINT ( 'NONE',  ( -36.63359589171323449, 0.7811288459610937762, 5.350925378100968466 ) ) ;
#11842=ORIENTED_EDGE ( 'NONE', *, *, #8184, .T. ) ;
#11846=AXIS2_PLACEMENT_3D ( 'NONE', #23894, #24042, #19164 ) ;
#11851=DIRECTION ( 'NONE',  ( 0.000000000000000000, 0.000000000000000000, -1.000000000000000000 ) ) ;
#11853=FACE_OUTER_BOUND ( 'NONE', #15251, .T. ) ;
#11856=AXIS2_PLACEMENT_3D ( 'NONE', #26279, #28340, #2199 ) ;
#11863=AXIS2_PLACEMENT_3D ( 'NONE', #2625, #17197, #26841 ) ;
#11864=ORIENTED_EDGE ( 'NONE', *, *, #18991, .T. ) ;
#11869=CARTESIAN_POINT ( 'NONE',  ( 56.95000000000001705, 0.000000000000000000, 0.000000000000000000 ) ) ;
#11880=ADVANCED_FACE ( 'NONE', ( #27195 ), #16186, .T. ) ;
#11881=CARTESIAN_POINT ( 'NONE',  ( 34.50000000000001421, 3.918869757271530460E-16, 3.200000000000000178 ) ) ;
#11884=CARTESIAN_POINT ( 'NONE',  ( -36.58361892165972762, 5.175840503946175453, 1.569056257078830008 ) ) ;
#11885=CARTESIAN_POINT ( 'NONE',  ( 15.03925126672133494, -4.683225679163354194, 2.703237727951214975 ) ) ;
#11886=ORIENTED_EDGE ( 'NONE', *, *, #20186, .F. ) ;
#11890=EDGE_LOOP ( 'NONE', ( #10441, #3001, #19473, #17139 ) ) ;
#11891=CARTESIAN_POINT ( 'NONE',  ( 57.05000000000001847, 0.8156862745098041323, -2.468735688885368873 ) ) ;
#11893=CARTESIAN_POINT ( 'NONE',  ( 56.95000000000001705, -0.7000000000000000666, -2.452039967047845437 ) ) ;
#11894=EDGE_LOOP ( 'NONE', ( #3371, #15312, #14652, #13153 ) ) ;
#11898=ORIENTED_EDGE ( 'NONE', *, *, #10892, .T. ) ;
#11899=AXIS2_PLACEMENT_3D ( 'NONE', #26429, #28492, #9186 ) ;
#11900=VERTEX_POINT ( 'NONE', #27022 ) ;
#11901=VERTEX_POINT ( 'NONE', #22303 ) ;
#11905=CARTESIAN_POINT ( 'NONE',  ( 58.45000000000001705, -0.8000000000000002665, -2.421260002560650104 ) ) ;
#11906=CYLINDRICAL_SURFACE ( 'NONE', #27588, 4.700000000000000178 ) ;
#11907=ADVANCED_FACE ( 'NONE', ( #2518 ), #24495, .T. ) ;
#11912=DIRECTION ( 'NONE',  ( -1.000000000000000000, -2.586136946169074517E-16, 0.000000000000000000 ) ) ;
#11913=AXIS2_PLACEMENT_3D ( 'NONE', #23914, #9524, #16647 ) ;
#11915=DIRECTION ( 'NONE',  ( 1.000000000000000000, 4.939082069373447378E-17, 1.520093157366847861E-16 ) ) ;
#11916=CARTESIAN_POINT ( 'NONE',  ( -44.49999999999997868, -6.938893903907228378E-14, 0.000000000000000000 ) ) ;
#11920=CIRCLE ( 'NONE', #10917, 4.650000000000000355 ) ;
#11922=CARTESIAN_POINT ( 'NONE',  ( 48.39258289184584783, -1.342093792059618762, 3.874237195466570416 ) ) ;
#11930=ORIENTED_EDGE ( 'NONE', *, *, #12981, .F. ) ;
#11931=EDGE_CURVE ( 'NONE', #30450, #16732, #23265, .T. ) ;
#11934=CARTESIAN_POINT ( 'NONE',  ( 15.86395258069111414, 4.872718122832685239, 2.345308583460563590 ) ) ;
#11935=EDGE_LOOP ( 'NONE', ( #22188, #10854 ) ) ;
#11936=TOROIDAL_SURFACE ( 'NONE', #2817, 4.275000000000000355, 0.1000000000000000056 ) ;
#11944=ORIENTED_EDGE ( 'NONE', *, *, #16853, .F. ) ;
#11956=CARTESIAN_POINT ( 'NONE',  ( 56.95442145253466038, 0.7107037530308675244, 1.762072693003282398 ) ) ;
#11958=CARTESIAN_POINT ( 'NONE',  ( -35.85663232820584057, -1.793057972832186486, -4.026191436122056544 ) ) ;
#11959=DIRECTION ( 'NONE',  ( 1.000000000000000000, 0.000000000000000000, -0.000000000000000000 ) ) ;
#11960=AXIS2_PLACEMENT_3D ( 'NONE', #13078, #10236, #22602 ) ;
#11962=DIRECTION ( 'NONE',  ( 1.000000000000000000, -0.000000000000000000, -0.000000000000000000 ) ) ;
#11967=VERTEX_POINT ( 'NONE', #3736 ) ;
#11969=ORIENTED_EDGE ( 'NONE', *, *, #30124, .T. ) ;
#11971=CARTESIAN_POINT ( 'NONE',  ( 50.30000000000001847, 1.426739617975221641, -3.843750000000023093 ) ) ;
#11975=EDGE_LOOP ( 'NONE', ( #14358, #7740, #5118, #12478 ) ) ;
#11976=EDGE_CURVE ( 'NONE', #12204, #21976, #3534, .T. ) ;
#11985=B_SPLINE_CURVE_WITH_KNOTS ( 'NONE', 3,
 ( #29314, #22043, #24404, #27080, #29162, #341, #9704, #26790, #22204, #4769, #5400, #15058 ),
 .UNSPECIFIED., .F., .F.,
 ( 4, 2, 2, 2, 2, 4 ),
 ( 0.000000000000000000, 5.522938194211708289E-05, 0.0001104587638842341658, 0.0002209175277684793091, 0.0004418350555369705986, 0.0008836701110739516056 ),
 .UNSPECIFIED. ) ;
#11988=VECTOR ( 'NONE', #10818, 1000.000000000000000 ) ;
#11996=TOROIDAL_SURFACE ( 'NONE', #15947, 4.000000000000022204, 0.1000000000000000056 ) ;
#12003=DIRECTION ( 'NONE',  ( 0.000000000000000000, 0.000000000000000000, -1.000000000000000000 ) ) ;
#12010=CARTESIAN_POINT ( 'NONE',  ( -54.45487361440510909, 1.499999999999999556, 4.029888335921975262 ) ) ;
#12013=CARTESIAN_POINT ( 'NONE',  ( 15.76675455518219593, -0.1030603059131519339, -5.407440145940146436 ) ) ;
#12015=DIRECTION ( 'NONE',  ( -1.000000000000000000, 0.000000000000000000, 0.000000000000000000 ) ) ;
#12016=ORIENTED_EDGE ( 'NONE', *, *, #24316, .F. ) ;
#12019=EDGE_CURVE ( 'NONE', #10802, #20370, #20399, .T. ) ;
#12026=ORIENTED_EDGE ( 'NONE', *, *, #6616, .F. ) ;
#12028=DIRECTION ( 'NONE',  ( 0.000000000000000000, 0.000000000000000000, -1.000000000000000000 ) ) ;
#12034=AXIS2_PLACEMENT_3D ( 'NONE', #28054, #28706, #23469 ) ;
#12036=CIRCLE ( 'NONE', #6448, 0.09999999999999982514 ) ;
#12038=( BOUNDED_SURFACE ( )  B_SPLINE_SURFACE ( 3, 2, ( 
 ( #15228, #984, #12685 ),
 ( #5724, #22365, #8252 ),
 ( #15546, #27733, #17772 ),
 ( #20160, #25199, #3515 ),
 ( #8409, #18090, #6052 ),
 ( #3656, #13292, #10165 ),
 ( #29464, #7780, #29624 ),
 ( #17447, #655, #17615 ),
 ( #27260, #5578, #24874 ),
 ( #12832, #18390, #8562 ) ),
 .UNSPECIFIED., .F., .F., .F. ) 
 B_SPLINE_SURFACE_WITH_KNOTS ( ( 4, 2, 2, 2, 4 ),
 ( 3, 3 ),
 ( 0.0002526260074104870901, 0.0003606909493797115550, 0.0004687558913489359657, 0.0006848857752873848412, 0.001117145543164282592 ),
 ( 0.000000000000000000, 1.000000000000000000 ),
 .UNSPECIFIED. ) 
 GEOMETRIC_REPRESENTATION_ITEM ( )  RATIONAL_B_SPLINE_SURFACE ( (
 ( 1.000000000000000000, 0.9842509842511785179, 1.000000000000000000),
 ( 1.000000000000000000, 0.9838268088398964828, 1.000000000000000000),
 ( 1.000000000000000000, 0.9731519947952215199, 1.000000000000000000),
 ( 1.000000000000000000, 0.9499473078865533493, 1.000000000000000000),
 ( 1.000000000000000000, 0.9371632344323691521, 1.000000000000000000),
 ( 1.000000000000000000, 0.8981767195495000689, 1.000000000000000000),
 ( 1.000000000000000000, 0.8714317066438477255, 1.000000000000000000),
 ( 1.000000000000000000, 0.7945716934681549271, 1.000000000000000000),
 ( 1.000000000000000000, 0.7462340517456440558, 1.000000000000000000),
 ( 1.000000000000000000, 0.7071067811865505703, 1.000000000000000000) ) ) 
 REPRESENTATION_ITEM ( '' )  SURFACE ( )  );
#12040=CARTESIAN_POINT ( 'NONE',  ( 15.98305126557428935, -3.597789892641458209, 4.037455662930108602 ) ) ;
#12044=CARTESIAN_POINT ( 'NONE',  ( 57.00000000000001421, 0.7500000000000000000, 1.778341924377873751 ) ) ;
#12054=CARTESIAN_POINT ( 'NONE',  ( 15.61033468494288279, -2.777216423308003002, -4.646230875016937212 ) ) ;
#12055=CARTESIAN_POINT ( 'NONE',  ( -36.92362342067168868, 5.192953935288548095, 1.516181439821858268 ) ) ;
#12056=DIRECTION ( 'NONE',  ( -1.000000000000000000, -0.000000000000000000, -0.000000000000000000 ) ) ;
#12060=VECTOR ( 'NONE', #15165, 1000.000000000000000 ) ;
#12063=CARTESIAN_POINT ( 'NONE',  ( 56.96751809705963154, 0.7713737938325972987, -2.482938273535672646 ) ) ;
#12066=CARTESIAN_POINT ( 'NONE',  ( -36.38139716712353788, -4.735424960531383398, -2.618558234550535602 ) ) ;
#12071=VERTEX_POINT ( 'NONE', #8501 ) ;
#12073=EDGE_CURVE ( 'NONE', #19387, #9397, #30342, .T. ) ;
#12077=CARTESIAN_POINT ( 'NONE',  ( 51.70000000000001705, -4.276948333784438283, -0.9210526315789475671 ) ) ;
#12080=CIRCLE ( 'NONE', #7020, 0.04999999999999991257 ) ;
#12083=CARTESIAN_POINT ( 'NONE',  ( -36.58413561666693425, 0.1030603059130986848, -5.407440145940149989 ) ) ;
#12084=CARTESIAN_POINT ( 'NONE',  ( 47.03762875446323477, -4.256129153948961630, 1.015733033895002357 ) ) ;
#12085=CARTESIAN_POINT ( 'NONE',  ( -54.49999999999997868, 1.549999999999999600, 4.064480286580312907 ) ) ;
#12086=CARTESIAN_POINT ( 'NONE',  ( 54.47118315602192951, -0.0009370910484279708656, -4.346120462634435633 ) ) ;
#12088=EDGE_LOOP ( 'NONE', ( #14260, #19881, #14923, #26410 ) ) ;
#12091=CARTESIAN_POINT ( 'NONE',  ( 48.40000000000002700, -0.7707709757764150682, 3.938803467580344719 ) ) ;
#12095=LINE ( 'NONE', #17006, #13935 ) ;
#12100=EDGE_LOOP ( 'NONE', ( #6639, #25577, #29441 ) ) ;
#12103=EDGE_LOOP ( 'NONE', ( #13117, #3144, #10645, #7750 ) ) ;
#12107=DIRECTION ( 'NONE',  ( -8.673617379883787770E-15, 0.000000000000000000, 1.000000000000000000 ) ) ;
#12115=DIRECTION ( 'NONE',  ( 0.000000000000000000, 0.000000000000000000, 1.000000000000000000 ) ) ;
#12116=CARTESIAN_POINT ( 'NONE',  ( 15.03925126672132961, 2.199885893005992799, -4.939696249117662141 ) ) ;
#12118=CARTESIAN_POINT ( 'NONE',  ( -35.85663232820597557, -3.779372838781795529, 3.883777296072546736 ) ) ;
#12120=EDGE_CURVE ( 'NONE', #13545, #1571, #22776, .T. ) ;
#12121=CARTESIAN_POINT ( 'NONE',  ( 51.70000000000001705, -4.179189514726513899, 0.9999999999999995559 ) ) ;
#12122=CARTESIAN_POINT ( 'NONE',  ( 51.70000000000001705, -3.826179070414207573, 1.000000000000000222 ) ) ;
#12123=EDGE_LOOP ( 'NONE', ( #22946, #242, #16331 ) ) ;
#12124=AXIS2_PLACEMENT_3D ( 'NONE', #24926, #22742, #10688 ) ;
#12126=EDGE_CURVE ( 'NONE', #23664, #30343, #13118, .T. ) ;
#12128=ORIENTED_EDGE ( 'NONE', *, *, #24023, .T. ) ;
#12135=VERTEX_POINT ( 'NONE', #30972 ) ;
#12140=ORIENTED_EDGE ( 'NONE', *, *, #14158, .F. ) ;
#12141=CARTESIAN_POINT ( 'NONE',  ( -36.00201293083840426, 5.377732432866750401, 0.5657657256210959495 ) ) ;
#12145=VECTOR ( 'NONE', #29724, 1000.000000000000000 ) ;
#12146=EDGE_CURVE ( 'NONE', #3490, #3082, #30487, .T. ) ;
#12152=CARTESIAN_POINT ( 'NONE',  ( 50.42118334212123898, 1.311095223031216284, -3.884869838566831657 ) ) ;
#12153=ADVANCED_FACE ( 'NONE', ( #6599 ), #15220, .T. ) ;
#12154=CARTESIAN_POINT ( 'NONE',  ( 15.32766723174653656, -4.698774973472838568, -2.676767126782125583 ) ) ;
#12156=EDGE_CURVE ( 'NONE', #12911, #29967, #1020, .T. ) ;
#12158=CARTESIAN_POINT ( 'NONE',  ( 57.00000000000001421, -0.7000000000000006217, -2.452039967047844993 ) ) ;
#12163=CARTESIAN_POINT ( 'NONE',  ( -36.00197790576392265, -5.377732432866662471, 0.5657657256215433694 ) ) ;
#12167=CARTESIAN_POINT ( 'NONE',  ( -36.68133364217572989, -4.872718122832729648, 2.345308583460507190 ) ) ;
#12172=LINE ( 'NONE', #7422, #19107 ) ;
#12174=CARTESIAN_POINT ( 'NONE',  ( -54.49999999999997868, -1.549999999999999600, -4.064480286580312907 ) ) ;
#12175=ORIENTED_EDGE ( 'NONE', *, *, #11678, .T. ) ;
#12181=DIRECTION ( 'NONE',  ( -1.000000000000000000, -0.000000000000000000, -0.000000000000000000 ) ) ;
#12183=FACE_BOUND ( 'NONE', #6356, .T. ) ;
#12184=ORIENTED_EDGE ( 'NONE', *, *, #16717, .F. ) ;
#12185=CARTESIAN_POINT ( 'NONE',  ( 15.74652664997095286, -3.008101665203153807, 4.495550615867657918 ) ) ;
#12189=CIRCLE ( 'NONE', #8137, 0.09999999999999986677 ) ;
#12190=ADVANCED_FACE ( 'NONE', ( #29225 ), #12272, .F. ) ;
#12195=DIRECTION ( 'NONE',  ( 0.000000000000000000, 0.3137254901960787046, 0.9495137264943726008 ) ) ;
#12197=CARTESIAN_POINT ( 'NONE',  ( 50.36640492253748391, -1.250162886418155761, -3.874884102585953727 ) ) ;
#12203=FACE_OUTER_BOUND ( 'NONE', #368, .T. ) ;
#12204=VERTEX_POINT ( 'NONE', #14950 ) ;
#12206=AXIS2_PLACEMENT_3D ( 'NONE', #21221, #6630, #21053 ) ;
#12208=ORIENTED_EDGE ( 'NONE', *, *, #24035, .T. ) ;
#12210=FACE_OUTER_BOUND ( 'NONE', #19746, .T. ) ;
#12212=CARTESIAN_POINT ( 'NONE',  ( -35.85663232820580504, -5.340403872473343583, -0.9205822173396128738 ) ) ;
#12215=ORIENTED_EDGE ( 'NONE', *, *, #1559, .F. ) ;
#12224=AXIS2_PLACEMENT_3D ( 'NONE', #13718, #30669, #18028 ) ;
#12230=CARTESIAN_POINT ( 'NONE',  ( 15.95705409078463788, 4.926689578693635774, -2.233438676318118432 ) ) ;
#12235=CARTESIAN_POINT ( 'NONE',  ( 48.50000000000263611, -1.409901620923685206, 3.849999999997240518 ) ) ;
#12237=CARTESIAN_POINT ( 'NONE',  ( -35.85663232820584057, -5.086913985776155833, -1.171642053949114803 ) ) ;
#12247=CARTESIAN_POINT ( 'NONE',  ( 48.46953526341860652, -1.366509374015013600, 3.854674997130604908 ) ) ;
#12250=CARTESIAN_POINT ( 'NONE',  ( 54.45370770736469268, -0.0004837498569785767585, 4.360091688067994298 ) ) ;
#12255=CARTESIAN_POINT ( 'NONE',  ( -54.44999999999997442, -1.499999999999998668, 4.029888335921975262 ) ) ;
#12258=CARTESIAN_POINT ( 'NONE',  ( 57.01898512823798626, 0.7746824256175574019, 1.734896867090173211 ) ) ;
#12271=CARTESIAN_POINT ( 'NONE',  ( 16.00221665700882312, 5.295593823078800000, 1.114646847977682098 ) ) ;
#12272=PLANE ( 'NONE',  #10621 ) ;
#12274=ORIENTED_EDGE ( 'NONE', *, *, #5828, .T. ) ;
#12275=CARTESIAN_POINT ( 'NONE',  ( 58.45000000000001705, -0.8000000000000000444, 3.499999999999999556 ) ) ;
#12278=ORIENTED_EDGE ( 'NONE', *, *, #27542, .T. ) ;
#12285=EDGE_CURVE ( 'NONE', #24464, #31094, #13350, .T. ) ;
#12287=CARTESIAN_POINT ( 'NONE',  ( 50.36581974271289397, 1.399739523915438211, -3.853780793998481169 ) ) ;
#12290=DIRECTION ( 'NONE',  ( 0.000000000000000000, -1.000000000000000000, -0.000000000000000000 ) ) ;
#12292=EDGE_LOOP ( 'NONE', ( #9727, #26571, #16668, #25816 ) ) ;
#12294=CARTESIAN_POINT ( 'NONE',  ( -36.42771574642738130, -3.560621078037132570, -4.077054076718796161 ) ) ;
#12296=ORIENTED_EDGE ( 'NONE', *, *, #12393, .T. ) ;
#12299=VERTEX_POINT ( 'NONE', #3414 ) ;
#12301=CARTESIAN_POINT ( 'NONE',  ( -36.92443669619682112, -5.191204783933228484, 1.522159526382896866 ) ) ;
#12302=LINE ( 'NONE', #9947, #12986 ) ;
#12305=DIRECTION ( 'NONE',  ( 1.000000000000000000, 0.000000000000000000, 0.000000000000000000 ) ) ;
#12307=LINE ( 'NONE', #19776, #27685 ) ;
#12310=CIRCLE ( 'NONE', #15362, 4.786668705877438867 ) ;
#12313=EDGE_CURVE ( 'NONE', #4345, #473, #877, .T. ) ;
#12316=CARTESIAN_POINT ( 'NONE',  ( 51.80000000000001847, -0.1421112804877788793, -7.888760782825513275E-16 ) ) ;
#12319=ADVANCED_FACE ( 'NONE', ( #25397 ), #5469, .T. ) ;
#12321=EDGE_CURVE ( 'NONE', #3273, #17666, #5394, .T. ) ;
#12325=DIRECTION ( 'NONE',  ( 0.000000000000000000, 0.1576190026614809614, -0.9875000000000001554 ) ) ;
#12327=CIRCLE ( 'NONE', #10820, 2.600000000000000089 ) ;
#12336=CARTESIAN_POINT ( 'NONE',  ( 15.44631504820157808, -3.231775792180293649, -4.079530926931276724 ) ) ;
#12342=CARTESIAN_POINT ( 'NONE',  ( -53.99999999999997868, 5.755839955992559655E-16, -4.700000000000000178 ) ) ;
#12346=LINE ( 'NONE', #27066, #23005 ) ;
#12348=CARTESIAN_POINT ( 'NONE',  ( -36.42771574642760157, -5.277035221755912886, -1.205525476379292416 ) ) ;
#12359=FACE_OUTER_BOUND ( 'NONE', #14871, .T. ) ;
#12367=DIRECTION ( 'NONE',  ( -1.000000000000000000, -0.000000000000000000, -0.000000000000000000 ) ) ;
#12368=CARTESIAN_POINT ( 'NONE',  ( 15.03925126672132606, 4.861582140531648832, -2.394243978978272569 ) ) ;
#12372=B_SPLINE_CURVE_WITH_KNOTS ( 'NONE', 3,
 ( #25167, #2843, #29756, #12799, #22480, #22022, #315, #8073, #7608, #17263, #26908, #14866, #10135, #23115, #8826, #27856 ),
 .UNSPECIFIED., .F., .F.,
 ( 4, 3, 3, 3, 3, 4 ),
 ( 0.000000000000000000, 1.625241835515689952E-05, 3.292491922809579385E-05, 5.060195339673861708E-05, 6.961003767230190245E-05, 8.476187580399473969E-05 ),
 .UNSPECIFIED. ) ;
#12379=CARTESIAN_POINT ( 'NONE',  ( 50.30000000000001847, 1.426739617975221641, 3.843750000000023093 ) ) ;
#12382=CARTESIAN_POINT ( 'NONE',  ( 15.90468948301722918, -5.313409993919707475, 1.009519134730179291 ) ) ;
#12386=CARTESIAN_POINT ( 'NONE',  ( 15.18463186935387554, 5.377732432866777934, -0.5657657256209858154 ) ) ;
#12393=EDGE_CURVE ( 'NONE', #3627, #28219, #2374, .T. ) ;
#12399=DIRECTION ( 'NONE',  ( 1.000000000000000000, 0.000000000000000000, 0.000000000000000000 ) ) ;
#12404=EDGE_CURVE ( 'NONE', #27956, #16762, #21475, .T. ) ;
#12406=CARTESIAN_POINT ( 'NONE',  ( -36.38139716712170468, -3.953723660658932992, 3.694477770903708436 ) ) ;
#12407=FACE_BOUND ( 'NONE', #4091, .T. ) ;
#12408=CARTESIAN_POINT ( 'NONE',  ( 51.73137679800704802, -4.259946794064842557, 1.000000024775425711 ) ) ;
#12412=AXIS2_PLACEMENT_3D ( 'NONE', #18546, #16162, #4119 ) ;
#12431=ORIENTED_EDGE ( 'NONE', *, *, #25276, .F. ) ;
#12433=CARTESIAN_POINT ( 'NONE',  ( 46.90000000000001279, 1.734723475976807094E-15, 4.275000000000000355 ) ) ;
#12442=AXIS2_PLACEMENT_3D ( 'NONE', #28106, #25420, #13366 ) ;
#12444=CARTESIAN_POINT ( 'NONE',  ( 15.71019289815288644, -4.797343084509205546, -2.497389432263995346 ) ) ;
#12448=ORIENTED_EDGE ( 'NONE', *, *, #18730, .F. ) ;
#12450=EDGE_CURVE ( 'NONE', #28184, #6720, #6945, .T. ) ;
#12451=CARTESIAN_POINT ( 'NONE',  ( -36.04581030752635229, -2.525801262579533191, -4.794550356814626824 ) ) ;
#12454=CARTESIAN_POINT ( 'NONE',  ( 58.45000000000001705, -0.8000000000000000444, 1.778341924377873751 ) ) ;
#12458=DIRECTION ( 'NONE',  ( 0.000000000000000000, 0.000000000000000000, -1.000000000000000000 ) ) ;
#12460=VECTOR ( 'NONE', #14093, 1000.000000000000000 ) ;
#12464=DIRECTION ( 'NONE',  ( 1.000000000000000000, 0.000000000000000000, 0.000000000000000000 ) ) ;
#12470=AXIS2_PLACEMENT_3D ( 'NONE', #6623, #23409, #3510 ) ;
#12478=ORIENTED_EDGE ( 'NONE', *, *, #686, .T. ) ;
#12479=EDGE_CURVE ( 'NONE', #26012, #21420, #10978, .T. ) ;
#12495=TOROIDAL_SURFACE ( 'NONE', #2908, 2.649999999999999911, 0.05000000000000000278 ) ;
#12503=ADVANCED_FACE ( 'NONE', ( #9544 ), #23100, .T. ) ;
#12509=CIRCLE ( 'NONE', #23654, 2.600000000000000089 ) ;
#12511=CARTESIAN_POINT ( 'NONE',  ( -36.27260443516959043, -5.005099703116284715, -1.423440526321894328 ) ) ;
#12512=ORIENTED_EDGE ( 'NONE', *, *, #16390, .F. ) ;
#12515=CYLINDRICAL_SURFACE ( 'NONE', #24037, 0.1000000000000002554 ) ;
#12522=CARTESIAN_POINT ( 'NONE',  ( 48.38577482684819131, -1.132063507975290095, -3.941224428058327511 ) ) ;
#12523=DIRECTION ( 'NONE',  ( 0.000000000000000000, 0.000000000000000000, 1.000000000000000000 ) ) ;
#12524=CARTESIAN_POINT ( 'NONE',  ( 51.78960940689399450, -4.157292525004591788, -1.048498855808313035 ) ) ;
#12526=CARTESIAN_POINT ( 'NONE',  ( -36.56242893520685300, -0.2143423494565226961, -5.404929114625703690 ) ) ;
#12529=LINE ( 'NONE', #30684, #30672 ) ;
#12531=CARTESIAN_POINT ( 'NONE',  ( 54.50000000000002132, -0.003160834336494982005, -4.277587663180611344 ) ) ;
#12532=CARTESIAN_POINT ( 'NONE',  ( 57.05000000000002558, -0.7500000000000000000, 2.490438859776669123 ) ) ;
#12537=CARTESIAN_POINT ( 'NONE',  ( 15.17214319754864427, 3.426725954212534120, -3.937891351789542416 ) ) ;
#12539=DIRECTION ( 'NONE',  ( -1.000000000000000000, -0.000000000000000000, -0.000000000000000000 ) ) ;
#12542=EDGE_LOOP ( 'NONE', ( #27314, #16360, #2860, #12184 ) ) ;
#12543=CARTESIAN_POINT ( 'NONE',  ( 51.70000000000001705, -3.826179070414207573, 1.000000000000000222 ) ) ;
#12545=EDGE_LOOP ( 'NONE', ( #24322, #26187, #16409, #29338 ) ) ;
#12549=DIRECTION ( 'NONE',  ( -1.000000000000000000, -0.000000000000000000, -0.000000000000000000 ) ) ;
#12551=EDGE_LOOP ( 'NONE', ( #2682, #24927, #16484 ) ) ;
#12552=DIRECTION ( 'NONE',  ( 0.000000000000000000, -1.000000000000000000, 0.000000000000000000 ) ) ;
#12558=CARTESIAN_POINT ( 'NONE',  ( 51.72219788184018086, -4.178381389434671078, -1.001886780333043125 ) ) ;
#12559=CARTESIAN_POINT ( 'NONE',  ( -35.85663232820583346, -4.383220986679603470, -0.4611378927910509407 ) ) ;
#12561=CARTESIAN_POINT ( 'NONE',  ( 56.95000000000001705, -0.7137254901960785602, -2.500119182087999548 ) ) ;
#12562=CARTESIAN_POINT ( 'NONE',  ( 57.01550456668461209, -0.7366124869942373143, 2.429953032873097829 ) ) ;
#12563=CARTESIAN_POINT ( 'NONE',  ( -36.23324115033521053, -3.272294129011612540, 4.050092634494196098 ) ) ;
#12569=CARTESIAN_POINT ( 'NONE',  ( -54.49865678108456279, 1.537045020190657585, -3.323865043138458208 ) ) ;
#12574=EDGE_LOOP ( 'NONE', ( #16883, #6193, #23633, #9022 ) ) ;
#12575=CIRCLE ( 'NONE', #19193, 1.000000000000000000 ) ;
#12583=ORIENTED_EDGE ( 'NONE', *, *, #6084, .F. ) ;
#12587=DIRECTION ( 'NONE',  ( 0.000000000000000000, 0.000000000000000000, -1.000000000000000000 ) ) ;
#12590=ORIENTED_EDGE ( 'NONE', *, *, #4470, .T. ) ;
#12592=AXIS2_PLACEMENT_3D ( 'NONE', #5486, #16464, #9671 ) ;
#12595=CARTESIAN_POINT ( 'NONE',  ( 15.41586008885046866, -5.027926281937888042, -1.353187539902112491 ) ) ;
#12600=CARTESIAN_POINT ( 'NONE',  ( 48.30000000000001847, 0.6462379109120995890, -4.048750000000023164 ) ) ;
#12601=CYLINDRICAL_SURFACE ( 'NONE', #11468, 1.000000000000000000 ) ;
#12602=CARTESIAN_POINT ( 'NONE',  ( 50.40896409817930390, 1.199904535326282495, -3.921111011342365504 ) ) ;
#12605=DIRECTION ( 'NONE',  ( 0.000000000000000000, 0.000000000000000000, -1.000000000000000000 ) ) ;
#12606=EDGE_CURVE ( 'NONE', #12299, #26302, #18432, .T. ) ;
#12611=ORIENTED_EDGE ( 'NONE', *, *, #147, .F. ) ;
#12613=EDGE_LOOP ( 'NONE', ( #29641, #29301, #29190, #23958 ) ) ;
#12615=CARTESIAN_POINT ( 'NONE',  ( -35.85663232820584057, -0.4576450603547173035, -5.200000000000000178 ) ) ;
#12619=VECTOR ( 'NONE', #16443, 1000.000000000000000 ) ;
#12623=VERTEX_POINT ( 'NONE', #22033 ) ;
#12634=CARTESIAN_POINT ( 'NONE',  ( 15.59140265158956318, -0.9780988077348131693, 5.318542208600381294 ) ) ;
#12637=CARTESIAN_POINT ( 'NONE',  ( 15.61552784268253724, -2.776541361170953515, 4.646985486732154946 ) ) ;
#12639=EDGE_CURVE ( 'NONE', #11417, #8120, #1868, .T. ) ;
#12640=DIRECTION ( 'NONE',  ( -1.000000000000000000, -0.000000000000000000, -0.000000000000000000 ) ) ;
#12646=ORIENTED_EDGE ( 'NONE', *, *, #711, .T. ) ;
#12649=CARTESIAN_POINT ( 'NONE',  ( 16.07512358269907082, -3.430438802933840403, -4.182416543699102540 ) ) ;
#12652=ORIENTED_EDGE ( 'NONE', *, *, #2821, .F. ) ;
#12660=DIRECTION ( 'NONE',  ( -1.000000000000000000, -0.000000000000000000, -0.000000000000000000 ) ) ;
#12661=CARTESIAN_POINT ( 'NONE',  ( -36.89250464418362441, -5.037778396015640148, -1.970103387723705080 ) ) ;
#12665=EDGE_CURVE ( 'NONE', #13977, #13894, #25612, .T. ) ;
#12670=CARTESIAN_POINT ( 'NONE',  ( 48.42250533816334013, -1.328329461116573684, -3.879000873601222477 ) ) ;
#12671=CARTESIAN_POINT ( 'NONE',  ( 15.56274145962601807, -1.026563698233271538, 5.312790900508115755 ) ) ;
#12674=ADVANCED_FACE ( 'NONE', ( #6176 ), #855, .F. ) ;
#12676=CARTESIAN_POINT ( 'NONE',  ( -36.04518387042617888, -0.7747498539018073949, -5.363501450340010024 ) ) ;
#12678=EDGE_CURVE ( 'NONE', #10332, #19277, #25125, .T. ) ;
#12681=CARTESIAN_POINT ( 'NONE',  ( 54.46244440770933437, -0.0007103938888845436886, -4.353106894003209604 ) ) ;
#12682=CARTESIAN_POINT ( 'NONE',  ( 56.99368740573074632, -0.8156852809530760195, 2.468736017162952656 ) ) ;
#12685=CARTESIAN_POINT ( 'NONE',  ( 50.29999999999649418, -1.426739617988837194, -3.843749999997122746 ) ) ;
#12686=CARTESIAN_POINT ( 'NONE',  ( -36.40878371307407946, -5.360483378448159364, -0.7132926830812800212 ) ) ;
#12687=CARTESIAN_POINT ( 'NONE',  ( 15.30042582489635095, 2.199885882961221562, -4.939696253591084663 ) ) ;
#12689=CARTESIAN_POINT ( 'NONE',  ( 56.95000081403880188, 0.7675332364161941978, 2.484758330364432943 ) ) ;
#12692=CARTESIAN_POINT ( 'NONE',  ( 47.06748821295592933, -4.176834854957374610, 1.005432649909180132 ) ) ;
#12698=CARTESIAN_POINT ( 'NONE',  ( 15.32752150720752837, 4.698781674909530359, -2.676750094560090165 ) ) ;
#12699=ORIENTED_EDGE ( 'NONE', *, *, #502, .T. ) ;
#12702=ORIENTED_EDGE ( 'NONE', *, *, #28233, .T. ) ;
#12704=ORIENTED_EDGE ( 'NONE', *, *, #9624, .F. ) ;
#12705=DIRECTION ( 'NONE',  ( -1.000000000000000000, -2.586136946169074517E-16, 0.000000000000000000 ) ) ;
#12717=DIRECTION ( 'NONE',  ( 0.000000000000000000, 0.000000000000000000, -1.000000000000000000 ) ) ;
#12719=ADVANCED_BREP_SHAPE_REPRESENTATION ( '', ( #5173, #9018 ), #23745 ) ;
#12721=CARTESIAN_POINT ( 'NONE',  ( 50.40811050917465508, -1.340787288841403635, -3.874691554877328858 ) ) ;
#12725=CARTESIAN_POINT ( 'NONE',  ( 51.80000000000001847, -1.084202172485504434E-16, 4.374999999999999112 ) ) ;
#12733=DIRECTION ( 'NONE',  ( 1.000000000000000000, 0.000000000000000000, 0.000000000000000000 ) ) ;
#12734=DIRECTION ( 'NONE',  ( 0.000000000000000000, 0.000000000000000000, -1.000000000000000000 ) ) ;
#12740=ORIENTED_EDGE ( 'NONE', *, *, #20652, .F. ) ;
#12747=CARTESIAN_POINT ( 'NONE',  ( 15.98305126557417921, -4.951626736499063597, -2.174059107776757038 ) ) ;
#12753=DIRECTION ( 'NONE',  ( 0.000000000000000000, 1.000000000000000000, -1.224646799147353207E-16 ) ) ;
#12754=CARTESIAN_POINT ( 'NONE',  ( -36.22818246778668083, -3.722599991951390130, -3.938370952810070769 ) ) ;
#12756=DIRECTION ( 'NONE',  ( -1.520093157366893960E-16, 0.5877852522924802425, -0.8090169943749422332 ) ) ;
#12766=CARTESIAN_POINT ( 'NONE',  ( 15.41586008885046155, -0.2667568399899467591, -5.200000000294864755 ) ) ;
#12769=ORIENTED_EDGE ( 'NONE', *, *, #23398, .F. ) ;
#12771=LINE ( 'NONE', #17709, #3406 ) ;
#12774=CARTESIAN_POINT ( 'NONE',  ( -54.47328085509070661, -1.505517457405397774, -4.033720452520548783 ) ) ;
#12787=CARTESIAN_POINT ( 'NONE',  ( 15.61552784268253902, 3.561547362098769209, 4.076645242318642559 ) ) ;
#12790=DIRECTION ( 'NONE',  ( 0.000000000000000000, -1.000000000000000000, 0.000000000000000000 ) ) ;
#12792=FACE_OUTER_BOUND ( 'NONE', #24750, .T. ) ;
#12793=CARTESIAN_POINT ( 'NONE',  ( 48.39258289184584783, 1.342093792059667390, -3.874237195466570416 ) ) ;
#12794=ORIENTED_EDGE ( 'NONE', *, *, #19523, .T. ) ;
#12799=CARTESIAN_POINT ( 'NONE',  ( 57.03405126743467690, 0.7473881623357462312, -2.422979693216943176 ) ) ;
#12800=CARTESIAN_POINT ( 'NONE',  ( 19.23646557533807666, -1.947877022684209034E-15, 0.000000000000000000 ) ) ;
#12803=ORIENTED_EDGE ( 'NONE', *, *, #16390, .T. ) ;
#12813=EDGE_CURVE ( 'NONE', #21815, #23640, #28333, .T. ) ;
#12814=ORIENTED_EDGE ( 'NONE', *, *, #12073, .F. ) ;
#12819=CARTESIAN_POINT ( 'NONE',  ( 15.68751737981905947, -0.3564988296780420840, 5.398869307934826445 ) ) ;
#12821=ADVANCED_FACE ( 'NONE', ( #11853 ), #10461, .F. ) ;
#12827=CARTESIAN_POINT ( 'NONE',  ( 15.59055531549693896, -2.334444681449719283, 4.877899991435270977 ) ) ;
#12832=CARTESIAN_POINT ( 'NONE',  ( 50.40000000000001279, -0.6304760106459033064, -3.950000000000022826 ) ) ;
#12833=CARTESIAN_POINT ( 'NONE',  ( -43.84599839145305111, -4.786668705877446861, 6.082865895343455568E-16 ) ) ;
#12834=CARTESIAN_POINT ( 'NONE',  ( 15.03925126672122659, 4.018128179617576734, -3.618665901676609842 ) ) ;
#12839=CARTESIAN_POINT ( 'NONE',  ( 47.07780211815985894, -4.178381389434672855, 1.001886780333041571 ) ) ;
#12842=AXIS2_PLACEMENT_3D ( 'NONE', #5038, #14370, #19311 ) ;
#12843=CARTESIAN_POINT ( 'NONE',  ( 15.18459684427939749, -4.683225679163354194, 2.703237727951212754 ) ) ;
#12844=VERTEX_POINT ( 'NONE', #9012 ) ;
#12845=VERTEX_POINT ( 'NONE', #21531 ) ;
#12848=DIRECTION ( 'NONE',  ( 0.000000000000000000, 0.3137254901960767617, -0.9495137264943732669 ) ) ;
#12861=CARTESIAN_POINT ( 'NONE',  ( -54.44999999999997442, 1.549999999999999600, -4.029888335921975262 ) ) ;
#12862=CARTESIAN_POINT ( 'NONE',  ( 36.50000000000002132, 0.000000000000000000, 0.000000000000000000 ) ) ;
#12864=AXIS2_PLACEMENT_3D ( 'NONE', #4667, #1988, #11959 ) ;
#12869=VECTOR ( 'NONE', #9139, 1000.000000000000000 ) ;
#12871=PLANE ( 'NONE',  #10927 ) ;
#12875=ORIENTED_EDGE ( 'NONE', *, *, #9015, .F. ) ;
#12892=EDGE_CURVE ( 'NONE', #15120, #15422, #18092, .T. ) ;
#12897=CARTESIAN_POINT ( 'NONE',  ( 15.03925126672133494, -5.377732432866644707, -0.5657657256215723462 ) ) ;
#12904=DIRECTION ( 'NONE',  ( -1.000000000000000000, -2.586136946169074517E-16, 0.000000000000000000 ) ) ;
#12911=VERTEX_POINT ( 'NONE', #8043 ) ;
#12912=B_SPLINE_CURVE_WITH_KNOTS ( 'NONE', 3,
 ( #14782, #21794, #79, #29489, #17028, #19562, #534, #24442, #9740, #384, #10048, #2610, #10191, #17322, #19718, #22391, #29352, #26966, #12255 ),
 .UNSPECIFIED., .F., .F.,
 ( 4, 3, 3, 3, 3, 3, 4 ),
 ( -1.463115107851837610E-06, 0.000000000000000000, 2.244303852771090691E-05, 4.060544239443336439E-05, 5.609829020924229540E-05, 7.063629490958459251E-05, 8.524507318609981404E-05 ),
 .UNSPECIFIED. ) ;
#12914=EDGE_CURVE ( 'NONE', #9901, #8886, #12307, .T. ) ;
#12915=CYLINDRICAL_SURFACE ( 'NONE', #20583, 0.09999999999999982514 ) ;
#12920=EDGE_LOOP ( 'NONE', ( #26608, #8031, #28701, #6888, #12590 ) ) ;
#12925=CARTESIAN_POINT ( 'NONE',  ( 48.37818655883430807, -1.309616516426920230, -3.885368734293527471 ) ) ;
#12933=CYLINDRICAL_SURFACE ( 'NONE', #29673, 4.299999999999998046 ) ;
#12935=FACE_OUTER_BOUND ( 'NONE', #23936, .T. ) ;
#12938=AXIS2_PLACEMENT_3D ( 'NONE', #905, #15629, #12605 ) ;
#12939=DIRECTION ( 'NONE',  ( 0.000000000000000000, 0.000000000000000000, -1.000000000000000000 ) ) ;
#12948=VECTOR ( 'NONE', #15406, 1000.000000000000000 ) ;
#12950=CARTESIAN_POINT ( 'NONE',  ( 15.17214319754860696, 2.686240675664339328, 4.475885398016751004 ) ) ;
#12957=CARTESIAN_POINT ( 'NONE',  ( -36.11122220296831387, 0.3980941177579020440, 5.199999998461541928 ) ) ;
#12960=ORIENTED_EDGE ( 'NONE', *, *, #2278, .F. ) ;
#12961=LINE ( 'NONE', #29906, #19902 ) ;
#12966=CARTESIAN_POINT ( 'NONE',  ( 15.87128154250933321, -3.738196885377849998, -3.908481927057574801 ) ) ;
#12973=ORIENTED_EDGE ( 'NONE', *, *, #8251, .F. ) ;
#12981=EDGE_CURVE ( 'NONE', #3532, #2009, #27847, .T. ) ;
#12986=VECTOR ( 'NONE', #17702, 1000.000000000000000 ) ;
#12992=CARTESIAN_POINT ( 'NONE',  ( 15.95705409078464498, 0.6016956010317275894, 5.375730734456589666 ) ) ;
#12994=AXIS2_PLACEMENT_3D ( 'NONE', #21992, #5189, #29105 ) ;
#13005=FACE_OUTER_BOUND ( 'NONE', #22702, .T. ) ;
#13006=CARTESIAN_POINT ( 'NONE',  ( 58.45000000000001705, 0.7500000000000000000, 2.421260002560649660 ) ) ;
#13007=VECTOR ( 'NONE', #13856, 1000.000000000000000 ) ;
#13008=CARTESIAN_POINT ( 'NONE',  ( 15.76623786017565187, 3.265074799938528116, -4.311675893544650862 ) ) ;
#13011=ORIENTED_EDGE ( 'NONE', *, *, #21720, .T. ) ;
#13013=CARTESIAN_POINT ( 'NONE',  ( 47.01022879663531029, -4.154252208774217969, 1.054526470899727286 ) ) ;
#13020=ORIENTED_EDGE ( 'NONE', *, *, #529, .F. ) ;
#13023=VECTOR ( 'NONE', #28769, 1000.000000000000000 ) ;
#13024=EDGE_CURVE ( 'NONE', #1709, #8004, #26171, .T. ) ;
#13027=CARTESIAN_POINT ( 'NONE',  ( 56.95000000000001705, 0.6937162836135747357, -1.768873629894432975 ) ) ;
#13035=CARTESIAN_POINT ( 'NONE',  ( 56.99999999998442490, -0.7044205509462206916, 2.449516039469794570 ) ) ;
#13038=VECTOR ( 'NONE', #19910, 1000.000000000000000 ) ;
#13041=CARTESIAN_POINT ( 'NONE',  ( -54.44999999999997442, 0.000000000000000000, 2.168404344971008868E-14 ) ) ;
#13043=CARTESIAN_POINT ( 'NONE',  ( 58.45000000000001705, -0.8000000000000000444, 2.421260002560649660 ) ) ;
#13048=CARTESIAN_POINT ( 'NONE',  ( -54.49646078629579193, 1.531523113441620731, 3.320331042554034440 ) ) ;
#13059=EDGE_CURVE ( 'NONE', #27956, #30450, #12509, .T. ) ;
#13064=CARTESIAN_POINT ( 'NONE',  ( -54.44999999999997442, 5.694607616035192869E-16, -4.650000000000000355 ) ) ;
#13065=CARTESIAN_POINT ( 'NONE',  ( 15.03925126672127988, -4.804073783693435296, -2.042134687550375638 ) ) ;
#13068=DIRECTION ( 'NONE',  ( 0.000000000000000000, 0.000000000000000000, -1.000000000000000000 ) ) ;
#13075=DIRECTION ( 'NONE',  ( 0.000000000000000000, 0.000000000000000000, -1.000000000000000000 ) ) ;
#13078=CARTESIAN_POINT ( 'NONE',  ( -45.15971931043468146, 0.000000000000000000, 0.000000000000000000 ) ) ;
#13079=ADVANCED_FACE ( 'NONE', ( #27971 ), #3603, .T. ) ;
#13087=CARTESIAN_POINT ( 'NONE',  ( 57.00000000000001421, 0.000000000000000000, 0.000000000000000000 ) ) ;
#13092=FACE_OUTER_BOUND ( 'NONE', #16411, .T. ) ;
#13095=CARTESIAN_POINT ( 'NONE',  ( 57.00000000000001421, 0.000000000000000000, 0.000000000000000000 ) ) ;
#13096=EDGE_LOOP ( 'NONE', ( #14653, #7467, #12026, #19042 ) ) ;
#13098=CARTESIAN_POINT ( 'NONE',  ( -36.68133364217572989, 4.872718122832791821, -2.345308583460306462 ) ) ;
#13100=PRODUCT_DEFINITION_FORMATION_WITH_SPECIFIED_SOURCE ( 'ANY', '', #11370, .NOT_KNOWN. ) ;
#13102=CARTESIAN_POINT ( 'NONE',  ( -35.85663232820584057, -4.018128179617557194, 3.618665901676652918 ) ) ;
#13103=DIRECTION ( 'NONE',  ( 0.000000000000000000, 0.000000000000000000, -1.000000000000000000 ) ) ;
#13104=FACE_OUTER_BOUND ( 'NONE', #16614, .T. ) ;
#13107=ADVANCED_FACE ( 'NONE', ( #1380 ), #20867, .T. ) ;
#13108=CARTESIAN_POINT ( 'NONE',  ( 15.39414421509791353, 2.821511581828376247, 4.377605326016295706 ) ) ;
#13110=AXIS2_PLACEMENT_3D ( 'NONE', #11071, #3163, #22486 ) ;
#13113=ADVANCED_FACE ( 'NONE', ( #18018 ), #10578, .T. ) ;
#13117=ORIENTED_EDGE ( 'NONE', *, *, #7690, .T. ) ;
#13118=CIRCLE ( 'NONE', #2012, 0.4576450603546999840 ) ;
#13126=AXIS2_PLACEMENT_3D ( 'NONE', #6608, #25295, #6456 ) ;
#13132=DIRECTION ( 'NONE',  ( -1.000000000000000000, -1.786976680021908743E-16, 2.459562394685749209E-16 ) ) ;
#13137=ORIENTED_EDGE ( 'NONE', *, *, #12892, .T. ) ;
#13140=ADVANCED_FACE ( 'NONE', ( #29886 ), #8196, .T. ) ;
#13143=AXIS2_PLACEMENT_3D ( 'NONE', #2124, #19089, #7052 ) ;
#13144=CARTESIAN_POINT ( 'NONE',  ( 15.03925126672125856, -0.7747498368337712993, 5.363501452440941009 ) ) ;
#13150=DIRECTION ( 'NONE',  ( 2.586136946169074517E-16, -1.000000000000000000, 0.000000000000000000 ) ) ;
#13151=CARTESIAN_POINT ( 'NONE',  ( 57.00000000000001421, 0.000000000000000000, 1.949999999999999956 ) ) ;
#13153=ORIENTED_EDGE ( 'NONE', *, *, #8735, .F. ) ;
#13154=DIRECTION ( 'NONE',  ( 0.000000000000000000, 0.000000000000000000, -1.000000000000000000 ) ) ;
#13156=CARTESIAN_POINT ( 'NONE',  ( 15.48686146417446530, 2.966783028120432153, -4.272059443775269472 ) ) ;
#13158=DIRECTION ( 'NONE',  ( 0.000000000000000000, 0.000000000000000000, -1.000000000000000000 ) ) ;
#13159=ORIENTED_EDGE ( 'NONE', *, *, #18150, .T. ) ;
#13165=LINE ( 'NONE', #2044, #20374 ) ;
#13169=VECTOR ( 'NONE', #22793, 1000.000000000000000 ) ;
#13170=CARTESIAN_POINT ( 'NONE',  ( -35.85663232820584057, -1.793057972834465108, 4.026191436120613254 ) ) ;
#13181=CARTESIAN_POINT ( 'NONE',  ( 56.99976900444080030, -0.7668859551697654320, -1.738368808232523044 ) ) ;
#13186=CARTESIAN_POINT ( 'NONE',  ( 50.49731030164353029, -0.9327905306641465222, -3.995066436131524235 ) ) ;
#13189=ADVANCED_FACE ( 'NONE', ( #21496 ), #8798, .T. ) ;
#13190=CARTESIAN_POINT ( 'NONE',  ( -54.48167032960165557, 1.510995100284905579, -3.307167554963766243 ) ) ;
#13193=CARTESIAN_POINT ( 'NONE',  ( 50.37823977475586190, -1.183413901109533706, 3.885761703493072705 ) ) ;
#13194=CARTESIAN_POINT ( 'NONE',  ( -36.52757395963740095, -0.8926979523208378176, -5.334280177567952919 ) ) ;
#13196=ORIENTED_EDGE ( 'NONE', *, *, #25259, .T. ) ;
#13202=ORIENTED_EDGE ( 'NONE', *, *, #2200, .F. ) ;
#13205=VERTEX_POINT ( 'NONE', #28130 ) ;
#13211=DIRECTION ( 'NONE',  ( 0.000000000000000000, -8.881784197001252323E-16, -1.000000000000000000 ) ) ;
#13214=CARTESIAN_POINT ( 'NONE',  ( 15.03925126672132961, 0.000000000000000000, 5.200000000000000178 ) ) ;
#13216=CARTESIAN_POINT ( 'NONE',  ( 15.59055531549693541, 3.917775493694363398, 3.727542820438278337 ) ) ;
#13222=LINE ( 'NONE', #22906, #26696 ) ;
#13223=AXIS2_PLACEMENT_3D ( 'NONE', #24018, #7388, #31140 ) ;
#13225=CARTESIAN_POINT ( 'NONE',  ( 58.45000000000001705, 0.000000000000000000, 0.000000000000000000 ) ) ;
#13228=EDGE_LOOP ( 'NONE', ( #18220, #2113, #15091, #26735 ) ) ;
#13237=CARTESIAN_POINT ( 'NONE',  ( 57.02474788916244108, -0.7434350531339385393, -1.784201504348416067 ) ) ;
#13239=FACE_OUTER_BOUND ( 'NONE', #26029, .T. ) ;
#13241=CYLINDRICAL_SURFACE ( 'NONE', #4858, 1.000000000000000000 ) ;
#13242=VERTEX_POINT ( 'NONE', #6453 ) ;
#13246=FACE_OUTER_BOUND ( 'NONE', #31051, .T. ) ;
#13250=CARTESIAN_POINT ( 'NONE',  ( 15.86395258069111769, 2.563573972737327455, 4.761506352252367513 ) ) ;
#13252=DIRECTION ( 'NONE',  ( 0.000000000000000000, 0.000000000000000000, -1.000000000000000000 ) ) ;
#13257=EDGE_LOOP ( 'NONE', ( #29720, #4689, #17306, #22910 ) ) ;
#13258=DIRECTION ( 'NONE',  ( 0.000000000000000000, 0.000000000000000000, -1.000000000000000000 ) ) ;
#13270=CARTESIAN_POINT ( 'NONE',  ( -45.15971931043468146, -8.341470767433328331E-15, 0.000000000000000000 ) ) ;
#13273=DIRECTION ( 'NONE',  ( 1.000000000000000000, -0.000000000000000000, -0.000000000000000000 ) ) ;
#13274=EDGE_CURVE ( 'NONE', #30652, #18266, #26069, .T. ) ;
#13276=EDGE_CURVE ( 'NONE', #10683, #24584, #27183, .T. ) ;
#13277=ADVANCED_FACE ( 'NONE', ( #18650 ), #6755, .T. ) ;
#13282=CARTESIAN_POINT ( 'NONE',  ( 15.81621483022874131, -0.7811288459611355206, 5.350925378100964913 ) ) ;
#13284=LINE ( 'NONE', #3345, #1388 ) ;
#13291=VERTEX_POINT ( 'NONE', #11673 ) ;
#13292=CARTESIAN_POINT ( 'NONE',  ( 50.40918227724429101, -1.198378070452279509, -3.921585382224056282 ) ) ;
#13304=CARTESIAN_POINT ( 'NONE',  ( 46.90000000000001279, 1.734723475976807094E-15, 0.000000000000000000 ) ) ;
#13306=CARTESIAN_POINT ( 'NONE',  ( 47.00000000000002132, 2.428612866367529932E-14, 0.000000000000000000 ) ) ;
#13320=DIRECTION ( 'NONE',  ( -1.000000000000000000, -2.586136946169074517E-16, 0.000000000000000000 ) ) ;
#13322=DIRECTION ( 'NONE',  ( 0.000000000000000000, 0.000000000000000000, -1.000000000000000000 ) ) ;
#13326=CARTESIAN_POINT ( 'NONE',  ( 57.02131420290184138, 0.8120900198065377218, 2.469921935184963502 ) ) ;
#13327=CARTESIAN_POINT ( 'NONE',  ( 15.03925126672132961, -0.9159215771349653590, 4.311190327366007047 ) ) ;
#13329=ORIENTED_EDGE ( 'NONE', *, *, #83, .F. ) ;
#13330=CARTESIAN_POINT ( 'NONE',  ( 50.40000000000001279, -0.7711297561635979125, 3.938774833552910692 ) ) ;
#13342=ORIENTED_EDGE ( 'NONE', *, *, #4524, .F. ) ;
#13343=ORIENTED_EDGE ( 'NONE', *, *, #24307, .T. ) ;
#13350=( BOUNDED_CURVE ( )  B_SPLINE_CURVE ( 3, ( #7373, #1327, #3701, #25245 ),
 .UNSPECIFIED., .F., .T. ) 
 B_SPLINE_CURVE_WITH_KNOTS ( ( 4, 4 ),
 ( 0.000000000000000000, 1.570796326794896558 ),
 .UNSPECIFIED. ) 
 CURVE ( )  GEOMETRIC_REPRESENTATION_ITEM ( )  RATIONAL_B_SPLINE_CURVE ( ( 1.000000000000000000, 0.8047378541243649375, 0.8047378541243649375, 1.000000000000000000 ) ) 
 REPRESENTATION_ITEM ( '' )  );
#13351=DIRECTION ( 'NONE',  ( 0.000000000000000000, 0.000000000000000000, -1.000000000000000000 ) ) ;
#13354=EDGE_CURVE ( 'NONE', #23640, #1093, #14559, .T. ) ;
#13359=CARTESIAN_POINT ( 'NONE',  ( 58.45000000000001705, -0.8000000000000000444, -2.421260002560650104 ) ) ;
#13360=CARTESIAN_POINT ( 'NONE',  ( 16.08093158123429234, 2.941172302008990602, 4.539591111929677680 ) ) ;
#13366=DIRECTION ( 'NONE',  ( 0.000000000000000000, 0.000000000000000000, 1.000000000000000000 ) ) ;
#13370=AXIS2_PLACEMENT_3D ( 'NONE', #688, #3226, #27294 ) ;
#13374=EDGE_LOOP ( 'NONE', ( #26259, #3092, #4726, #9483 ) ) ;
#13384=CARTESIAN_POINT ( 'NONE',  ( 50.31907412294955861, 1.391939743175939048, 3.849999999996903899 ) ) ;
#13388=CARTESIAN_POINT ( 'NONE',  ( -36.39645873810162868, 4.962973169597041156, -2.162832296644261021 ) ) ;
#13391=CARTESIAN_POINT ( 'NONE',  ( -36.72207054450175434, -2.602043737612686591, 4.741394629686801920 ) ) ;
#13392=CARTESIAN_POINT ( 'NONE',  ( 57.05000000000001847, 0.7794871794871794934, 1.732743413496389717 ) ) ;
#13396=CIRCLE ( 'NONE', #11913, 2.549999999999999822 ) ;
#13402=DIRECTION ( 'NONE',  ( -1.000000000000000000, -0.000000000000000000, -0.000000000000000000 ) ) ;
#13407=ORIENTED_EDGE ( 'NONE', *, *, #31322, .F. ) ;
#13409=CARTESIAN_POINT ( 'NONE',  ( 48.29999997257028355, 0.7904052113207087338, 4.025738854575411807 ) ) ;
#13424=DIRECTION ( 'NONE',  ( 1.000000000000000000, -0.000000000000000000, -0.000000000000000000 ) ) ;
#13434=CARTESIAN_POINT ( 'NONE',  ( 47.04913391925882138, -4.173104349845818462, -1.013903299540405367 ) ) ;
#13445=CIRCLE ( 'NONE', #17526, 0.05000000000000143219 ) ;
#13448=ORIENTED_EDGE ( 'NONE', *, *, #21330, .T. ) ;
#13449=CIRCLE ( 'NONE', #23097, 2.549999999999999822 ) ;
#13453=ADVANCED_FACE ( 'NONE', ( #23178 ), #15404, .T. ) ;
#13454=CARTESIAN_POINT ( 'NONE',  ( 58.45000000000001705, 0.8000000000000000444, 3.499999999999999556 ) ) ;
#13457=CARTESIAN_POINT ( 'NONE',  ( 15.03925126672126211, -5.340403872473332925, 0.9205822173395827868 ) ) ;
#13480=ORIENTED_EDGE ( 'NONE', *, *, #5431, .F. ) ;
#13483=CIRCLE ( 'NONE', #3893, 0.04999999999999991257 ) ;
#13486=CARTESIAN_POINT ( 'NONE',  ( 48.50000000000002132, -1.391941090707485396, -3.750000000000022649 ) ) ;
#13489=DIRECTION ( 'NONE',  ( 1.000000000000000000, 0.000000000000000000, 0.000000000000000000 ) ) ;
#13491=DIRECTION ( 'NONE',  ( 1.000000000000000000, -0.000000000000000000, 0.000000000000000000 ) ) ;
#13497=CARTESIAN_POINT ( 'NONE',  ( 58.45000000000001705, -0.8000000000000000444, 2.421260002560650104 ) ) ;
#13500=CARTESIAN_POINT ( 'NONE',  ( 57.00000000000001421, 0.7263196003080392149, -2.437012689524181486 ) ) ;
#13501=ADVANCED_FACE ( 'NONE', ( #27439 ), #5752, .F. ) ;
#13503=ORIENTED_EDGE ( 'NONE', *, *, #20264, .T. ) ;
#13506=CARTESIAN_POINT ( 'NONE',  ( -36.40878371307407235, -0.9780988077348349297, -5.318542208600382182 ) ) ;
#13510=AXIS2_PLACEMENT_3D ( 'NONE', #2194, #28488, #16781 ) ;
#13515=VERTEX_POINT ( 'NONE', #6685 ) ;
#13517=DIRECTION ( 'NONE',  ( -1.000000000000000000, -0.000000000000000000, -0.000000000000000000 ) ) ;
#13525=ORIENTED_EDGE ( 'NONE', *, *, #24118, .F. ) ;
#13526=AXIS2_PLACEMENT_3D ( 'NONE', #17265, #12056, #5375 ) ;
#13529=CARTESIAN_POINT ( 'NONE',  ( 57.02131420290184138, -0.8120900198065377218, -2.469921935184963502 ) ) ;
#13531=EDGE_CURVE ( 'NONE', #1995, #4702, #9943, .T. ) ;
#13534=DIRECTION ( 'NONE',  ( 1.000000000000000000, 0.000000000000000000, 0.000000000000000000 ) ) ;
#13536=CARTESIAN_POINT ( 'NONE',  ( 57.00000000000001421, 0.6999999999999999556, -1.820027472320129736 ) ) ;
#13545=VERTEX_POINT ( 'NONE', #4149 ) ;
#13555=EDGE_LOOP ( 'NONE', ( #9220, #6607, #13159, #10587 ) ) ;
#13561=CARTESIAN_POINT ( 'NONE',  ( -54.49999999999997868, 2.818925648462311528E-15, 9.856100559121352825E-17 ) ) ;
#13566=LINE ( 'NONE', #20570, #17271 ) ;
#13568=CIRCLE ( 'NONE', #20679, 1.000000000000000000 ) ;
#13571=CARTESIAN_POINT ( 'NONE',  ( 15.17256654081422163, 3.426725948577415526, 3.937891352654330213 ) ) ;
#13575=CARTESIAN_POINT ( 'NONE',  ( 57.05000000000001847, -0.8000000000000000444, -2.421260002560649660 ) ) ;
#13576=VERTEX_POINT ( 'NONE', #2239 ) ;
#13581=CARTESIAN_POINT ( 'NONE',  ( 48.48122134030800368, 1.391940262981064214, 3.850000000000022293 ) ) ;
#13582=VERTEX_POINT ( 'NONE', #21426 ) ;
#13597=CARTESIAN_POINT ( 'NONE',  ( 47.00587335483849216, -4.148449925053760090, -1.066233527417929761 ) ) ;
#13606=AXIS2_PLACEMENT_3D ( 'NONE', #25443, #25597, #16267 ) ;
#13610=EDGE_CURVE ( 'NONE', #24812, #24817, #25527, .T. ) ;
#13612=DIRECTION ( 'NONE',  ( -1.000000000000000000, 0.000000000000000000, -0.000000000000000000 ) ) ;
#13616=VERTEX_POINT ( 'NONE', #25690 ) ;
#13619=VERTEX_POINT ( 'NONE', #28226 ) ;
#13624=CARTESIAN_POINT ( 'NONE',  ( 15.03925126672132961, 2.199885893005992799, -4.939696249117662141 ) ) ;
#13633=ORIENTED_EDGE ( 'NONE', *, *, #1080, .F. ) ;
#13634=DIRECTION ( 'NONE',  ( 0.000000000000000000, 0.000000000000000000, -1.000000000000000000 ) ) ;
#13641=CARTESIAN_POINT ( 'NONE',  ( 56.98113911906671092, -0.7884861235339004626, 2.477567088838556586 ) ) ;
#13646=CIRCLE ( 'NONE', #21280, 0.04999999999999991257 ) ;
#13650=CARTESIAN_POINT ( 'NONE',  ( -36.72207054450174724, -3.705258523861251430, -3.939862169952880411 ) ) ;
#13651=DIRECTION ( 'NONE',  ( 1.000000000000000000, -7.137062321707633821E-17, 7.924918191883221096E-17 ) ) ;
#13660=SURFACE_STYLE_FILL_AREA ( #16366 ) ;
#13663=CARTESIAN_POINT ( 'NONE',  ( 57.05000000000001847, -0.7500000000000000000, -1.778341924377873751 ) ) ;
#13670=( BOUNDED_SURFACE ( )  B_SPLINE_SURFACE ( 3, 2, ( 
 ( #19079, #14304, #31085 ),
 ( #11631, #9410, #21310 ),
 ( #9729, #4649, #18918 ),
 ( #26495, #23975, #16372 ),
 ( #11934, #4800, #21621 ),
 ( #31258, #19389, #14459 ),
 ( #4496, #9582, #7341 ),
 ( #28407, #26018, #21149 ),
 ( #14150, #23826, #4327 ),
 ( #13980, #23674, #30939 ),
 ( #28559, #27112, #29804 ),
 ( #17461, #24579, #29476 ),
 ( #21928, #10327, #5432 ),
 ( #371, #209, #19998 ),
 ( #15087, #17168, #24743 ),
 ( #520, #5738, #29640 ) ),
 .UNSPECIFIED., .F., .F., .F. ) 
 B_SPLINE_SURFACE_WITH_KNOTS ( ( 4, 2, 2, 2, 2, 2, 2, 4 ),
 ( 3, 3 ),
 ( 0.001780502285214185815, 0.002558945925323762027, 0.002753556835351156189, 0.002948167745378550350, 0.003337389565433338673, 0.003726611385488126996, 0.004115833205542915318, 0.004894276845652491097 ),
 ( 0.000000000000000000, 1.000000000000000000 ),
 .UNSPECIFIED. ) 
 GEOMETRIC_REPRESENTATION_ITEM ( )  RATIONAL_B_SPLINE_SURFACE ( (
 ( 1.000000000000000000, 0.9418517008537251600, 1.000000000000000000),
 ( 1.000000000000000000, 0.9417987965885094015, 1.000000000000000000),
 ( 1.000000000000000000, 0.9418198861734091709, 1.000000000000000000),
 ( 1.000000000000000000, 0.9434060303845579476, 1.000000000000000000),
 ( 1.000000000000000000, 0.9437939819948207854, 1.000000000000000000),
 ( 1.000000000000000000, 0.9445989566712774677, 1.000000000000000000),
 ( 1.000000000000000000, 0.9450169930049769906, 1.000000000000000000),
 ( 1.000000000000000000, 0.9461610507673769987, 1.000000000000000000),
 ( 1.000000000000000000, 0.9467217966427221576, 1.000000000000000000),
 ( 1.000000000000000000, 0.9467345476124371384, 1.000000000000000000),
 ( 1.000000000000000000, 0.9461964028052877174, 1.000000000000000000),
 ( 1.000000000000000000, 0.9446801822473928079, 1.000000000000000000),
 ( 1.000000000000000000, 0.9437582546536690264, 1.000000000000000000),
 ( 1.000000000000000000, 0.9418129560295395164, 1.000000000000000000),
 ( 1.000000000000000000, 0.9418016889777716116, 1.000000000000000000),
 ( 1.000000000000000000, 0.9418517008537247159, 1.000000000000000000) ) ) 
 REPRESENTATION_ITEM ( '' )  SURFACE ( )  );
#13675=LINE ( 'NONE', #28739, #26808 ) ;
#13678=EDGE_CURVE ( 'NONE', #25510, #16074, #11985, .T. ) ;
#13679=DIRECTION ( 'NONE',  ( 0.000000000000000000, 0.000000000000000000, 1.000000000000000000 ) ) ;
#13681=DIRECTION ( 'NONE',  ( -0.000000000000000000, -0.000000000000000000, 1.000000000000000000 ) ) ;
#13683=CIRCLE ( 'NONE', #18777, 0.4576450603546999840 ) ;
#13684=ADVANCED_FACE ( 'NONE', ( #30243 ), #19566, .T. ) ;
#13686=AXIS2_PLACEMENT_3D ( 'NONE', #2820, #17721, #29737 ) ;
#13687=CARTESIAN_POINT ( 'NONE',  ( 48.40000000000001990, 2.428612866367529932E-14, 4.000000000000022204 ) ) ;
#13689=CARTESIAN_POINT ( 'NONE',  ( -36.80043232705924083, -2.728070298465809618, 4.669343935538287305 ) ) ;
#13691=CARTESIAN_POINT ( 'NONE',  ( 51.90000000000001279, -4.227689052994015206, 1.125730994152045916 ) ) ;
#13698=DIRECTION ( 'NONE',  ( 1.000000000000000000, 2.586136946169074517E-16, -0.000000000000000000 ) ) ;
#13703=CARTESIAN_POINT ( 'NONE',  ( 36.50000000000002132, 0.7794871794871797155, 1.732743413496390161 ) ) ;
#13705=ADVANCED_FACE ( 'NONE', ( #10466 ), #27369, .T. ) ;
#13706=CARTESIAN_POINT ( 'NONE',  ( 15.03925126672132784, 5.086913985776164715, -1.171642053949048856 ) ) ;
#13717=CARTESIAN_POINT ( 'NONE',  ( -36.14504829323104218, -2.228024565339430385, 4.927420728799218885 ) ) ;
#13718=CARTESIAN_POINT ( 'NONE',  ( 56.95000000000001705, 0.6999999999999999556, -1.820027472320129736 ) ) ;
#13721=CARTESIAN_POINT ( 'NONE',  ( 15.22842924604237247, 3.779372845002901382, 3.883777290285411077 ) ) ;
#13726=CARTESIAN_POINT ( 'NONE',  ( -35.85663232820592583, -0.4576450603546987073, 5.200000000000000178 ) ) ;
#13728=EDGE_LOOP ( 'NONE', ( #17736, #16152, #13202, #4506 ) ) ;
#13732=CARTESIAN_POINT ( 'NONE',  ( 48.50000000000002132, 1.426739617975228525, 3.843750000000022649 ) ) ;
#13737=EDGE_CURVE ( 'NONE', #8353, #20985, #24171, .T. ) ;
#13742=ORIENTED_EDGE ( 'NONE', *, *, #26865, .F. ) ;
#13744=CARTESIAN_POINT ( 'NONE',  ( 47.00000000000002132, -4.131056160354152240, -1.100000000000000089 ) ) ;
#13750=CARTESIAN_POINT ( 'NONE',  ( 57.04171473382086077, -0.7493275531345221507, 1.778946371510476077 ) ) ;
#13753=CARTESIAN_POINT ( 'NONE',  ( -35.85663232820584057, -4.018128179617548312, -3.618665901676662244 ) ) ;
#13754=CARTESIAN_POINT ( 'NONE',  ( 57.00000000000001421, -0.7058179832143345322, -2.448718171069995009 ) ) ;
#13761=DIRECTION ( 'NONE',  ( 0.000000000000000000, 0.000000000000000000, -1.000000000000000000 ) ) ;
#13763=CIRCLE ( 'NONE', #2679, 0.4576450603546982632 ) ;
#13765=DIRECTION ( 'NONE',  ( 0.000000000000000000, 0.000000000000000000, -1.000000000000000000 ) ) ;
#13766=CARTESIAN_POINT ( 'NONE',  ( 15.76623786017565187, -5.175840503946257165, 1.569056257078743855 ) ) ;
#13768=ORIENTED_EDGE ( 'NONE', *, *, #8184, .F. ) ;
#13770=CARTESIAN_POINT ( 'NONE',  ( 50.40000000000001990, -0.6304760106459028624, 3.950000000000022826 ) ) ;
#13773=CARTESIAN_POINT ( 'NONE',  ( 47.00000000000002132, -3.726179070414207040, -1.041421356237309581 ) ) ;
#13782=ORIENTED_EDGE ( 'NONE', *, *, #25467, .F. ) ;
#13789=CARTESIAN_POINT ( 'NONE',  ( 57.05000000000001847, 0.7500000000000000000, 2.421260002560649660 ) ) ;
#13794=CARTESIAN_POINT ( 'NONE',  ( -54.49999999999997868, -4.179189514726507682, 0.8999999999999994671 ) ) ;
#13795=CARTESIAN_POINT ( 'NONE',  ( 15.22780280894161287, 5.340403875750862284, -0.9205822004573419592 ) ) ;
#13800=DIRECTION ( 'NONE',  ( 0.000000000000000000, 0.000000000000000000, 1.000000000000000000 ) ) ;
#13806=CARTESIAN_POINT ( 'NONE',  ( 51.70000000000001705, -4.259181259350203419, -1.000000000000000000 ) ) ;
#13808=ORIENTED_EDGE ( 'NONE', *, *, #18332, .F. ) ;
#13815=CARTESIAN_POINT ( 'NONE',  ( 56.95000000000001705, 0.000000000000000000, 1.949999999999999956 ) ) ;
#13820=ADVANCED_FACE ( 'NONE', ( #7131 ), #21944, .T. ) ;
#13823=CARTESIAN_POINT ( 'NONE',  ( 57.03253626007334987, -0.8141194241917997232, -2.469252834999610791 ) ) ;
#13828=CARTESIAN_POINT ( 'NONE',  ( -35.85663232820584057, 5.086913985776147840, -1.171642053949061513 ) ) ;
#13829=CARTESIAN_POINT ( 'NONE',  ( -36.39645873810207632, -2.743848709681594222, 4.666930520580660158 ) ) ;
#13833=CARTESIAN_POINT ( 'NONE',  ( 15.03925126672132784, 4.817150320980643663, 2.203324261490556157 ) ) ;
#13841=( BOUNDED_CURVE ( )  B_SPLINE_CURVE ( 3, ( #5283, #88, #19729, #12122 ),
 .UNSPECIFIED., .F., .T. ) 
 B_SPLINE_CURVE_WITH_KNOTS ( ( 4, 4 ),
 ( -8.881784197001252323E-16, 1.570796326794897446 ),
 .UNSPECIFIED. ) 
 CURVE ( )  GEOMETRIC_REPRESENTATION_ITEM ( )  RATIONAL_B_SPLINE_CURVE ( ( 1.000000000000000000, 0.8047378541243646044, 0.8047378541243646044, 1.000000000000000000 ) ) 
 REPRESENTATION_ITEM ( '' )  );
#13843=ADVANCED_FACE ( 'NONE', ( #15657 ), #1282, .T. ) ;
#13855=CARTESIAN_POINT ( 'NONE',  ( 50.50000002815836098, 0.7900353715961344614, 4.025797886239747214 ) ) ;
#13856=DIRECTION ( 'NONE',  ( -1.000000000000000000, -2.586136946169074517E-16, 0.000000000000000000 ) ) ;
#13857=ORIENTED_EDGE ( 'NONE', *, *, #2046, .F. ) ;
#13858=AXIS2_PLACEMENT_3D ( 'NONE', #7254, #28643, #17236 ) ;
#13859=CARTESIAN_POINT ( 'NONE',  ( 57.00000000000002132, -0.6820512820512792951, 1.773360101234991770 ) ) ;
#13867=EDGE_CURVE ( 'NONE', #30656, #16179, #25453, .T. ) ;
#13872=CIRCLE ( 'NONE', #17954, 0.05000000000000005829 ) ;
#13875=CARTESIAN_POINT ( 'NONE',  ( 44.98443556292537693, -3.726179070414207928, 1.000000000000002220 ) ) ;
#13877=CARTESIAN_POINT ( 'NONE',  ( -36.42771574642760868, 0.4841707035673717407, 5.391286593723181753 ) ) ;
#13881=EDGE_LOOP ( 'NONE', ( #27793, #8582, #5006, #17659 ) ) ;
#13884=CARTESIAN_POINT ( 'NONE',  ( 51.90000000000001279, -4.131056160354152240, 1.099999999999999867 ) ) ;
#13885=DIRECTION ( 'NONE',  ( 1.000000000000000000, 0.000000000000000000, 0.000000000000000000 ) ) ;
#13887=EDGE_CURVE ( 'NONE', #17048, #3273, #13952, .T. ) ;
#13889=EDGE_LOOP ( 'NONE', ( #15518, #27148, #5894, #18148 ) ) ;
#13894=VERTEX_POINT ( 'NONE', #1393 ) ;
#13899=AXIS2_PLACEMENT_3D ( 'NONE', #21917, #2883, #26942 ) ;
#13906=AXIS2_PLACEMENT_3D ( 'NONE', #10296, #27241, #26923 ) ;
#13907=CARTESIAN_POINT ( 'NONE',  ( -36.21152527658243514, 2.821511581828426429, -4.377605326016285936 ) ) ;
#13912=CARTESIAN_POINT ( 'NONE',  ( 57.03008957414009217, -0.7461961634598838211, -2.423767181580114727 ) ) ;
#13913=CARTESIAN_POINT ( 'NONE',  ( 56.95000000000001705, -0.6820512820512819596, -1.773360101234998210 ) ) ;
#13916=AXIS2_PLACEMENT_3D ( 'NONE', #30349, #27673, #28299 ) ;
#13919=DIRECTION ( 'NONE',  ( 0.000000000000000000, 1.224646799147353207E-16, 1.000000000000000000 ) ) ;
#13925=CARTESIAN_POINT ( 'NONE',  ( 57.00000000000001421, 0.000000000000000000, 2.549999999999999822 ) ) ;
#13926=CARTESIAN_POINT ( 'NONE',  ( 15.29384114148389884, -5.068511731019460065, 1.228278365482025070 ) ) ;
#13927=CIRCLE ( 'NONE', #1303, 0.05000000000000008604 ) ;
#13928=ORIENTED_EDGE ( 'NONE', *, *, #2681, .F. ) ;
#13930=CARTESIAN_POINT ( 'NONE',  ( -36.27260443516959754, -4.885888067249525513, 1.790336215468749215 ) ) ;
#13931=LINE ( 'NONE', #9214, #9306 ) ;
#13935=VECTOR ( 'NONE', #28875, 1000.000000000000000 ) ;
#13949=CARTESIAN_POINT ( 'NONE',  ( 54.50000000000002132, 1.734723475976807094E-15, 0.000000000000000000 ) ) ;
#13952=CIRCLE ( 'NONE', #16511, 0.05000000000000012768 ) ;
#13957=DIRECTION ( 'NONE',  ( 1.000000000000000000, 0.000000000000000000, 0.000000000000000000 ) ) ;
#13960=CARTESIAN_POINT ( 'NONE',  ( -35.85663232820584057, -2.199885893005943949, -4.939696249117691451 ) ) ;
#13962=CARTESIAN_POINT ( 'NONE',  ( 57.05000000000002558, 0.7500000000000000000, -2.490438859776669123 ) ) ;
#13966=CARTESIAN_POINT ( 'NONE',  ( 50.31877865969203611, -1.391940262980897236, 3.850000000000022293 ) ) ;
#13977=VERTEX_POINT ( 'NONE', #23559 ) ;
#13980=CARTESIAN_POINT ( 'NONE',  ( 16.10705563471229596, 5.191204783933242695, 1.522159526382794059 ) ) ;
#13985=SPHERICAL_SURFACE ( 'NONE', #28230, 0.05000000000000000278 ) ;
#13989=DIRECTION ( 'NONE',  ( 1.000000000000000000, 0.000000000000000000, 0.000000000000000000 ) ) ;
#13995=VERTEX_POINT ( 'NONE', #11054 ) ;
#14000=ADVANCED_FACE ( 'NONE', ( #28462 ), #18346, .T. ) ;
#14001=DIRECTION ( 'NONE',  ( 0.000000000000000000, 0.000000000000000000, -1.000000000000000000 ) ) ;
#14007=CARTESIAN_POINT ( 'NONE',  ( 46.90000000000001279, -4.227689052994015206, 1.125730994152046582 ) ) ;
#14010=VECTOR ( 'NONE', #30394, 1000.000000000000000 ) ;
#14011=ORIENTED_EDGE ( 'NONE', *, *, #7552, .F. ) ;
#14013=CARTESIAN_POINT ( 'NONE',  ( -44.49999999999999289, 1.499999999999999556, -4.029888335921975262 ) ) ;
#14021=FACE_OUTER_BOUND ( 'NONE', #29472, .T. ) ;
#14024=CARTESIAN_POINT ( 'NONE',  ( -37.18272003341174781, -1.653865106024005792E-14, 0.000000000000000000 ) ) ;
#14026=VERTEX_POINT ( 'NONE', #6153 ) ;
#14027=CARTESIAN_POINT ( 'NONE',  ( 50.33305158408655444, 1.365427245289844826, 3.854926352964885172 ) ) ;
#14035=CARTESIAN_POINT ( 'NONE',  ( -54.48167032960165557, -1.510995100284905579, -3.307167554963765799 ) ) ;
#14036=CARTESIAN_POINT ( 'NONE',  ( 36.55000000000001847, 2.326828918379971365E-16, 1.899999999999999911 ) ) ;
#14038=CARTESIAN_POINT ( 'NONE',  ( 51.89158610412761874, -1.677904505874998473E-13, 4.375000000000013323 ) ) ;
#14039=EDGE_CURVE ( 'NONE', #24537, #1564, #21508, .T. ) ;
#14041=EDGE_CURVE ( 'NONE', #31086, #1993, #19579, .T. ) ;
#14047=( BOUNDED_CURVE ( )  B_SPLINE_CURVE ( 3, ( #27894, #13773, #1140, #1285 ),
 .UNSPECIFIED., .F., .T. ) 
 B_SPLINE_CURVE_WITH_KNOTS ( ( 4, 4 ),
 ( 3.141592653589793116, 4.712388980384689674 ),
 .UNSPECIFIED. ) 
 CURVE ( )  GEOMETRIC_REPRESENTATION_ITEM ( )  RATIONAL_B_SPLINE_CURVE ( ( 1.000000000000000000, 0.8047378541243649375, 0.8047378541243649375, 1.000000000000000000 ) ) 
 REPRESENTATION_ITEM ( '' )  );
#14052=B_SPLINE_CURVE_WITH_KNOTS ( 'NONE', 3,
 ( #3878, #30464, #18460, #13823, #13529, #4344, #20989, #9270, #16386, #28422, #28575, #6887, #30624, #8936, #18775, #28097 ),
 .UNSPECIFIED., .F., .F.,
 ( 4, 3, 3, 3, 3, 4 ),
 ( 0.000000000000000000, 1.754151282668922588E-05, 5.222880005687533889E-05, 8.869434694929045231E-05, 0.0001259176481356621589, 0.0001632567749836554797 ),
 .UNSPECIFIED. ) ;
#14053=CARTESIAN_POINT ( 'NONE',  ( -36.80043232705879319, 0.5375162698823430230, 5.381098085087389293 ) ) ;
#14054=DIRECTION ( 'NONE',  ( 1.000000000000000000, 2.586136946169074517E-16, -0.000000000000000000 ) ) ;
#14056=ADVANCED_FACE ( 'NONE', ( #21680 ), #29652, .T. ) ;
#14057=CARTESIAN_POINT ( 'NONE',  ( 58.45000000000001705, -0.8000000000000000444, 2.421260002560649660 ) ) ;
#14058=ORIENTED_EDGE ( 'NONE', *, *, #3009, .F. ) ;
#14061=LINE ( 'NONE', #14216, #12619 ) ;
#14062=EDGE_LOOP ( 'NONE', ( #28452, #18594, #30750, #28951 ) ) ;
#14066=DIRECTION ( 'NONE',  ( -1.000000000000000000, 0.000000000000000000, 0.000000000000000000 ) ) ;
#14070=CARTESIAN_POINT ( 'NONE',  ( 46.90000000000001279, -4.227689052994015206, -1.125730994152046804 ) ) ;
#14071=ADVANCED_FACE ( 'NONE', ( #16903 ), #19558, .T. ) ;
#14072=VECTOR ( 'NONE', #18715, 1000.000000000000000 ) ;
#14075=CIRCLE ( 'NONE', #25192, 0.05000000000000014155 ) ;
#14076=DIRECTION ( 'NONE',  ( 1.000000000000000000, 0.000000000000000000, 0.000000000000000000 ) ) ;
#14081=CARTESIAN_POINT ( 'NONE',  ( -35.85663232820584767, 5.377732432866631385, -0.5657657256215208319 ) ) ;
#14082=B_SPLINE_CURVE_WITH_KNOTS ( 'NONE', 3,
 ( #23205, #1493, #213, #29034, #12247, #9731, #70, #7045, #7651, #28735, #19392, #19246, #9875, #373 ),
 .UNSPECIFIED., .F., .F.,
 ( 4, 2, 2, 2, 2, 2, 4 ),
 ( 0.000000000000000000, 2.506106230924558877E-05, 5.012212461849117754E-05, 0.0001002442492369727192, 0.0002004884984739364396, 0.0004009769969478670787, 0.0008019539938957288448 ),
 .UNSPECIFIED. ) ;
#14083=CARTESIAN_POINT ( 'NONE',  ( -35.85663232820592583, 3.426725943139576458, -3.937891353488712110 ) ) ;
#14084=EDGE_CURVE ( 'NONE', #24615, #1696, #21090, .T. ) ;
#14085=CARTESIAN_POINT ( 'NONE',  ( 48.43454905095371998, 1.397701019745849704, -3.854421226863028682 ) ) ;
#14088=CARTESIAN_POINT ( 'NONE',  ( 57.02007310689670305, -0.7405013978967619481, -2.427462356522636533 ) ) ;
#14090=CYLINDRICAL_SURFACE ( 'NONE', #29588, 0.1000000000000000472 ) ;
#14093=DIRECTION ( 'NONE',  ( -1.000000000000000000, -3.385297212316258532E-16, 2.459562394685744279E-16 ) ) ;
#14097=DIRECTION ( 'NONE',  ( 0.000000000000000000, -0.000000000000000000, 1.000000000000000000 ) ) ;
#14098=DIRECTION ( 'NONE',  ( 1.000000000000000000, 3.125586771759065906E-16, 0.000000000000000000 ) ) ;
#14099=CARTESIAN_POINT ( 'NONE',  ( -36.48821680285228553, 5.009497273852823618, 2.047744636826942521 ) ) ;
#14101=ORIENTED_EDGE ( 'NONE', *, *, #23820, .T. ) ;
#14104=DIRECTION ( 'NONE',  ( 0.9913331294122580406, -0.1313720918981620966, 1.608844118403764524E-17 ) ) ;
#14107=B_SPLINE_CURVE_WITH_KNOTS ( 'NONE', 3,
 ( #3457, #20402, #22452, #8040, #27352, #10720, #10408, #1210, #8193, #8506, #13237, #25288, #18186, #30191, #17861, #27498, #3741, #3600, #27199 ),
 .UNSPECIFIED., .F., .F.,
 ( 4, 3, 3, 3, 3, 3, 4 ),
 ( 0.000000000000000000, 1.884866041445846106E-05, 3.951905945590748818E-05, 5.784447894079529801E-05, 7.452120580692728668E-05, 7.659178893127488138E-05, 9.043917046408786540E-05 ),
 .UNSPECIFIED. ) ;
#14108=AXIS2_PLACEMENT_3D ( 'NONE', #23368, #4190, #14001 ) ;
#14127=CARTESIAN_POINT ( 'NONE',  ( -35.85663232820584057, -2.686240680702151717, -4.475885388010727439 ) ) ;
#14129=CARTESIAN_POINT ( 'NONE',  ( 48.40000000000001990, -1.391941090707485618, -3.850000000000022737 ) ) ;
#14131=CARTESIAN_POINT ( 'NONE',  ( -36.14504829323104929, -3.997758138077572632, -3.641634024966094341 ) ) ;
#14138=CARTESIAN_POINT ( 'NONE',  ( 50.37749466183669966, -1.328329461116575461, 3.879000873601222033 ) ) ;
#14143=AXIS2_PLACEMENT_3D ( 'NONE', #28707, #21590, #9558 ) ;
#14148=VERTEX_POINT ( 'NONE', #11833 ) ;
#14150=CARTESIAN_POINT ( 'NONE',  ( 16.10624235918716352, 5.092377074781523127, 1.825725187625140133 ) ) ;
#14156=ORIENTED_EDGE ( 'NONE', *, *, #20656, .T. ) ;
#14158=EDGE_CURVE ( 'NONE', #247, #8353, #24592, .T. ) ;
#14159=FACE_OUTER_BOUND ( 'NONE', #1224, .T. ) ;
#14167=CARTESIAN_POINT ( 'NONE',  ( 48.40000000000001990, 1.409787217987196861, 3.950000000000022826 ) ) ;
#14168=CARTESIAN_POINT ( 'NONE',  ( 56.95766603241608550, 0.7209790597604740503, 1.757928312873409116 ) ) ;
#14171=PLANE ( 'NONE',  #12864 ) ;
#14177=ORIENTED_EDGE ( 'NONE', *, *, #28931, .T. ) ;
#14180=FACE_OUTER_BOUND ( 'NONE', #12542, .T. ) ;
#14182=DIRECTION ( 'NONE',  ( 1.000000000000000000, 4.939082069373447378E-17, 1.520093157366847861E-16 ) ) ;
#14183=CARTESIAN_POINT ( 'NONE',  ( -36.30347965937239962, 3.148602930107292419, 4.139959549308673381 ) ) ;
#14185=DIRECTION ( 'NONE',  ( 1.000000000000000000, 0.000000000000000000, 0.000000000000000000 ) ) ;
#14190=CARTESIAN_POINT ( 'NONE',  ( -36.40793637698147478, 4.755763096844229487, 2.574151833883839835 ) ) ;
#14194=ADVANCED_FACE ( 'NONE', ( #898 ), #12601, .T. ) ;
#14195=CARTESIAN_POINT ( 'NONE',  ( 57.02075198358709684, 0.7405530952691583568, 1.786721332245943428 ) ) ;
#14196=AXIS2_PLACEMENT_3D ( 'NONE', #8126, #23595, #22536 ) ;
#14202=DIRECTION ( 'NONE',  ( -1.000000000000000000, 0.000000000000000000, 0.000000000000000000 ) ) ;
#14203=( BOUNDED_SURFACE ( )  B_SPLINE_SURFACE ( 3, 2, ( 
 ( #7236, #9304, #26541 ),
 ( #14516, #6761, #16899 ),
 ( #19433, #16421, #29079 ),
 ( #6932, #21503, #26075 ) ),
 .UNSPECIFIED., .F., .F., .F. ) 
 B_SPLINE_SURFACE_WITH_KNOTS ( ( 4, 4 ),
 ( 3, 3 ),
 ( 7.500129584393919939E-05, 0.0002378367988924469107 ),
 ( 0.000000000000000000, 1.000000000000000000 ),
 .UNSPECIFIED. ) 
 GEOMETRIC_REPRESENTATION_ITEM ( )  RATIONAL_B_SPLINE_SURFACE ( (
 ( 1.000000000000000000, 0.7071067811864996111, 1.000000000000000000),
 ( 1.000000000000000000, 0.7717803178830575650, 1.000000000000000000),
 ( 1.000000000000000000, 0.8407248428044677979, 1.000000000000000000),
 ( 1.000000000000000000, 0.8397191227596303431, 1.000000000000000000) ) ) 
 REPRESENTATION_ITEM ( '' )  SURFACE ( )  );
#14208=DIRECTION ( 'NONE',  ( 0.000000000000000000, 0.000000000000000000, -1.000000000000000000 ) ) ;
#14212=CARTESIAN_POINT ( 'NONE',  ( -54.49999999999997868, 1.549598385535858380, 4.064203588144675194 ) ) ;
#14213=ORIENTED_EDGE ( 'NONE', *, *, #502, .F. ) ;
#14214=CARTESIAN_POINT ( 'NONE',  ( 58.45000000000001705, 0.7500000000000000000, 2.489477856900920383 ) ) ;
#14216=CARTESIAN_POINT ( 'NONE',  ( 58.50000000000001421, 3.184081677783118191E-16, -2.600000000000000089 ) ) ;
#14218=EDGE_LOOP ( 'NONE', ( #11898, #3195, #8882, #22785 ) ) ;
#14220=EDGE_CURVE ( 'NONE', #29305, #17261, #22594, .T. ) ;
#14222=CARTESIAN_POINT ( 'NONE',  ( 56.95000000000001705, 3.184081677783118191E-16, -2.600000000000000089 ) ) ;
#14228=EDGE_CURVE ( 'NONE', #19303, #29056, #10450, .T. ) ;
#14229=CARTESIAN_POINT ( 'NONE',  ( -35.85663232820584057, 4.018128179617486140, 3.618665901676695995 ) ) ;
#14239=CARTESIAN_POINT ( 'NONE',  ( 15.86395258069112479, -3.736273719777164271, 3.909490113446820292 ) ) ;
#14248=VECTOR ( 'NONE', #13132, 1000.000000000000000 ) ;
#14258=CARTESIAN_POINT ( 'NONE',  ( -36.43290890416664496, 4.977698683490404008, 2.127480166903978454 ) ) ;
#14259=CARTESIAN_POINT ( 'NONE',  ( 16.07279755198632287, -5.235729994560235134, 1.359191621353775137 ) ) ;
#14260=ORIENTED_EDGE ( 'NONE', *, *, #29734, .T. ) ;
#14268=B_SPLINE_CURVE_WITH_KNOTS ( 'NONE', 3,
 ( #26728, #24193, #17221, #2499, #14354, #14819, #10088, #24480, #17360, #5020, #27007, #12444, #22135, #12154, #426, #29389 ),
 .UNSPECIFIED., .F., .F.,
 ( 4, 2, 2, 2, 2, 2, 2, 4 ),
 ( 1.738108305489988542E-18, 0.0004351083927046443789, 0.0008702167854092870232, 0.001740433570818579684, 0.002175541963523226503, 0.002610650356227873538, 0.003045758748932521007, 0.003480867141637168476 ),
 .UNSPECIFIED. ) ;
#14270=ADVANCED_FACE ( 'NONE', ( #19900 ), #8922, .T. ) ;
#14271=DIRECTION ( 'NONE',  ( 0.000000000000000000, 0.000000000000000000, 1.000000000000000000 ) ) ;
#14284=DIRECTION ( 'NONE',  ( 0.000000000000000000, -1.000000000000000000, 0.000000000000000000 ) ) ;
#14289=CARTESIAN_POINT ( 'NONE',  ( 57.00000000000001421, -0.6999999999999999556, 1.745709025009609228 ) ) ;
#14291=CARTESIAN_POINT ( 'NONE',  ( 57.00000000000001421, -0.7500000000000000000, 1.778341924377873751 ) ) ;
#14293=CARTESIAN_POINT ( 'NONE',  ( 50.34656340841117839, 1.329326705022644051, -3.861343257506216098 ) ) ;
#14294=CARTESIAN_POINT ( 'NONE',  ( 48.47161145301956253, -1.409900272549268641, 3.850000494969540554 ) ) ;
#14298=ORIENTED_EDGE ( 'NONE', *, *, #21900, .T. ) ;
#14304=CARTESIAN_POINT ( 'NONE',  ( 15.03925126672124968, 4.861582140531591989, 2.394243978978380927 ) ) ;
#14305=ORIENTED_EDGE ( 'NONE', *, *, #11006, .T. ) ;
#14308=ORIENTED_EDGE ( 'NONE', *, *, #25882, .T. ) ;
#14309=DIRECTION ( 'NONE',  ( 1.000000000000000000, 0.000000000000000000, 8.673617379883787770E-15 ) ) ;
#14313=ORIENTED_EDGE ( 'NONE', *, *, #15021, .T. ) ;
#14314=DIRECTION ( 'NONE',  ( 0.000000000000000000, 0.000000000000000000, -1.000000000000000000 ) ) ;
#14317=ORIENTED_EDGE ( 'NONE', *, *, #30124, .F. ) ;
#14319=CARTESIAN_POINT ( 'NONE',  ( 56.95000000000001705, 0.000000000000000000, 2.600000000000000089 ) ) ;
#14320=CARTESIAN_POINT ( 'NONE',  ( -36.38012252111054323, -2.292272662153026719, 4.901537128432083001 ) ) ;
#14328=ORIENTED_EDGE ( 'NONE', *, *, #20186, .T. ) ;
#14329=AXIS2_PLACEMENT_3D ( 'NONE', #13454, #30089, #3356 ) ;
#14337=EDGE_LOOP ( 'NONE', ( #16979, #3590, #25022, #17332, #6784 ) ) ;
#14338=ORIENTED_EDGE ( 'NONE', *, *, #16234, .T. ) ;
#14340=ORIENTED_EDGE ( 'NONE', *, *, #16759, .T. ) ;
#14341=EDGE_CURVE ( 'NONE', #1709, #28800, #25650, .T. ) ;
#14342=ORIENTED_EDGE ( 'NONE', *, *, #6394, .T. ) ;
#14343=CARTESIAN_POINT ( 'NONE',  ( -36.14504829323105639, 5.374753047227021518, 0.5963205376974505256 ) ) ;
#14348=FACE_OUTER_BOUND ( 'NONE', #25170, .T. ) ;
#14354=CARTESIAN_POINT ( 'NONE',  ( 15.70940947763171636, -5.349174094756193654, -0.7986533162261060248 ) ) ;
#14356=VERTEX_POINT ( 'NONE', #13828 ) ;
#14358=ORIENTED_EDGE ( 'NONE', *, *, #27476, .T. ) ;
#14363=DIRECTION ( 'NONE',  ( 1.000000000000000000, 0.000000000000000000, 0.000000000000000000 ) ) ;
#14368=CYLINDRICAL_SURFACE ( 'NONE', #3022, 0.05000000000000143219 ) ;
#14370=DIRECTION ( 'NONE',  ( -1.000000000000000000, -0.000000000000000000, -0.000000000000000000 ) ) ;
#14371=EDGE_CURVE ( 'NONE', #9408, #25588, #13445, .T. ) ;
#14377=AXIS2_PLACEMENT_3D ( 'NONE', #29485, #11385, #6646 ) ;
#14380=CARTESIAN_POINT ( 'NONE',  ( 16.10660252424457184, -3.410993390446848572, -4.205682099886866254 ) ) ;
#14382=CARTESIAN_POINT ( 'NONE',  ( 57.00000000000001421, 0.7500000000000000000, 2.421260002560649660 ) ) ;
#14386=AXIS2_PLACEMENT_3D ( 'NONE', #6226, #27447, #18423 ) ;
#14390=CARTESIAN_POINT ( 'NONE',  ( 15.41217651307625758, -3.272340825137230347, 4.050058705652139324 ) ) ;
#14392=VECTOR ( 'NONE', #24663, 1000.000000000000000 ) ;
#14396=AXIS2_PLACEMENT_3D ( 'NONE', #23629, #9545, #30747 ) ;
#14397=DIRECTION ( 'NONE',  ( 0.000000000000000000, -1.000000000000000000, -0.000000000000000000 ) ) ;
#14402=VERTEX_POINT ( 'NONE', #8486 ) ;
#14405=CARTESIAN_POINT ( 'NONE',  ( -54.49999999999997868, 1.734723475976807094E-15, 0.000000000000000000 ) ) ;
#14406=CARTESIAN_POINT ( 'NONE',  ( -35.85663232820579793, 5.377732432866620726, 0.5657657256216184205 ) ) ;
#14408=ORIENTED_EDGE ( 'NONE', *, *, #20049, .F. ) ;
#14410=ORIENTED_EDGE ( 'NONE', *, *, #21435, .F. ) ;
#14418=CARTESIAN_POINT ( 'NONE',  ( -36.43290890416663785, -4.977698683490452858, -2.127480166903659597 ) ) ;
#14423=CIRCLE ( 'NONE', #9376, 1.949999999999999956 ) ;
#14424=ORIENTED_EDGE ( 'NONE', *, *, #20359, .F. ) ;
#14435=CARTESIAN_POINT ( 'NONE',  ( 56.95000000000001705, -0.6999999999999998446, -1.820027472320129514 ) ) ;
#14436=CARTESIAN_POINT ( 'NONE',  ( -36.63359589171323449, -0.7811288459611956947, -5.350925378100957808 ) ) ;
#14438=EDGE_CURVE ( 'NONE', #28113, #26864, #6429, .T. ) ;
#14442=CARTESIAN_POINT ( 'NONE',  ( 54.50000000000002132, -0.003244837758069130020, -4.274998768541101057 ) ) ;
#14446=CARTESIAN_POINT ( 'NONE',  ( 48.34311953187607003, -1.211457450596347352, 3.917546004217186351 ) ) ;
#14447=CARTESIAN_POINT ( 'NONE',  ( 48.41852494697948828, -1.153996415704668044, -3.890257736381618869 ) ) ;
#14449=ORIENTED_EDGE ( 'NONE', *, *, #24023, .F. ) ;
#14459=CARTESIAN_POINT ( 'NONE',  ( 15.44259799936806132, 4.878092280899815059, 1.814329181850222072 ) ) ;
#14460=ORIENTED_EDGE ( 'NONE', *, *, #1528, .T. ) ;
#14464=ORIENTED_EDGE ( 'NONE', *, *, #1139, .F. ) ;
#14465=DIRECTION ( 'NONE',  ( 0.000000000000000000, 0.000000000000000000, 1.000000000000000000 ) ) ;
#14477=PLANE ( 'NONE',  #3625 ) ;
#14483=ADVANCED_FACE ( 'NONE', ( #26932 ), #7939, .T. ) ;
#14492=AXIS2_PLACEMENT_3D ( 'NONE', #10199, #10670, #5927 ) ;
#14496=CIRCLE ( 'NONE', #9965, 1.000000000000000000 ) ;
#14500=CARTESIAN_POINT ( 'NONE',  ( -36.04581030752770943, 2.525801262579482120, 4.794550356815209469 ) ) ;
#14503=DIRECTION ( 'NONE',  ( -1.000000000000000000, -0.000000000000000000, -0.000000000000000000 ) ) ;
#14507=CARTESIAN_POINT ( 'NONE',  ( 50.38719906715037666, 1.295960864328800088, 3.889961360030739002 ) ) ;
#14508=B_SPLINE_CURVE_WITH_KNOTS ( 'NONE', 3,
 ( #24755, #29488, #12558, #10189, #17180, #3065, #27128, #19858, #22543, #2913, #26826, #24299, #22389, #19716, #17801, #2753 ),
 .UNSPECIFIED., .F., .F.,
 ( 4, 3, 3, 3, 3, 4 ),
 ( 0.000000000000000000, 3.304654905548784445E-05, 6.654308848431610937E-05, 0.0001011328993923922879, 0.0001374176636839657517, 0.0001650454644847076165 ),
 .UNSPECIFIED. ) ;
#14516=CARTESIAN_POINT ( 'NONE',  ( 57.00000000000001421, 0.7256836306366275524, -1.800271087100996592 ) ) ;
#14520=CLOSED_SHELL ( 'NONE', ( #8665, #178, #12674, #23991, #10396, #26459, #21268, #17217, #23418, #21035, #11548, #5695, #15327, #3242, #17455, #29316, #11880, #10081, #7106, #15015, #20912, #11907, #28579, #1572, #24540, #23395, #14071, #5245, #28632, #26872, #29496, #22390, #23185, #22585, #21989, #883, #16914, #14857, #9531, #11795, #30666, #13501, #17670, #6516, #12190, #1447, #7652, #17766, #22412, #21817, #17744, #5864, #28415, #7814, #25450, #16898, #2893, #29777, #1592, #8803, #9197, #15256, #15109, #26677, #25842, #1973, #11427, #3393, #6911, #8056, #28341, #4510, #27140, #4078, #10130, #14483, #30746, #6863, #5172, #2283, #19329, #23247, #4895, #17209, #28562, #26209, #22451, #18344, #13079, #7157, #5732, #19104, #13453, #30399, #18315, #9920, #30283, #5145, #8317, #20106, #31096, #24298, #14056, #6088, #22108, #12503, #3618, #11771, #31275, #12821, #14555, #20860, #2487, #28006, #29095, #4870, #24742, #20426, #28856, #14270, #94, #1746, #29571, #29243, #30773, #188, #8037, #30777, #11049, #28757, #17166, #18742, #9769, #20715, #12319, #28194, #8451, #4953, #24147, #117, #18375, #8027, #15712, #15358, #10220, #30313, #22000, #20507, #25478, #13684, #11560, #15351, #1691, #15530, #2003, #4189, #252, #7759, #3179, #31229, #11398, #8242, #22004, #15013, #5, #4205, #27361, #5643, #731, #27472, #9866, #21505, #28387, #27196, #7302, #13189, #11197, #17375, #121, #13277, #21501, #10085, #12153, #27776, #18497, #13843, #11391, #22861, #6708, #22869, #6723, #4936, #13107, #27393, #13705, #7443, #13140, #29256, #18209, #14194, #20752, #4773, #28962, #11534, #13113, #29504, #393, #26642, #19752, #8354, #23639, #23462, #14000, #28466, #25829, #1664, #16784, #13820, #10764, #16730, #2552, #17281 ) ) ;
#14523=CARTESIAN_POINT ( 'NONE',  ( 56.95000000000001705, 0.000000000000000000, 0.000000000000000000 ) ) ;
#14525=CARTESIAN_POINT ( 'NONE',  ( 50.40000000000001279, 0.6304760106459517122, -3.950000000000022826 ) ) ;
#14533=CARTESIAN_POINT ( 'NONE',  ( -54.46926330052497178, 1.503605180550108944, 3.302415457191590242 ) ) ;
#14535=EDGE_LOOP ( 'NONE', ( #17935, #18762, #983, #8571 ) ) ;
#14536=DIRECTION ( 'NONE',  ( 0.000000000000000000, 0.000000000000000000, 1.000000000000000000 ) ) ;
#14539=CARTESIAN_POINT ( 'NONE',  ( 15.48686146417452569, -0.1108756495953492488, -5.200000001675014971 ) ) ;
#14544=TOROIDAL_SURFACE ( 'NONE', #8981, 2.549999999999999822, 0.05000000000000000278 ) ;
#14547=CYLINDRICAL_SURFACE ( 'NONE', #22141, 0.05000000000000143219 ) ;
#14548=CARTESIAN_POINT ( 'NONE',  ( -54.49853245345825314, -1.536420219664552667, -4.055116445457033869 ) ) ;
#14554=CARTESIAN_POINT ( 'NONE',  ( 15.70940947763171636, -3.858136107555796279, -3.790289750283466486 ) ) ;
#14555=ADVANCED_FACE ( 'NONE', ( #4518 ), #11996, .T. ) ;
#14556=DIRECTION ( 'NONE',  ( -1.000000000000000000, 0.000000000000000000, 0.000000000000000000 ) ) ;
#14559=CIRCLE ( 'NONE', #5975, 0.04999999999999991257 ) ;
#14568=DIRECTION ( 'NONE',  ( 1.000000000000000000, 2.586136946169074517E-16, -0.000000000000000000 ) ) ;
#14577=DIRECTION ( 'NONE',  ( 0.000000000000000000, 1.000000000000000000, 0.000000000000000000 ) ) ;
#14578=LINE ( 'NONE', #9990, #17111 ) ;
#14579=ORIENTED_EDGE ( 'NONE', *, *, #27266, .F. ) ;
#14585=DIRECTION ( 'NONE',  ( -1.000000000000000000, -4.678365685400793326E-16, 1.520093157366863638E-16 ) ) ;
#14586=B_SPLINE_CURVE_WITH_KNOTS ( 'NONE', 3,
 ( #19395, #24294, #24751, #14920, #24586, #12250, #24435, #15247, #19852, #3061, #14627, #10183, #7973, #29037, #3209, #216, #14777, #29198, #17466 ),
 .UNSPECIFIED., .F., .F.,
 ( 4, 3, 3, 3, 3, 3, 4 ),
 ( 7.925977934669585492E-22, 3.356391004153398916E-05, 6.712733219957284561E-05, 0.0001006985180134183105, 0.0001342867383218968741, 0.0001485301915999662963, 0.0001563009630072294926 ),
 .UNSPECIFIED. ) ;
#14588=CARTESIAN_POINT ( 'NONE',  ( -36.25997906085252964, -5.012895491272632675, -1.399447560527455003 ) ) ;
#14591=CARTESIAN_POINT ( 'NONE',  ( -44.49999999999999289, 1.499999999999999556, -4.029888335921975262 ) ) ;
#14594=EDGE_LOOP ( 'NONE', ( #10328, #22772, #7167, #28257 ) ) ;
#14603=CARTESIAN_POINT ( 'NONE',  ( -36.23324115033522475, 0.2667568399896946829, -5.200000000294884295 ) ) ;
#14605=CARTESIAN_POINT ( 'NONE',  ( 16.00221665700883733, -2.696520634775326108, 4.691964194339917071 ) ) ;
#14610=CARTESIAN_POINT ( 'NONE',  ( 48.42201677308601404, -1.327156576403696553, 3.879406274192464643 ) ) ;
#14614=CARTESIAN_POINT ( 'NONE',  ( -54.49999999999997868, 1.734723475976807094E-15, 0.000000000000000000 ) ) ;
#14619=ORIENTED_EDGE ( 'NONE', *, *, #21967, .T. ) ;
#14623=AXIS2_PLACEMENT_3D ( 'NONE', #22481, #778, #20128 ) ;
#14627=CARTESIAN_POINT ( 'NONE',  ( 54.49070678691090563, -0.001831363507947880720, 4.318560329337371329 ) ) ;
#14632=ORIENTED_EDGE ( 'NONE', *, *, #28082, .F. ) ;
#14639=CARTESIAN_POINT ( 'NONE',  ( 57.03907689491666844, -0.7490795634100378964, 2.421870079683545285 ) ) ;
#14650=ORIENTED_EDGE ( 'NONE', *, *, #23175, .F. ) ;
#14651=EDGE_CURVE ( 'NONE', #28473, #18214, #6189, .T. ) ;
#14652=ORIENTED_EDGE ( 'NONE', *, *, #8835, .F. ) ;
#14653=ORIENTED_EDGE ( 'NONE', *, *, #20025, .F. ) ;
#14654=DIRECTION ( 'NONE',  ( 0.000000000000000000, -1.000000000000000000, 0.000000000000000000 ) ) ;
#14657=DIRECTION ( 'NONE',  ( 0.000000000000000000, 0.000000000000000000, -1.000000000000000000 ) ) ;
#14671=AXIS2_PLACEMENT_3D ( 'NONE', #21956, #28912, #7223 ) ;
#14673=VECTOR ( 'NONE', #8763, 1000.000000000000000 ) ;
#14678=CARTESIAN_POINT ( 'NONE',  ( -36.04518387042615757, -3.779372851356037621, -3.883777284340919067 ) ) ;
#14682=CARTESIAN_POINT ( 'NONE',  ( 57.00000000000001421, -0.7263660278559024297, -2.436986164851962844 ) ) ;
#14686=ORIENTED_EDGE ( 'NONE', *, *, #9991, .F. ) ;
#14690=CARTESIAN_POINT ( 'NONE',  ( 15.81621483022863117, 0.7811288459611720469, -5.350925378100957808 ) ) ;
#14691=CARTESIAN_POINT ( 'NONE',  ( -36.80043232705877898, -4.951626736499100900, 2.174059107776701971 ) ) ;
#14695=CARTESIAN_POINT ( 'NONE',  ( 57.05000000000001847, 0.8000000000000000444, -1.778341924377873751 ) ) ;
#14700=ORIENTED_EDGE ( 'NONE', *, *, #24711, .T. ) ;
#14704=EDGE_CURVE ( 'NONE', #1571, #2659, #3402, .T. ) ;
#14705=CARTESIAN_POINT ( 'NONE',  ( 15.18459684427939926, -4.018128179617528772, -3.618665901676669350 ) ) ;
#14709=DIRECTION ( 'NONE',  ( -1.000000000000000000, 0.000000000000000000, -0.000000000000000000 ) ) ;
#14710=VERTEX_POINT ( 'NONE', #16158 ) ;
#14717=CARTESIAN_POINT ( 'NONE',  ( 58.45000000000001705, -0.8000000000000000444, -2.421260002560650104 ) ) ;
#14722=CARTESIAN_POINT ( 'NONE',  ( 58.50000000000001421, 0.8000000000000000444, 1.745709025009609228 ) ) ;
#14723=ORIENTED_EDGE ( 'NONE', *, *, #17724, .T. ) ;
#14724=EDGE_CURVE ( 'NONE', #30697, #1709, #21398, .T. ) ;
#14726=CARTESIAN_POINT ( 'NONE',  ( 15.98305126557417566, -2.728070298465786525, -4.669343935538291746 ) ) ;
#14731=DIRECTION ( 'NONE',  ( 0.000000000000000000, 0.000000000000000000, -1.000000000000000000 ) ) ;
#14735=ORIENTED_EDGE ( 'NONE', *, *, #1080, .T. ) ;
#14736=CARTESIAN_POINT ( 'NONE',  ( -36.21152527658242093, -5.035245099686886050, -1.330662535294857340 ) ) ;
#14738=EDGE_CURVE ( 'NONE', #2659, #30697, #13396, .T. ) ;
#14745=PRODUCT_DEFINITION ( 'UNKNOWN', '', #13100, #3156 ) ;
#14746=CARTESIAN_POINT ( 'NONE',  ( -54.49646078629579193, -1.531523113441621176, 3.320331042554033552 ) ) ;
#14747=CARTESIAN_POINT ( 'NONE',  ( 51.70000000000000995, -4.276948333784437395, -0.9210526315789474561 ) ) ;
#14751=CARTESIAN_POINT ( 'NONE',  ( -36.21152527658242093, -0.2904410314644593760, -5.200000000384610743 ) ) ;
#14754=CARTESIAN_POINT ( 'NONE',  ( 15.56401610563844962, 4.735424960531769756, -2.618558234549730024 ) ) ;
#14758=ORIENTED_EDGE ( 'NONE', *, *, #17185, .F. ) ;
#14762=DIRECTION ( 'NONE',  ( 0.000000000000000000, 0.000000000000000000, 1.000000000000000000 ) ) ;
#14772=ORIENTED_EDGE ( 'NONE', *, *, #6897, .F. ) ;
#14777=CARTESIAN_POINT ( 'NONE',  ( 54.49989931805382071, -0.003076767801038497469, 4.280178505497699071 ) ) ;
#14778=CARTESIAN_POINT ( 'NONE',  ( -44.49999999999999289, 2.818925648462311528E-15, 9.856100559121352825E-17 ) ) ;
#14782=CARTESIAN_POINT ( 'NONE',  ( -54.49999999999997868, -1.549999999999999600, 4.064480286580312907 ) ) ;
#14788=FACE_OUTER_BOUND ( 'NONE', #9581, .T. ) ;
#14800=CARTESIAN_POINT ( 'NONE',  ( -35.85663232820592583, 2.686240680702101979, 4.475885388010746979 ) ) ;
#14803=ORIENTED_EDGE ( 'NONE', *, *, #969, .F. ) ;
#14811=CARTESIAN_POINT ( 'NONE',  ( 15.81621483022852281, -4.847650360853460683, -2.396424556483019774 ) ) ;
#14813=EDGE_CURVE ( 'NONE', #28557, #26264, #18824, .T. ) ;
#14815=DIRECTION ( 'NONE',  ( -1.000000000000000000, 0.000000000000000000, -0.000000000000000000 ) ) ;
#14816=CARTESIAN_POINT ( 'NONE',  ( -36.38012252111054323, -3.953287617511738627, -3.694739123711016759 ) ) ;
#14819=CARTESIAN_POINT ( 'NONE',  ( 16.00221665700883733, -5.295593823078813323, -1.114646847977642130 ) ) ;
#14821=DIRECTION ( 'NONE',  ( -2.964772755551650383E-16, -0.9875000000000001554, -0.1576190026614809614 ) ) ;
#14826=CARTESIAN_POINT ( 'NONE',  ( -36.76447480099788123, -3.646691605040335737, -3.993181011920743373 ) ) ;
#14830=ORIENTED_EDGE ( 'NONE', *, *, #12146, .T. ) ;
#14831=CARTESIAN_POINT ( 'NONE',  ( 15.86395258069112124, 0.7247683022689473953, -5.358970532132275366 ) ) ;
#14832=CARTESIAN_POINT ( 'NONE',  ( 48.30260100412290569, 0.9326869175216770946, 3.995127421239667687 ) ) ;
#14833=CARTESIAN_POINT ( 'NONE',  ( 48.43326094847141405, -1.398826622412639775, -3.854114288381606190 ) ) ;
#14839=CARTESIAN_POINT ( 'NONE',  ( -54.48779575765000516, -1.517266520141196118, -4.041867453639657271 ) ) ;
#14840=DIRECTION ( 'NONE',  ( 0.000000000000000000, 0.000000000000000000, 1.000000000000000000 ) ) ;
#14845=CARTESIAN_POINT ( 'NONE',  ( 15.59140265158956495, -2.334862116274967647, -4.877703086529571408 ) ) ;
#14847=FACE_OUTER_BOUND ( 'NONE', #31259, .T. ) ;
#14850=EDGE_LOOP ( 'NONE', ( #376, #12208, #30015, #1759 ) ) ;
#14851=EDGE_CURVE ( 'NONE', #24741, #31043, #26894, .T. ) ;
#14852=CARTESIAN_POINT ( 'NONE',  ( 15.03925126672123014, -4.018128179617556306, 3.618665901676639596 ) ) ;
#14854=DIRECTION ( 'NONE',  ( 1.000000000000000000, -0.000000000000000000, -0.000000000000000000 ) ) ;
#14857=ADVANCED_FACE ( 'NONE', ( #5207 ), #19789, .F. ) ;
#14860=DIRECTION ( 'NONE',  ( -1.583552166641333955E-32, 1.224646799147353207E-16, 1.000000000000000000 ) ) ;
#14862=CARTESIAN_POINT ( 'NONE',  ( 47.00000000000002132, -3.826179070414207573, -1.100000000000000089 ) ) ;
#14866=CARTESIAN_POINT ( 'NONE',  ( 57.00319509709754584, 0.7184317838911207232, -2.441240553461111684 ) ) ;
#14868=CARTESIAN_POINT ( 'NONE',  ( 57.00000000000001421, -0.7500000000000000000, -1.778341924377873751 ) ) ;
#14871=EDGE_LOOP ( 'NONE', ( #16344, #14464, #29542 ) ) ;
#14876=CARTESIAN_POINT ( 'NONE',  ( 51.79029922165371858, -4.153760649298012808, 1.055564289358534413 ) ) ;
#14882=AXIS2_PLACEMENT_3D ( 'NONE', #21814, #5003, #103 ) ;
#14885=EDGE_CURVE ( 'NONE', #22540, #21420, #16990, .T. ) ;
#14890=CARTESIAN_POINT ( 'NONE',  ( 58.45000000000001705, 0.8000000000000000444, 3.499999999999999556 ) ) ;
#14893=DIRECTION ( 'NONE',  ( 0.000000000000000000, -0.3589743589743574215, -0.9333474217026310749 ) ) ;
#14894=CARTESIAN_POINT ( 'NONE',  ( -36.58361892165972762, -0.1071614981651333592, -5.407381887150175537 ) ) ;
#14896=CARTESIAN_POINT ( 'NONE',  ( -54.44999999999997442, -1.499999999999998668, 4.029888335921975262 ) ) ;
#14898=CARTESIAN_POINT ( 'NONE',  ( 54.49754940158101846, -0.002530889200248514093, -4.297001851131137862 ) ) ;
#14905=CARTESIAN_POINT ( 'NONE',  ( -44.49999999999999289, -1.500000000000000000, 3.300094695611020867 ) ) ;
#14908=EDGE_LOOP ( 'NONE', ( #2727, #30017, #18475, #30754 ) ) ;
#14913=EDGE_LOOP ( 'NONE', ( #11387, #11257, #14177, #23811 ) ) ;
#14914=ORIENTED_EDGE ( 'NONE', *, *, #6756, .T. ) ;
#14915=CARTESIAN_POINT ( 'NONE',  ( 57.05000000000001847, -0.7500000000000000000, -1.745709025009609228 ) ) ;
#14920=CARTESIAN_POINT ( 'NONE',  ( 54.43308742068420969, -0.0001827659103420331901, 4.369367483123359541 ) ) ;
#14921=VECTOR ( 'NONE', #19058, 1000.000000000000000 ) ;
#14923=ORIENTED_EDGE ( 'NONE', *, *, #22966, .F. ) ;
#14930=CARTESIAN_POINT ( 'NONE',  ( 57.05000000000001847, 0.8156862745098041323, -2.468735688885368873 ) ) ;
#14931=CARTESIAN_POINT ( 'NONE',  ( 57.00103033359725657, 0.7116617362530316404, 2.445288145576760552 ) ) ;
#14933=CIRCLE ( 'NONE', #25533, 1.000000000000000000 ) ;
#14934=CARTESIAN_POINT ( 'NONE',  ( -35.85663232820601820, -4.018128179617563411, 3.618665901676646257 ) ) ;
#14935=DIRECTION ( 'NONE',  ( 0.000000000000000000, 0.000000000000000000, -1.000000000000000000 ) ) ;
#14936=( BOUNDED_SURFACE ( )  B_SPLINE_SURFACE ( 3, 2, ( 
 ( #1118, #22830, #5236 ),
 ( #27546, #5872, #27247 ),
 ( #10767, #7626, #25187 ),
 ( #17285, #12522, #15533 ),
 ( #29452, #26928, #24551 ),
 ( #2871, #15361, #494 ),
 ( #25011, #12670, #22205 ),
 ( #22676, #5564, #29931 ),
 ( #3339, #8240, #10153 ),
 ( #15213, #19820, #24714 ) ),
 .UNSPECIFIED., .F., .F., .F. ) 
 B_SPLINE_SURFACE_WITH_KNOTS ( ( 4, 2, 2, 2, 4 ),
 ( 3, 3 ),
 ( 0.0004005301535625022482, 0.0008279283193725973976, 0.001041627402277645054, 0.001148476943730168936, 0.001255326485182692601 ),
 ( 0.000000000000000000, 1.000000000000000000 ),
 .UNSPECIFIED. ) 
 GEOMETRIC_REPRESENTATION_ITEM ( )  RATIONAL_B_SPLINE_SURFACE ( (
 ( 1.000000000000000000, 0.7071067811865260344, 1.000000000000000000),
 ( 1.000000000000000000, 0.7463463187144947497, 1.000000000000000000),
 ( 1.000000000000000000, 0.7946150999565809725, 1.000000000000000000),
 ( 1.000000000000000000, 0.8720431506958414847, 1.000000000000000000),
 ( 1.000000000000000000, 0.8987780092778684393, 1.000000000000000000),
 ( 1.000000000000000000, 0.9375340664365204857, 1.000000000000000000),
 ( 1.000000000000000000, 0.9504270566176279411, 1.000000000000000000),
 ( 1.000000000000000000, 0.9732249474031190450, 1.000000000000000000),
 ( 1.000000000000000000, 0.9839441327696822892, 1.000000000000000000),
 ( 1.000000000000000000, 0.9842509842514762797, 1.000000000000000000) ) ) 
 REPRESENTATION_ITEM ( '' )  SURFACE ( )  );
#14937=DIRECTION ( 'NONE',  ( -1.000000000000000000, -0.000000000000000000, -0.000000000000000000 ) ) ;
#14940=CARTESIAN_POINT ( 'NONE',  ( -54.49646078629579193, 1.531523113441620731, -3.320331042554034440 ) ) ;
#14947=LINE ( 'NONE', #699, #11351 ) ;
#14950=CARTESIAN_POINT ( 'NONE',  ( 50.50000000000002132, -0.6462379109120514054, -4.048750000000023164 ) ) ;
#14956=AXIS2_PLACEMENT_3D ( 'NONE', #17324, #24758, #10342 ) ;
#14964=EDGE_CURVE ( 'NONE', #22807, #1093, #13927, .T. ) ;
#14965=B_SPLINE_CURVE_WITH_KNOTS ( 'NONE', 3,
 ( #26427, #14705, #9664, #19320, #14554, #7266, #14380, #2986, #28955, #7430, #17103, #16932, #14845, #17387, #10113, #24365 ),
 .UNSPECIFIED., .F., .F.,
 ( 4, 2, 2, 2, 2, 2, 2, 4 ),
 ( 1.734723475976807094E-18, 0.0004351083927046438368, 0.0008702167854092859390, 0.001740433570818577733, 0.002175541963523223467, 0.002610650356227869635, 0.003045758748932515369, 0.003480867141637161537 ),
 .UNSPECIFIED. ) ;
#14973=CIRCLE ( 'NONE', #22564, 1.000000000000000000 ) ;
#14974=DIRECTION ( 'NONE',  ( 0.000000000000000000, 0.000000000000000000, -1.000000000000000000 ) ) ;
#14975=CARTESIAN_POINT ( 'NONE',  ( 50.33290990662629838, 1.365599538210783281, -3.854893000251051749 ) ) ;
#14978=FACE_OUTER_BOUND ( 'NONE', #11773, .T. ) ;
#14982=ORIENTED_EDGE ( 'NONE', *, *, #14228, .T. ) ;
#14984=CARTESIAN_POINT ( 'NONE',  ( -36.68866260399369850, -2.562020839648592396, -4.763023844701044673 ) ) ;
#14986=VERTEX_POINT ( 'NONE', #18037 ) ;
#14987=CARTESIAN_POINT ( 'NONE',  ( 50.33710128586459120, 1.426739617975221863, -3.843750000000023981 ) ) ;
#14989=VECTOR ( 'NONE', #17968, 1000.000000000000000 ) ;
#14990=CARTESIAN_POINT ( 'NONE',  ( 15.66436536804551416, 0.4008586329627058520, -5.396496690166812549 ) ) ;
#14997=LINE ( 'NONE', #7868, #14392 ) ;
#14999=DIRECTION ( 'NONE',  ( -0.000000000000000000, -0.9875000000000001554, 0.1576190026614806561 ) ) ;
#15012=AXIS2_PLACEMENT_3D ( 'NONE', #29046, #4666, #19404 ) ;
#15013=ADVANCED_FACE ( 'NONE', ( #15659 ), #25151, .F. ) ;
#15014=DIRECTION ( 'NONE',  ( 0.000000000000000000, 4.440892098500626951E-15, 1.000000000000000000 ) ) ;
#15015=ADVANCED_FACE ( 'NONE', ( #20269 ), #30212, .T. ) ;
#15016=CARTESIAN_POINT ( 'NONE',  ( 15.90468948301723628, -0.6818242347930719705, 5.365311767243448493 ) ) ;
#15018=CARTESIAN_POINT ( 'NONE',  ( 15.44259799936806488, 2.880023619481773434, 4.335093843541880432 ) ) ;
#15021=EDGE_CURVE ( 'NONE', #473, #3555, #24080, .T. ) ;
#15022=VECTOR ( 'NONE', #14054, 1000.000000000000000 ) ;
#15029=AXIS2_PLACEMENT_3D ( 'NONE', #19923, #17239, #19628 ) ;
#15031=AXIS2_PLACEMENT_3D ( 'NONE', #20701, #6267, #8323 ) ;
#15034=CARTESIAN_POINT ( 'NONE',  ( -35.85663232820584057, 3.426725943139506292, 3.937891353488775170 ) ) ;
#15037=CARTESIAN_POINT ( 'NONE',  ( 57.00000000000001421, 0.7500000000000000000, -2.421260002560649216 ) ) ;
#15042=LINE ( 'NONE', #27063, #11613 ) ;
#15048=CARTESIAN_POINT ( 'NONE',  ( -36.39645873810205501, -5.286410563980360244, -1.167394352644205213 ) ) ;
#15058=CARTESIAN_POINT ( 'NONE',  ( 50.50000000000002132, 0.6462379109120995890, 4.048750000000023164 ) ) ;
#15064=CARTESIAN_POINT ( 'NONE',  ( -36.80043232705879319, -0.5375162698823703344, -5.381098085087390182 ) ) ;
#15067=CARTESIAN_POINT ( 'NONE',  ( 16.08093158123429234, -3.408535483610572570, 4.200031884472242183 ) ) ;
#15068=CARTESIAN_POINT ( 'NONE',  ( 54.49508724208691746, -0.002176679993726876768, -4.307918145378301311 ) ) ;
#15072=DIRECTION ( 'NONE',  ( 1.000000000000000000, 0.000000000000000000, -0.000000000000000000 ) ) ;
#15073=CARTESIAN_POINT ( 'NONE',  ( -36.81959771849334828, -4.939398376933301194, -2.210903708596504202 ) ) ;
#15076=FACE_OUTER_BOUND ( 'NONE', #14337, .T. ) ;
#15080=CARTESIAN_POINT ( 'NONE',  ( 51.86029176559893017, 0.1231600413635689645, -4.365376941996956361 ) ) ;
#15081=EDGE_CURVE ( 'NONE', #18214, #9901, #14268, .T. ) ;
#15086=ORIENTED_EDGE ( 'NONE', *, *, #8014, .T. ) ;
#15087=CARTESIAN_POINT ( 'NONE',  ( 15.30042582489632608, 5.377732434016984975, 0.5657657146872882015 ) ) ;
#15089=DIRECTION ( 'NONE',  ( 0.000000000000000000, 0.000000000000000000, 1.000000000000000000 ) ) ;
#15091=ORIENTED_EDGE ( 'NONE', *, *, #14438, .F. ) ;
#15102=CARTESIAN_POINT ( 'NONE',  ( -36.58361892165971341, -3.091683853622008371, 4.437651790014588649 ) ) ;
#15104=CARTESIAN_POINT ( 'NONE',  ( 50.33625478868709990, -1.419210040599374612, -3.846553521706499001 ) ) ;
#15106=CARTESIAN_POINT ( 'NONE',  ( -54.44999999999997442, 1.549999999999999600, 4.029888335921975262 ) ) ;
#15108=ORIENTED_EDGE ( 'NONE', *, *, #29371, .T. ) ;
#15109=ADVANCED_FACE ( 'NONE', ( #14978 ), #29249, .F. ) ;
#15112=ORIENTED_EDGE ( 'NONE', *, *, #23377, .F. ) ;
#15120=VERTEX_POINT ( 'NONE', #21975 ) ;
#15128=CARTESIAN_POINT ( 'NONE',  ( 46.90000000000001279, 1.734723475976807094E-15, 0.000000000000000000 ) ) ;
#15133=CARTESIAN_POINT ( 'NONE',  ( 15.86395258069124559, -4.872718122832710996, -2.345308583460518292 ) ) ;
#15138=CARTESIAN_POINT ( 'NONE',  ( 48.48125827213483774, 1.426739617975217866, -3.843750000000022649 ) ) ;
#15145=ORIENTED_EDGE ( 'NONE', *, *, #14039, .F. ) ;
#15149=ORIENTED_EDGE ( 'NONE', *, *, #131, .T. ) ;
#15157=DIRECTION ( 'NONE',  ( 0.000000000000000000, 1.000000000000000000, 0.000000000000000000 ) ) ;
#15165=DIRECTION ( 'NONE',  ( 1.000000000000000000, 1.786976680021908743E-16, -2.459562394685749209E-16 ) ) ;
#15171=CIRCLE ( 'NONE', #22262, 1.000000000000000000 ) ;
#15178=CIRCLE ( 'NONE', #3040, 4.275000000000000355 ) ;
#15179=CARTESIAN_POINT ( 'NONE',  ( 15.67083574136752944, 3.495540671458142068, 4.131527132740846042 ) ) ;
#15181=DIRECTION ( 'NONE',  ( 0.000000000000000000, -5.942513678379226626E-16, -1.000000000000000000 ) ) ;
#15182=FACE_OUTER_BOUND ( 'NONE', #3588, .T. ) ;
#15186=CARTESIAN_POINT ( 'NONE',  ( 48.50000000000178346, 1.391941090720882235, -3.849999999997240074 ) ) ;
#15192=CARTESIAN_POINT ( 'NONE',  ( 50.45683212279338647, -1.211455355144520185, 3.917539841352834173 ) ) ;
#15193=CARTESIAN_POINT ( 'NONE',  ( 15.95705409078465209, -3.646557212684145899, -3.995389720703518055 ) ) ;
#15194=FACE_OUTER_BOUND ( 'NONE', #6531, .T. ) ;
#15196=ORIENTED_EDGE ( 'NONE', *, *, #22395, .T. ) ;
#15197=ORIENTED_EDGE ( 'NONE', *, *, #8062, .T. ) ;
#15202=CARTESIAN_POINT ( 'NONE',  ( 51.80000000000001847, -4.131056160354152240, 1.099999999999999867 ) ) ;
#15203=CARTESIAN_POINT ( 'NONE',  ( 50.36033030378882103, 1.282137971188145320, 3.869545987293864897 ) ) ;
#15204=LINE ( 'NONE', #10458, #14248 ) ;
#15210=AXIS2_PLACEMENT_3D ( 'NONE', #28176, #27582, #30533 ) ;
#15213=CARTESIAN_POINT ( 'NONE',  ( 48.50000000000002132, -1.391941090707492057, -3.850000000000022293 ) ) ;
#15214=CARTESIAN_POINT ( 'NONE',  ( 15.30042582489634384, 1.123735543663135550, 5.289358694936654004 ) ) ;
#15216=CARTESIAN_POINT ( 'NONE',  ( 51.72661555197463912, -4.179189466084497262, -0.9999999999999991118 ) ) ;
#15220=( BOUNDED_SURFACE ( )  B_SPLINE_SURFACE ( 3, 2, ( 
 ( #30650, #6916, #18482 ),
 ( #26226, #9290, #21343 ),
 ( #4369, #16105, #7075 ),
 ( #18953, #23236, #25586 ),
 ( #25754, #23709, #1999 ),
 ( #28599, #4060, #16581 ),
 ( #4532, #21489, #23536 ),
 ( #23385, #11509, #14183 ),
 ( #31122, #9454, #3904 ),
 ( #1668, #1524, #23858 ),
 ( #11185, #2151, #8963 ),
 ( #11327, #21013, #18642 ),
 ( #16257, #25904, #4209 ),
 ( #1836, #5150, #21661 ),
 ( #19740, #14500, #17054 ),
 ( #2628, #9618, #14800 ) ),
 .UNSPECIFIED., .F., .F., .F. ) 
 B_SPLINE_SURFACE_WITH_KNOTS ( ( 4, 2, 2, 2, 2, 2, 2, 4 ),
 ( 3, 3 ),
 ( 0.001780502285214235472, 0.002558945925323760293, 0.002753556835351141444, 0.002948167745378522595, 0.003337389565433285330, 0.003726611385488048066, 0.004115833205542810368, 0.004894276845652334972 ),
 ( 0.000000000000000000, 1.000000000000000000 ),
 .UNSPECIFIED. ) 
 GEOMETRIC_REPRESENTATION_ITEM ( )  RATIONAL_B_SPLINE_SURFACE ( (
 ( 1.000000000000000000, 0.9418517008537247159, 1.000000000000000000),
 ( 1.000000000000000000, 0.9417987965884988544, 1.000000000000000000),
 ( 1.000000000000000000, 0.9418198861734239369, 1.000000000000000000),
 ( 1.000000000000000000, 0.9434060303845547280, 1.000000000000000000),
 ( 1.000000000000000000, 0.9437939819948095721, 1.000000000000000000),
 ( 1.000000000000000000, 0.9445989566712877927, 1.000000000000000000),
 ( 1.000000000000000000, 0.9450169930049913125, 1.000000000000000000),
 ( 1.000000000000000000, 0.9461610507673479109, 1.000000000000000000),
 ( 1.000000000000000000, 0.9467217966425561793, 1.000000000000000000),
 ( 1.000000000000000000, 0.9467345476126033388, 1.000000000000000000),
 ( 1.000000000000000000, 0.9461964028053023723, 1.000000000000000000),
 ( 1.000000000000000000, 0.9446801822473783750, 1.000000000000000000),
 ( 1.000000000000000000, 0.9437582546536112948, 1.000000000000000000),
 ( 1.000000000000000000, 0.9418129560296572000, 1.000000000000000000),
 ( 1.000000000000000000, 0.9418016889776811285, 1.000000000000000000),
 ( 1.000000000000000000, 0.9418517008537240498, 1.000000000000000000) ) ) 
 REPRESENTATION_ITEM ( '' )  SURFACE ( )  );
#15221=CIRCLE ( 'NONE', #19297, 1.949999999999999956 ) ;
#15223=CARTESIAN_POINT ( 'NONE',  ( 48.41298237836545582, 1.088467210617599656, -3.899823238510140122 ) ) ;
#15224=CARTESIAN_POINT ( 'NONE',  ( 17.21035195517768557, -2.471857751707525626E-15, 0.000000000000000000 ) ) ;
#15228=CARTESIAN_POINT ( 'NONE',  ( 50.29999999999825633, -1.391941090720833607, -3.849999999997240074 ) ) ;
#15229=EDGE_CURVE ( 'NONE', #560, #4498, #24646, .T. ) ;
#15231=CARTESIAN_POINT ( 'NONE',  ( 15.39414421509792419, 3.291455042465473824, -4.036171416105450049 ) ) ;
#15240=ORIENTED_EDGE ( 'NONE', *, *, #27445, .F. ) ;
#15247=CARTESIAN_POINT ( 'NONE',  ( 54.47118315602192951, -0.0009370910484917797413, 4.346120462634435633 ) ) ;
#15249=LINE ( 'NONE', #5125, #26339 ) ;
#15251=EDGE_LOOP ( 'NONE', ( #20034, #25356, #24057, #31212 ) ) ;
#15256=ADVANCED_FACE ( 'NONE', ( #15771 ), #23697, .F. ) ;
#15260=DIRECTION ( 'NONE',  ( 0.000000000000000000, 0.000000000000000000, -1.000000000000000000 ) ) ;
#15266=ORIENTED_EDGE ( 'NONE', *, *, #5760, .T. ) ;
#15279=EDGE_LOOP ( 'NONE', ( #28983, #17778, #25879, #10277 ) ) ;
#15283=CARTESIAN_POINT ( 'NONE',  ( -44.49999999999999289, -1.499999999999999556, -3.300094695611020867 ) ) ;
#15286=CARTESIAN_POINT ( 'NONE',  ( 15.56274145962692401, -4.735538777079653983, -2.618062770413819518 ) ) ;
#15302=CARTESIAN_POINT ( 'NONE',  ( -36.11780688638066295, -2.199885882963843908, -4.939696253589922925 ) ) ;
#15304=EDGE_LOOP ( 'NONE', ( #22660, #15800, #6881, #17672 ) ) ;
#15309=CARTESIAN_POINT ( 'NONE',  ( -36.04581030752631676, -5.340403874104872273, 0.9205822090003401570 ) ) ;
#15312=ORIENTED_EDGE ( 'NONE', *, *, #6539, .F. ) ;
#15321=CARTESIAN_POINT ( 'NONE',  ( 56.96065904101961763, -0.7273651001630837554, 1.755300599839360265 ) ) ;
#15324=DIRECTION ( 'NONE',  ( -2.964772755551650383E-16, -0.9875000000000001554, 0.1576190026614809614 ) ) ;
#15325=CARTESIAN_POINT ( 'NONE',  ( 48.50000000000002132, -4.899999999999999467, 3.950000000000022826 ) ) ;
#15327=ADVANCED_FACE ( 'NONE', ( #9121 ), #10931, .T. ) ;
#15329=CARTESIAN_POINT ( 'NONE',  ( 15.57907767661756004, 2.743848709681572018, 4.666930520580628183 ) ) ;
#15334=CARTESIAN_POINT ( 'NONE',  ( 48.42155979508061137, 1.181909706220234613, -3.885998080850100234 ) ) ;
#15337=DIRECTION ( 'NONE',  ( 0.000000000000000000, 1.000000000000000000, 0.000000000000000000 ) ) ;
#15339=CARTESIAN_POINT ( 'NONE',  ( 50.36673905152862574, -1.398826622412641996, 3.854114288381605302 ) ) ;
#15340=VECTOR ( 'NONE', #29133, 1000.000000000000000 ) ;
#15350=CARTESIAN_POINT ( 'NONE',  ( 51.73054293450984886, -4.177413309949346676, 1.004109922956872625 ) ) ;
#15351=ADVANCED_FACE ( 'NONE', ( #18942 ), #28585, .T. ) ;
#15358=ADVANCED_FACE ( 'NONE', ( #11025 ), #1474, .T. ) ;
#15361=CARTESIAN_POINT ( 'NONE',  ( 48.41306782696076993, -1.296871156637267486, -3.889656364559859192 ) ) ;
#15362=AXIS2_PLACEMENT_3D ( 'NONE', #23379, #13698, #8332 ) ;
#15363=CARTESIAN_POINT ( 'NONE',  ( 15.76675455518219593, 0.1030603059132040172, 5.407440145940146436 ) ) ;
#15364=DIRECTION ( 'NONE',  ( 1.000000000000000000, 2.586136946169074517E-16, -0.000000000000000000 ) ) ;
#15373=ORIENTED_EDGE ( 'NONE', *, *, #31267, .T. ) ;
#15375=DIRECTION ( 'NONE',  ( -1.000000000000000000, -0.000000000000000000, -0.000000000000000000 ) ) ;
#15389=LINE ( 'NONE', #14915, #26033 ) ;
#15390=CARTESIAN_POINT ( 'NONE',  ( 46.90000000000001279, 1.734723475976807094E-15, 0.000000000000000000 ) ) ;
#15397=CARTESIAN_POINT ( 'NONE',  ( 57.00000000000001421, 0.7500000000000000000, -1.778341924377873751 ) ) ;
#15399=ORIENTED_EDGE ( 'NONE', *, *, #5976, .F. ) ;
#15404=CYLINDRICAL_SURFACE ( 'NONE', #23602, 0.04999999999999991257 ) ;
#15406=DIRECTION ( 'NONE',  ( 0.000000000000000000, 0.000000000000000000, -1.000000000000000000 ) ) ;
#15408=VECTOR ( 'NONE', #18285, 1000.000000000000000 ) ;
#15414=FACE_OUTER_BOUND ( 'NONE', #11106, .T. ) ;
#15422=VERTEX_POINT ( 'NONE', #29974 ) ;
#15427=ORIENTED_EDGE ( 'NONE', *, *, #8144, .F. ) ;
#15429=ORIENTED_EDGE ( 'NONE', *, *, #20376, .F. ) ;
#15430=CIRCLE ( 'NONE', #30082, 1.899999999999999911 ) ;
#15432=ORIENTED_EDGE ( 'NONE', *, *, #4292, .F. ) ;
#15441=( BOUNDED_SURFACE ( )  B_SPLINE_SURFACE ( 3, 2, ( 
 ( #8904, #13962, #4159 ),
 ( #23662, #9242, #26179 ),
 ( #13500, #1475, #20808 ),
 ( #30439, #16358, #18429 ) ),
 .UNSPECIFIED., .F., .F., .F. ) 
 B_SPLINE_SURFACE_WITH_KNOTS ( ( 4, 4 ),
 ( 3, 3 ),
 ( 6.470519842244164266E-05, 0.0002246728259156070709 ),
 ( 0.000000000000000000, 1.000000000000000000 ),
 .UNSPECIFIED. ) 
 GEOMETRIC_REPRESENTATION_ITEM ( )  RATIONAL_B_SPLINE_SURFACE ( (
 ( 1.000000000000000000, 0.5857791861290068125, 1.000000000000000000),
 ( 1.000000000000000000, 0.5849685391560944803, 1.000000000000000000),
 ( 1.000000000000000000, 0.6585504321673580908, 1.000000000000000000),
 ( 1.000000000000000000, 0.7071067811864985009, 1.000000000000000000) ) ) 
 REPRESENTATION_ITEM ( '' )  SURFACE ( )  );
#15442=CARTESIAN_POINT ( 'NONE',  ( 15.74652664997072549, -5.205077242910900459, -1.471673150993815682 ) ) ;
#15444=EDGE_CURVE ( 'NONE', #16322, #12204, #1420, .T. ) ;
#15447=EDGE_CURVE ( 'NONE', #3458, #10689, #18031, .T. ) ;
#15449=DIRECTION ( 'NONE',  ( 0.000000000000000000, 0.000000000000000000, 1.000000000000000000 ) ) ;
#15456=CARTESIAN_POINT ( 'NONE',  ( -36.52757395963740095, 0.8926979523208172784, 5.334280177567949366 ) ) ;
#15458=DIRECTION ( 'NONE',  ( 1.000000000000000000, -0.000000000000000000, -0.000000000000000000 ) ) ;
#15461=ORIENTED_EDGE ( 'NONE', *, *, #16851, .F. ) ;
#15462=DIRECTION ( 'NONE',  ( 0.000000000000000000, 0.000000000000000000, 1.000000000000000000 ) ) ;
#15463=ORIENTED_EDGE ( 'NONE', *, *, #10739, .F. ) ;
#15466=CARTESIAN_POINT ( 'NONE',  ( -35.85663232820597557, -5.340403872473347135, 0.9205822173395924457 ) ) ;
#15474=AXIS2_PLACEMENT_3D ( 'NONE', #19207, #23459, #14271 ) ;
#15477=CARTESIAN_POINT ( 'NONE',  ( -35.85663232820584057, 3.275050215668586784, -2.949461045527574932 ) ) ;
#15479=CARTESIAN_POINT ( 'NONE',  ( 48.30000000000001847, 2.428612866367529932E-14, 0.000000000000000000 ) ) ;
#15481=CARTESIAN_POINT ( 'NONE',  ( 50.30000000000001847, 1.391941090707534023, 3.850000000000022737 ) ) ;
#15482=CARTESIAN_POINT ( 'NONE',  ( 34.55000000000001847, 0.000000000000000000, 0.000000000000000000 ) ) ;
#15490=ORIENTED_EDGE ( 'NONE', *, *, #18636, .T. ) ;
#15492=CIRCLE ( 'NONE', #1334, 4.100000000000022737 ) ;
#15494=CARTESIAN_POINT ( 'NONE',  ( 15.30042582489635095, -2.199885882962415717, 4.939696253590554420 ) ) ;
#15497=AXIS2_PLACEMENT_3D ( 'NONE', #22716, #1011, #10663 ) ;
#15506=EDGE_LOOP ( 'NONE', ( #5620, #3087, #21615 ) ) ;
#15509=CARTESIAN_POINT ( 'NONE',  ( 15.76675455518197388, -3.261791109367189634, -4.314133646218568430 ) ) ;
#15513=ORIENTED_EDGE ( 'NONE', *, *, #3707, .F. ) ;
#15518=ORIENTED_EDGE ( 'NONE', *, *, #14041, .F. ) ;
#15523=DIRECTION ( 'NONE',  ( 0.000000000000000000, 0.000000000000000000, -1.000000000000000000 ) ) ;
#15530=ADVANCED_FACE ( 'NONE', ( #15414 ), #18528, .T. ) ;
#15531=AXIS2_PLACEMENT_3D ( 'NONE', #5728, #29949, #13158 ) ;
#15533=CARTESIAN_POINT ( 'NONE',  ( 48.33046193264123502, -1.143620537822785721, -3.937943076466140724 ) ) ;
#15543=CARTESIAN_POINT ( 'NONE',  ( -35.85663232820584057, 4.804073783693418420, 2.042134687550397398 ) ) ;
#15546=CARTESIAN_POINT ( 'NONE',  ( 50.33305158408655444, -1.365427245289796199, -3.854926352964885172 ) ) ;
#15547=CARTESIAN_POINT ( 'NONE',  ( -36.14490256869205353, 3.997744010329720599, -3.641645661657078037 ) ) ;
#15556=EDGE_CURVE ( 'NONE', #7731, #21976, #3864, .T. ) ;
#15561=ORIENTED_EDGE ( 'NONE', *, *, #7794, .F. ) ;
#15570=DIRECTION ( 'NONE',  ( 0.000000000000000000, -0.3137254901960767617, 0.9495137264943732669 ) ) ;
#15571=ORIENTED_EDGE ( 'NONE', *, *, #9432, .F. ) ;
#15582=AXIS2_PLACEMENT_3D ( 'NONE', #4127, #25971, #3809 ) ;
#15587=DIRECTION ( 'NONE',  ( 0.000000000000000000, -1.000000000000000000, 8.673617379884030739E-15 ) ) ;
#15591=CARTESIAN_POINT ( 'NONE',  ( 50.49738912176885464, -0.9335627837657783923, 3.994936164801344614 ) ) ;
#15593=VERTEX_POINT ( 'NONE', #29497 ) ;
#15601=ORIENTED_EDGE ( 'NONE', *, *, #304, .F. ) ;
#15602=VERTEX_POINT ( 'NONE', #15875 ) ;
#15610=( BOUNDED_SURFACE ( )  B_SPLINE_SURFACE ( 3, 2, ( 
 ( #6256, #8934, #20690 ),
 ( #22896, #8624, #25728 ),
 ( #18622, #28263, #6573 ),
 ( #17982, #20526, #27631 ),
 ( #1044, #1643, #27796 ),
 ( #23047, #30316, #27940 ) ),
 .UNSPECIFIED., .F., .F., .T. ) 
 B_SPLINE_SURFACE_WITH_KNOTS ( ( 4, 2, 4 ),
 ( 3, 3 ),
 ( 0.0001437848949530157389, 0.0003024153973479691408, 0.0004610458997429225697 ),
 ( 0.000000000000000000, 1.000000000000000000 ),
 .UNSPECIFIED. ) 
 GEOMETRIC_REPRESENTATION_ITEM ( )  RATIONAL_B_SPLINE_SURFACE ( (
 ( 1.000000000000000000, 0.7071067811865479058, 1.000000000000000000),
 ( 1.000000000000000000, 0.7306243023313020446, 1.000000000000000000),
 ( 1.000000000000000000, 0.7490085278695750581, 1.000000000000000000),
 ( 1.000000000000000000, 0.7725095633944483176, 1.000000000000000000),
 ( 1.000000000000000000, 0.7779630306549427665, 1.000000000000000000),
 ( 1.000000000000000000, 0.7779866052154988942, 1.000000000000000000) ) ) 
 REPRESENTATION_ITEM ( '' )  SURFACE ( )  );
#15620=CARTESIAN_POINT ( 'NONE',  ( 48.41300975153458097, 1.088846059295805135, 3.899771020632008423 ) ) ;
#15629=DIRECTION ( 'NONE',  ( 0.000000000000000000, -1.000000000000000000, 0.000000000000000000 ) ) ;
#15632=ORIENTED_EDGE ( 'NONE', *, *, #25197, .T. ) ;
#15644=ORIENTED_EDGE ( 'NONE', *, *, #3282, .T. ) ;
#15646=DIRECTION ( 'NONE',  ( 1.000000000000000000, 0.000000000000000000, 0.000000000000000000 ) ) ;
#15655=CYLINDRICAL_SURFACE ( 'NONE', #4771, 0.09999999999999982514 ) ;
#15656=VERTEX_POINT ( 'NONE', #25528 ) ;
#15657=FACE_OUTER_BOUND ( 'NONE', #30331, .T. ) ;
#15659=FACE_OUTER_BOUND ( 'NONE', #20891, .T. ) ;
#15666=CARTESIAN_POINT ( 'NONE',  ( 48.50000000000263611, 1.409901620923733390, -3.849999999997240518 ) ) ;
#15668=VECTOR ( 'NONE', #27660, 1000.000000000000000 ) ;
#15670=CYLINDRICAL_SURFACE ( 'NONE', #10281, 0.1000000000000002554 ) ;
#15671=VERTEX_POINT ( 'NONE', #4307 ) ;
#15673=CARTESIAN_POINT ( 'NONE',  ( 48.40000000000002700, 0.7711297561636268894, 3.938774833552663335 ) ) ;
#15683=CARTESIAN_POINT ( 'NONE',  ( -35.85663232820596846, -4.861582140531631069, -2.394243978978344956 ) ) ;
#15687=ORIENTED_EDGE ( 'NONE', *, *, #7552, .T. ) ;
#15691=CARTESIAN_POINT ( 'NONE',  ( 15.49676243306307732, -0.05686983728431626445, 5.199999998843000348 ) ) ;
#15692=EDGE_CURVE ( 'NONE', #28800, #24288, #23187, .T. ) ;
#15693=EDGE_CURVE ( 'NONE', #4483, #23272, #17022, .T. ) ;
#15712=ADVANCED_FACE ( 'NONE', ( #18897 ), #4709, .T. ) ;
#15713=VERTEX_POINT ( 'NONE', #29172 ) ;
#15715=ORIENTED_EDGE ( 'NONE', *, *, #19031, .T. ) ;
#15716=DIRECTION ( 'NONE',  ( 1.000000000000000000, -0.000000000000000000, -0.000000000000000000 ) ) ;
#15717=FACE_OUTER_BOUND ( 'NONE', #23499, .T. ) ;
#15718=EDGE_LOOP ( 'NONE', ( #10147, #513, #23201, #6593 ) ) ;
#15719=VECTOR ( 'NONE', #11562, 1000.000000000000000 ) ;
#15723=CARTESIAN_POINT ( 'NONE',  ( 57.01359174706111332, 0.7734660154240907692, -1.735448526467797459 ) ) ;
#15729=LINE ( 'NONE', #20344, #12948 ) ;
#15741=CARTESIAN_POINT ( 'NONE',  ( -36.92405921417685732, -0.1434351685890525030, -5.407416993630365099 ) ) ;
#15743=ORIENTED_EDGE ( 'NONE', *, *, #1559, .T. ) ;
#15747=DIRECTION ( 'NONE',  ( 1.000000000000000000, -0.000000000000000000, -0.000000000000000000 ) ) ;
#15763=DIRECTION ( 'NONE',  ( 0.000000000000000000, -1.000000000000000000, 0.000000000000000000 ) ) ;
#15767=CARTESIAN_POINT ( 'NONE',  ( 58.45000000000001705, 0.8000000000000002665, 2.421260002560650104 ) ) ;
#15771=FACE_OUTER_BOUND ( 'NONE', #558, .T. ) ;
#15774=DIRECTION ( 'NONE',  ( 0.000000000000000000, 0.000000000000000000, 1.000000000000000000 ) ) ;
#15775=ORIENTED_EDGE ( 'NONE', *, *, #31173, .F. ) ;
#15785=CARTESIAN_POINT ( 'NONE',  ( -35.85663232820584057, -3.426725943139567576, 3.937891353488737423 ) ) ;
#15795=EDGE_CURVE ( 'NONE', #1490, #24741, #4478, .T. ) ;
#15798=LINE ( 'NONE', #4850, #1584 ) ;
#15800=ORIENTED_EDGE ( 'NONE', *, *, #18713, .F. ) ;
#15807=CARTESIAN_POINT ( 'NONE',  ( 51.90000000000001279, -4.227689052994015206, 1.125730994152046582 ) ) ;
#15808=DIRECTION ( 'NONE',  ( 0.000000000000000000, -2.168404344971008128E-16, -1.000000000000000000 ) ) ;
#15815=CARTESIAN_POINT ( 'NONE',  ( -54.49999999999997868, 1.549999999999999600, 4.029888335921975262 ) ) ;
#15817=EDGE_LOOP ( 'NONE', ( #13196, #3706, #10576, #24429 ) ) ;
#15818=DIRECTION ( 'NONE',  ( 1.000000000000000000, 0.000000000000000000, 0.000000000000000000 ) ) ;
#15820=CARTESIAN_POINT ( 'NONE',  ( 58.45000000000001705, -0.8000000000000000444, 3.499999999999999556 ) ) ;
#15825=CARTESIAN_POINT ( 'NONE',  ( -35.85663232820601820, -4.683225679163349753, -2.703237727951245173 ) ) ;
#15827=EDGE_CURVE ( 'NONE', #4176, #28914, #3887, .T. ) ;
#15832=CYLINDRICAL_SURFACE ( 'NONE', #2014, 1.000000000000000000 ) ;
#15833=CARTESIAN_POINT ( 'NONE',  ( 15.29384114148388285, -0.3980941177579011003, 5.199999998461580120 ) ) ;
#15836=LINE ( 'NONE', #6501, #14010 ) ;
#15840=LINE ( 'NONE', #27878, #8888 ) ;
#15843=CARTESIAN_POINT ( 'NONE',  ( 54.40000000000001990, 0.000000000000000000, 0.000000000000000000 ) ) ;
#15844=CARTESIAN_POINT ( 'NONE',  ( -36.14504829323104218, 2.228024565339449481, -4.927420728799193128 ) ) ;
#15860=DIRECTION ( 'NONE',  ( 1.000000000000000000, 2.586136946169074517E-16, -0.000000000000000000 ) ) ;
#15863=CARTESIAN_POINT ( 'NONE',  ( 56.95641943120798345, 0.7163990203283279179, -1.759764883066090801 ) ) ;
#15865=ORIENTED_EDGE ( 'NONE', *, *, #20410, .F. ) ;
#15875=CARTESIAN_POINT ( 'NONE',  ( 47.10000000000002274, -4.276948333784438283, 0.9210526315789470120 ) ) ;
#15878=CARTESIAN_POINT ( 'NONE',  ( -54.49999999999997868, 0.000000000000000000, 0.000000000000000000 ) ) ;
#15881=ORIENTED_EDGE ( 'NONE', *, *, #22889, .F. ) ;
#15893=( BOUNDED_SURFACE ( )  B_SPLINE_SURFACE ( 3, 2, ( 
 ( #15186, #15666, #3623 ),
 ( #24837, #22945, #20585 ),
 ( #30219, #27373, #8526 ),
 ( #770, #18208, #12793 ),
 ( #22651, #20119, #5684 ),
 ( #15334, #24983, #9167 ),
 ( #18828, #6949, #15955 ),
 ( #4088, #20884, #11363 ),
 ( #23109, #9317, #1400 ),
 ( #6626, #6473, #25932 ) ),
 .UNSPECIFIED., .F., .F., .F. ) 
 B_SPLINE_SURFACE_WITH_KNOTS ( ( 4, 2, 2, 2, 4 ),
 ( 3, 3 ),
 ( 0.0002526260074104870901, 0.0003606909493797115550, 0.0004687558913489360741, 0.0006848857752873850581, 0.001117145543164283026 ),
 ( 0.000000000000000000, 1.000000000000000000 ),
 .UNSPECIFIED. ) 
 GEOMETRIC_REPRESENTATION_ITEM ( )  RATIONAL_B_SPLINE_SURFACE ( (
 ( 1.000000000000000000, 0.9842509842511785179, 1.000000000000000000),
 ( 1.000000000000000000, 0.9838268088398656186, 1.000000000000000000),
 ( 1.000000000000000000, 0.9731519947952637084, 1.000000000000000000),
 ( 1.000000000000000000, 0.9499473078865111608, 1.000000000000000000),
 ( 1.000000000000000000, 0.9371632344323043151, 1.000000000000000000),
 ( 1.000000000000000000, 0.8981767195496317413, 1.000000000000000000),
 ( 1.000000000000000000, 0.8714317066438567183, 1.000000000000000000),
 ( 1.000000000000000000, 0.7945716934681402721, 1.000000000000000000),
 ( 1.000000000000000000, 0.7462340517456830247, 1.000000000000000000),
 ( 1.000000000000000000, 0.7071067811865260344, 1.000000000000000000) ) ) 
 REPRESENTATION_ITEM ( '' )  SURFACE ( )  );
#15894=ORIENTED_EDGE ( 'NONE', *, *, #5431, .T. ) ;
#15905=CARTESIAN_POINT ( 'NONE',  ( 15.03925126672132961, 4.018128179617504792, 3.618665901676689778 ) ) ;
#15907=CARTESIAN_POINT ( 'NONE',  ( 48.46963600013424411, 1.366688880095624503, 3.854642372925540350 ) ) ;
#15908=TOROIDAL_SURFACE ( 'NONE', #24019, 4.275000000000000355, 0.1000000000000000056 ) ;
#15912=CARTESIAN_POINT ( 'NONE',  ( 46.90000000000001279, 1.734723475976807094E-15, 0.000000000000000000 ) ) ;
#15926=ORIENTED_EDGE ( 'NONE', *, *, #23161, .F. ) ;
#15933=FACE_BOUND ( 'NONE', #21957, .T. ) ;
#15936=FACE_OUTER_BOUND ( 'NONE', #27113, .T. ) ;
#15938=LINE ( 'NONE', #11196, #27287 ) ;
#15940=DIRECTION ( 'NONE',  ( -1.000000000000000000, -0.000000000000000000, -0.000000000000000000 ) ) ;
#15941=CARTESIAN_POINT ( 'NONE',  ( 57.02114944868134216, 0.7500000000000000000, 1.778342400449481442 ) ) ;
#15946=CARTESIAN_POINT ( 'NONE',  ( 15.56401610563799487, 3.953723660658996497, 3.694477770903627167 ) ) ;
#15947=AXIS2_PLACEMENT_3D ( 'NONE', #21472, #31107, #19101 ) ;
#15952=EDGE_CURVE ( 'NONE', #22807, #21791, #17610, .T. ) ;
#15953=LINE ( 'NONE', #23260, #24094 ) ;
#15955=CARTESIAN_POINT ( 'NONE',  ( 48.33019736648184050, 1.141995257496368987, -3.938405479918978713 ) ) ;
#15961=LINE ( 'NONE', #15815, #8579 ) ;
#15964=FACE_OUTER_BOUND ( 'NONE', #29193, .T. ) ;
#15967=CARTESIAN_POINT ( 'NONE',  ( 58.50000000000001421, -0.8000000000000000444, -1.778341924377873751 ) ) ;
#15968=CYLINDRICAL_SURFACE ( 'NONE', #18586, 0.05000000000000143219 ) ;
#15970=VERTEX_POINT ( 'NONE', #14896 ) ;
#15976=CIRCLE ( 'NONE', #2334, 4.375000000000000000 ) ;
#15979=AXIS2_PLACEMENT_3D ( 'NONE', #24447, #29357, #24760 ) ;
#15982=EDGE_CURVE ( 'NONE', #5897, #30927, #12529, .T. ) ;
#15985=CARTESIAN_POINT ( 'NONE',  ( -36.68866260399369139, 3.738196885377705225, -3.908481927057698257 ) ) ;
#15988=AXIS2_PLACEMENT_3D ( 'NONE', #3110, #12756, #20073 ) ;
#15990=AXIS2_PLACEMENT_3D ( 'NONE', #26331, #31066, #11762 ) ;
#15991=CARTESIAN_POINT ( 'NONE',  ( 58.45000000000001705, -0.7500000000000000000, 2.421260002560649660 ) ) ;
#15994=EDGE_CURVE ( 'NONE', #6668, #14986, #22106, .T. ) ;
#16003=FACE_OUTER_BOUND ( 'NONE', #20636, .T. ) ;
#16006=CARTESIAN_POINT ( 'NONE',  ( -35.85663232820584057, 0.000000000000000000, 5.200000000000000178 ) ) ;
#16009=CARTESIAN_POINT ( 'NONE',  ( 50.38147505302056572, -1.153996415704667156, 3.890257736381617537 ) ) ;
#16011=ORIENTED_EDGE ( 'NONE', *, *, #7264, .T. ) ;
#16015=ORIENTED_EDGE ( 'NONE', *, *, #1528, .F. ) ;
#16017=CIRCLE ( 'NONE', #3368, 10.00000000000000178 ) ;
#16022=DIRECTION ( 'NONE',  ( 0.000000000000000000, 1.000000000000000000, 0.000000000000000000 ) ) ;
#16026=CARTESIAN_POINT ( 'NONE',  ( 58.45000000000001705, -0.8000000000000002665, 2.421260002560650104 ) ) ;
#16034=CARTESIAN_POINT ( 'NONE',  ( 56.96751809705963154, -0.7713737938325972987, 2.482938273535672646 ) ) ;
#16035=LINE ( 'NONE', #16681, #4117 ) ;
#16036=CARTESIAN_POINT ( 'NONE',  ( 36.50000000000002132, 2.326828918379971365E-16, 1.899999999999999911 ) ) ;
#16055=CARTESIAN_POINT ( 'NONE',  ( -36.79682133506354091, -0.5584590966806997070, -5.380195666604552507 ) ) ;
#16056=AXIS2_PLACEMENT_3D ( 'NONE', #24357, #2669, #16775 ) ;
#16063=ORIENTED_EDGE ( 'NONE', *, *, #31135, .T. ) ;
#16073=DIRECTION ( 'NONE',  ( 0.000000000000000000, 0.000000000000000000, -1.000000000000000000 ) ) ;
#16074=VERTEX_POINT ( 'NONE', #18086 ) ;
#16077=AXIS2_PLACEMENT_3D ( 'NONE', #9823, #19490, #29138 ) ;
#16080=CARTESIAN_POINT ( 'NONE',  ( 15.71019289815287934, -0.8926979523208187217, 5.334280177567952919 ) ) ;
#16082=CARTESIAN_POINT ( 'NONE',  ( 58.45000000000001705, -0.8000000000000000444, 2.471260002560649927 ) ) ;
#16086=CARTESIAN_POINT ( 'NONE',  ( -36.76447480099788123, -2.670851142931307542, 4.702170608191340584 ) ) ;
#16090=CARTESIAN_POINT ( 'NONE',  ( 51.80000000000001137, -4.144729964592930749, 1.074323956811003011 ) ) ;
#16092=B_SPLINE_CURVE_WITH_KNOTS ( 'NONE', 3,
 ( #992, #24736, #12839, #12692, #1137, #6203, #8261, #29632, #17927, #7958, #13013, #18252, #10788, #22521, #25206, #8417 ),
 .UNSPECIFIED., .F., .F.,
 ( 4, 3, 3, 3, 3, 4 ),
 ( 0.000000000000000000, 3.304654905549463427E-05, 6.654308848431682766E-05, 0.0001011328993923933043, 0.0001374176636839670798, 0.0001650454644847091615 ),
 .UNSPECIFIED. ) ;
#16095=CARTESIAN_POINT ( 'NONE',  ( 48.40000000000001990, 0.6304760106459513791, -3.950000000000022826 ) ) ;
#16096=ORIENTED_EDGE ( 'NONE', *, *, #5681, .T. ) ;
#16105=CARTESIAN_POINT ( 'NONE',  ( -36.22818246778668794, 3.722599991951159648, 3.938370952810205772 ) ) ;
#16110=DIRECTION ( 'NONE',  ( -1.000000000000000000, 0.000000000000000000, 0.000000000000000000 ) ) ;
#16111=ORIENTED_EDGE ( 'NONE', *, *, #6365, .T. ) ;
#16116=CARTESIAN_POINT ( 'NONE',  ( -36.89250464418361020, 5.233646053067060322, -1.367284724151316189 ) ) ;
#16117=FACE_BOUND ( 'NONE', #11299, .T. ) ;
#16118=DIRECTION ( 'NONE',  ( 0.000000000000000000, 0.000000000000000000, 1.000000000000000000 ) ) ;
#16128=CARTESIAN_POINT ( 'NONE',  ( -54.44999999999997442, -1.499999999999999556, 4.029888335921975262 ) ) ;
#16129=CARTESIAN_POINT ( 'NONE',  ( -36.22955757456081471, 0.2668145608218083775, 5.199999998579032834 ) ) ;
#16133=EDGE_LOOP ( 'NONE', ( #19206, #26306, #11364, #3867 ) ) ;
#16147=DIRECTION ( 'NONE',  ( 0.000000000000000000, 0.000000000000000000, 1.000000000000000000 ) ) ;
#16150=CARTESIAN_POINT ( 'NONE',  ( -54.48779575765000516, 1.517266520141196118, -4.041867453639657271 ) ) ;
#16152=ORIENTED_EDGE ( 'NONE', *, *, #11089, .T. ) ;
#16153=CARTESIAN_POINT ( 'NONE',  ( 57.03469936322583322, -0.7478111487523275702, 1.780306085601951027 ) ) ;
#16158=CARTESIAN_POINT ( 'NONE',  ( 50.30000000000001847, 1.391941090707534023, -3.850000000000022737 ) ) ;
#16159=AXIS2_PLACEMENT_3D ( 'NONE', #2805, #15157, #22152 ) ;
#16162=DIRECTION ( 'NONE',  ( 1.000000000000000000, -0.000000000000000000, 0.000000000000000000 ) ) ;
#16170=DIRECTION ( 'NONE',  ( 1.000000000000000000, 0.000000000000000000, 0.000000000000000000 ) ) ;
#16172=CARTESIAN_POINT ( 'NONE',  ( -54.44999999999997442, -1.549999999999999600, -4.029888335921975262 ) ) ;
#16173=CARTESIAN_POINT ( 'NONE',  ( 15.98305126557428935, -5.283830060792393368, 1.151642405604310859 ) ) ;
#16176=CARTESIAN_POINT ( 'NONE',  ( -36.31414349454750834, -4.927920137446197835, 1.660974799722073403 ) ) ;
#16178=EDGE_CURVE ( 'NONE', #21494, #1093, #20692, .T. ) ;
#16179=VERTEX_POINT ( 'NONE', #2992 ) ;
#16186=TOROIDAL_SURFACE ( 'NONE', #11622, 4.000000000000022204, 0.1000000000000000056 ) ;
#16190=EDGE_CURVE ( 'NONE', #18491, #9980, #17478, .T. ) ;
#16206=CARTESIAN_POINT ( 'NONE',  ( 15.17214319754858209, 5.086913993735701744, -1.171642046065806131 ) ) ;
#16208=DIRECTION ( 'NONE',  ( 1.000000000000000000, -7.137062321647928144E-17, -7.924918191826694281E-17 ) ) ;
#16209=DIRECTION ( 'NONE',  ( -1.000000000000000000, -0.000000000000000000, -0.000000000000000000 ) ) ;
#16212=CARTESIAN_POINT ( 'NONE',  ( 50.41049980741060921, -0.7811435014051421044, 4.027217152858629134 ) ) ;
#16216=ORIENTED_EDGE ( 'NONE', *, *, #5826, .F. ) ;
#16218=LINE ( 'NONE', #13806, #22909 ) ;
#16222=CARTESIAN_POINT ( 'NONE',  ( 33.47623932017462778, 2.270506450603774156E-15, 4.375000000000000000 ) ) ;
#16226=EDGE_LOOP ( 'NONE', ( #4526, #9589, #674, #9833 ) ) ;
#16234=EDGE_CURVE ( 'NONE', #26742, #25704, #4662, .T. ) ;
#16241=CARTESIAN_POINT ( 'NONE',  ( 47.00000000000002132, 2.428612866367529932E-14, 0.000000000000000000 ) ) ;
#16249=CARTESIAN_POINT ( 'NONE',  ( -54.44999999999997442, 0.000000000000000000, 0.000000000000000000 ) ) ;
#16257=CARTESIAN_POINT ( 'NONE',  ( -36.68866260399460799, 2.562020839648815773, 4.763023844700911447 ) ) ;
#16267=DIRECTION ( 'NONE',  ( 6.938893903907228378E-15, -6.071532165918824830E-15, 1.000000000000000000 ) ) ;
#16271=CARTESIAN_POINT ( 'NONE',  ( -54.49865678108456279, -1.537045020190657807, -3.323865043138457320 ) ) ;
#16272=CIRCLE ( 'NONE', #24358, 0.05000000000000012768 ) ;
#16277=AXIS2_PLACEMENT_3D ( 'NONE', #26395, #21677, #23873 ) ;
#16281=B_SPLINE_CURVE_WITH_KNOTS ( 'NONE', 3,
 ( #13960, #23957, #16356, #31242, #4480, #21134, #9392, #11446, #11610, #30922, #13650, #9240, #26002, #14131, #4310, #9568 ),
 .UNSPECIFIED., .F., .F.,
 ( 4, 2, 2, 2, 2, 2, 2, 4 ),
 ( 0.000000000000000000, 0.0004351083927046470894, 0.0008702167854092941789, 0.001740433570818589008, 0.002175541963523235176, 0.002610650356227881344, 0.003045758748932527512, 0.003480867141637172812 ),
 .UNSPECIFIED. ) ;
#16288=CARTESIAN_POINT ( 'NONE',  ( -36.68866260399460799, -0.7269167730137759964, 5.359285300587722567 ) ) ;
#16290=ORIENTED_EDGE ( 'NONE', *, *, #16750, .F. ) ;
#16295=CARTESIAN_POINT ( 'NONE',  ( 48.39103590182073589, 1.199904535326282495, 3.921111011342365504 ) ) ;
#16296=CARTESIAN_POINT ( 'NONE',  ( 58.50000000000001421, 0.000000000000000000, 0.000000000000000000 ) ) ;
#16299=DIRECTION ( 'NONE',  ( -1.000000000000000000, -0.000000000000000000, -0.000000000000000000 ) ) ;
#16305=CARTESIAN_POINT ( 'NONE',  ( -36.72207054450174013, 3.705258523861193254, 3.939862169952904836 ) ) ;
#16310=AXIS2_PLACEMENT_3D ( 'NONE', #4051, #23374, #1655 ) ;
#16313=CARTESIAN_POINT ( 'NONE',  ( -36.04518387042614336, 2.525801254962709130, -4.794550361020548657 ) ) ;
#16316=CARTESIAN_POINT ( 'NONE',  ( 57.00303004862897183, -0.7171412854886025645, -2.441992855427530085 ) ) ;
#16320=DIRECTION ( 'NONE',  ( 0.000000000000000000, 0.000000000000000000, -1.000000000000000000 ) ) ;
#16322=VERTEX_POINT ( 'NONE', #23507 ) ;
#16326=CARTESIAN_POINT ( 'NONE',  ( -54.49999999999997868, -4.276948333784439171, 0.9210526315789471230 ) ) ;
#16327=CARTESIAN_POINT ( 'NONE',  ( -36.22955757456059445, 5.027944117023995574, 1.353132643598440987 ) ) ;
#16331=ORIENTED_EDGE ( 'NONE', *, *, #10667, .T. ) ;
#16332=CARTESIAN_POINT ( 'NONE',  ( -36.39645873810206211, -4.962973169597136192, 2.162832296644333852 ) ) ;
#16334=EDGE_LOOP ( 'NONE', ( #20179, #4012, #11576, #29559 ) ) ;
#16336=EDGE_LOOP ( 'NONE', ( #17046, #6446, #9013, #11328 ) ) ;
#16344=ORIENTED_EDGE ( 'NONE', *, *, #17072, .F. ) ;
#16349=AXIS2_PLACEMENT_3D ( 'NONE', #11766, #16209, #18593 ) ;
#16355=CARTESIAN_POINT ( 'NONE',  ( 58.50000000000001421, 0.8000000000000000444, 2.421260002560649660 ) ) ;
#16356=CARTESIAN_POINT ( 'NONE',  ( -36.14490256869206775, -2.228039998204413230, -4.927410888447854020 ) ) ;
#16357=CARTESIAN_POINT ( 'NONE',  ( 56.95000000000001705, 0.7137254901960785602, 2.500119182087999548 ) ) ;
#16358=CARTESIAN_POINT ( 'NONE',  ( 57.00000000000001421, 0.7137254901960804476, -2.500119182088006209 ) ) ;
#16360=ORIENTED_EDGE ( 'NONE', *, *, #29057, .F. ) ;
#16363=EDGE_CURVE ( 'NONE', #28473, #28315, #25058, .T. ) ;
#16365=ORIENTED_EDGE ( 'NONE', *, *, #8715, .F. ) ;
#16366=FILL_AREA_STYLE ('',( #4017 ) ) ;
#16372=CARTESIAN_POINT ( 'NONE',  ( 15.39414421509791175, 4.855742670514265669, 1.883114206442366489 ) ) ;
#16384=CARTESIAN_POINT ( 'NONE',  ( 47.00000000000002132, 1.426739617975221641, -3.843750000000023093 ) ) ;
#16386=CARTESIAN_POINT ( 'NONE',  ( 56.98109951608436319, -0.7885528131279547770, -2.477553856021609491 ) ) ;
#16387=ORIENTED_EDGE ( 'NONE', *, *, #16178, .T. ) ;
#16389=DIRECTION ( 'NONE',  ( 0.000000000000000000, 0.000000000000000000, 1.000000000000000000 ) ) ;
#16390=EDGE_CURVE ( 'NONE', #7615, #15970, #12912, .T. ) ;
#16392=CARTESIAN_POINT ( 'NONE',  ( 57.03052440771394060, 0.7462437932013319397, -1.781707539322121336 ) ) ;
#16396=CARTESIAN_POINT ( 'NONE',  ( 51.80000000000001847, -3.726179070414207928, -1.000000000000002220 ) ) ;
#16397=CARTESIAN_POINT ( 'NONE',  ( 51.80000000000001847, 2.428612866367529932E-14, 0.000000000000000000 ) ) ;
#16400=VECTOR ( 'NONE', #14208, 1000.000000000000000 ) ;
#16402=ORIENTED_EDGE ( 'NONE', *, *, #22563, .F. ) ;
#16409=ORIENTED_EDGE ( 'NONE', *, *, #25886, .F. ) ;
#16411=EDGE_LOOP ( 'NONE', ( #14340, #3859, #10170, #4463, #19812, #29299, #10398, #1181, #2895, #7013 ) ) ;
#16412=DIRECTION ( 'NONE',  ( 0.000000000000000000, 0.000000000000000000, 1.000000000000000000 ) ) ;
#16415=ORIENTED_EDGE ( 'NONE', *, *, #28770, .F. ) ;
#16421=CARTESIAN_POINT ( 'NONE',  ( 57.01079215475500206, 0.7500001437588036390, -1.746008375800299772 ) ) ;
#16426=CARTESIAN_POINT ( 'NONE',  ( -54.49999999999997868, 1.549999999999999600, 3.332135201338624952 ) ) ;
#16427=AXIS2_PLACEMENT_3D ( 'NONE', #2757, #20022, #12717 ) ;
#16434=CARTESIAN_POINT ( 'NONE',  ( -36.58361892165972762, 0.1071614981651403398, 5.407381887150175537 ) ) ;
#16443=DIRECTION ( 'NONE',  ( -1.000000000000000000, -0.000000000000000000, -0.000000000000000000 ) ) ;
#16448=CARTESIAN_POINT ( 'NONE',  ( 34.50000000000001421, 3.918869757271530460E-16, 3.200000000000000178 ) ) ;
#16457=CARTESIAN_POINT ( 'NONE',  ( -54.45981523601835761, 1.500740478982482973, -4.030402907299741599 ) ) ;
#16463=CARTESIAN_POINT ( 'NONE',  ( -36.22909104983231998, 3.722832355337073018, -3.938244298534259169 ) ) ;
#16464=DIRECTION ( 'NONE',  ( 1.000000000000000000, 2.586136946169074517E-16, -0.000000000000000000 ) ) ;
#16468=CARTESIAN_POINT ( 'NONE',  ( 50.30000000000001847, 1.409787217987196861, 3.850000000000022737 ) ) ;
#16472=DIRECTION ( 'NONE',  ( 0.000000000000000000, -1.000000000000000000, 0.000000000000000000 ) ) ;
#16474=EDGE_CURVE ( 'NONE', #24391, #29070, #792, .T. ) ;
#16481=CARTESIAN_POINT ( 'NONE',  ( -36.39645873810229659, 5.286410563980371791, 1.167394352644176569 ) ) ;
#16484=ORIENTED_EDGE ( 'NONE', *, *, #2856, .T. ) ;
#16485=ORIENTED_EDGE ( 'NONE', *, *, #1139, .T. ) ;
#16486=CARTESIAN_POINT ( 'NONE',  ( -36.63359589171323449, -4.847650360853545948, 2.396424556482879442 ) ) ;
#16487=DIRECTION ( 'NONE',  ( 1.000000000000000000, 1.786976680021873984E-16, 2.459562394685737870E-16 ) ) ;
#16488=CIRCLE ( 'NONE', #23066, 0.1000000000000002554 ) ;
#16497=EDGE_CURVE ( 'NONE', #8913, #25822, #23540, .T. ) ;
#16498=AXIS2_PLACEMENT_3D ( 'NONE', #9113, #13534, #23513 ) ;
#16506=CARTESIAN_POINT ( 'NONE',  ( 56.98981708175836758, -0.7951539052630037796, 2.475425269917271187 ) ) ;
#16507=DIRECTION ( 'NONE',  ( -1.000000000000000000, 0.000000000000000000, -0.000000000000000000 ) ) ;
#16511=AXIS2_PLACEMENT_3D ( 'NONE', #6617, #21036, #23404 ) ;
#16514=CARTESIAN_POINT ( 'NONE',  ( -36.81959771849335539, 5.295593823078808882, -1.114646847977579069 ) ) ;
#16517=CARTESIAN_POINT ( 'NONE',  ( -37.18272003341174781, -1.653865106024005792E-14, 0.000000000000000000 ) ) ;
#16518=DIRECTION ( 'NONE',  ( 0.000000000000000000, -1.000000000000000000, 0.000000000000000000 ) ) ;
#16521=LINE ( 'NONE', #23191, #6341 ) ;
#16525=CARTESIAN_POINT ( 'NONE',  ( 48.39081772275599747, -1.198378070452209121, 3.921585382223973681 ) ) ;
#16531=AXIS2_PLACEMENT_3D ( 'NONE', #3653, #10481, #8101 ) ;
#16536=ORIENTED_EDGE ( 'NONE', *, *, #23367, .T. ) ;
#16543=EDGE_CURVE ( 'NONE', #6673, #20943, #6727, .T. ) ;
#16545=VERTEX_POINT ( 'NONE', #31103 ) ;
#16562=CIRCLE ( 'NONE', #15531, 1.000000000000000000 ) ;
#16564=CARTESIAN_POINT ( 'NONE',  ( -36.04518387042615046, -2.525801254963603526, 4.794550361020572637 ) ) ;
#16570=DIRECTION ( 'NONE',  ( -1.000000000000000000, -0.000000000000000000, -0.000000000000000000 ) ) ;
#16581=CARTESIAN_POINT ( 'NONE',  ( -36.25997906085253675, 3.232943006030361666, 4.078682900256771937 ) ) ;
#16592=CARTESIAN_POINT ( 'NONE',  ( 50.49731436448253419, 0.9333771270347341886, 3.994943142064453667 ) ) ;
#16594=VERTEX_POINT ( 'NONE', #16082 ) ;
#16598=CARTESIAN_POINT ( 'NONE',  ( -54.49646078629579193, -1.531523113441620731, -3.320331042554033552 ) ) ;
#16601=DIRECTION ( 'NONE',  ( 1.000000000000000000, -0.000000000000000000, 0.000000000000000000 ) ) ;
#16603=FACE_OUTER_BOUND ( 'NONE', #7749, .T. ) ;
#16604=CIRCLE ( 'NONE', #28741, 0.05000000000000012768 ) ;
#16609=ORIENTED_EDGE ( 'NONE', *, *, #17593, .T. ) ;
#16614=EDGE_LOOP ( 'NONE', ( #12652, #17460, #17416, #27017 ) ) ;
#16615=B_SPLINE_CURVE_WITH_KNOTS ( 'NONE', 3,
 ( #11837, #31151, #28786, #4864, #7100, #16761, #2338, #19298, #28933, #24195, #2500, #15456, #22907, #3267, #22763, #3438 ),
 .UNSPECIFIED., .F., .F.,
 ( 4, 2, 2, 2, 2, 2, 2, 4 ),
 ( 0.000000000000000000, 0.0004351083927046413432, 0.0008702167854092826864, 0.001740433570818565373, 0.002175541963523206553, 0.002610650356227847951, 0.003045758748932489348, 0.003480867141637130745 ),
 .UNSPECIFIED. ) ;
#16616=CARTESIAN_POINT ( 'NONE',  ( -54.47710365256552478, 1.507983431629474014, 4.035431478432993657 ) ) ;
#16617=ORIENTED_EDGE ( 'NONE', *, *, #12156, .F. ) ;
#16618=LINE ( 'NONE', #14214, #28382 ) ;
#16620=CARTESIAN_POINT ( 'NONE',  ( 51.70000000000001705, -3.726179070414207928, 1.000000000000000444 ) ) ;
#16621=ORIENTED_EDGE ( 'NONE', *, *, #21381, .F. ) ;
#16629=CARTESIAN_POINT ( 'NONE',  ( 15.97944027357901398, 3.614202567156016954, -4.024415706308015928 ) ) ;
#16636=DIRECTION ( 'NONE',  ( 0.000000000000000000, 0.000000000000000000, -1.000000000000000000 ) ) ;
#16644=CARTESIAN_POINT ( 'NONE',  ( -36.92362342067259107, 3.046685255238509971, -4.470266847516099595 ) ) ;
#16645=CARTESIAN_POINT ( 'NONE',  ( 48.40115653635459125, 0.8930148142854623661, 3.925689827643446428 ) ) ;
#16647=DIRECTION ( 'NONE',  ( 0.000000000000000000, 3.552713678800500929E-15, 1.000000000000000000 ) ) ;
#16648=FACE_OUTER_BOUND ( 'NONE', #2394, .T. ) ;
#16649=CARTESIAN_POINT ( 'NONE',  ( -35.85663232820584767, 5.377732432866621615, 0.5657657256216177544 ) ) ;
#16658=FACE_OUTER_BOUND ( 'NONE', #1127, .T. ) ;
#16659=CARTESIAN_POINT ( 'NONE',  ( -36.31440869660546156, 4.928592478219054662, 1.658905555082685668 ) ) ;
#16660=CARTESIAN_POINT ( 'NONE',  ( 15.41170998834821226, -4.895911367890834143, 2.323639554370769300 ) ) ;
#16664=ORIENTED_EDGE ( 'NONE', *, *, #19942, .F. ) ;
#16667=CIRCLE ( 'NONE', #25752, 2.600000000000000089 ) ;
#16668=ORIENTED_EDGE ( 'NONE', *, *, #12914, .T. ) ;
#16670=ORIENTED_EDGE ( 'NONE', *, *, #2634, .F. ) ;
#16674=EDGE_LOOP ( 'NONE', ( #5914, #11003, #20547, #6169 ) ) ;
#16681=CARTESIAN_POINT ( 'NONE',  ( -44.49999999999999289, 1.499999999999999556, 4.029888335921975262 ) ) ;
#16687=FACE_OUTER_BOUND ( 'NONE', #7949, .T. ) ;
#16693=CARTESIAN_POINT ( 'NONE',  ( 48.43920370478603843, -1.278211010209444387, 3.870212229389975445 ) ) ;
#16700=CARTESIAN_POINT ( 'NONE',  ( 36.50000000000002132, 0.000000000000000000, 0.000000000000000000 ) ) ;
#16705=FACE_OUTER_BOUND ( 'NONE', #19620, .T. ) ;
#16711=DIRECTION ( 'NONE',  ( 0.000000000000000000, -0.000000000000000000, -1.000000000000000000 ) ) ;
#16712=CARTESIAN_POINT ( 'NONE',  ( -35.85663232820584057, -3.275050215668913189, -2.949461045527344893 ) ) ;
#16716=FACE_OUTER_BOUND ( 'NONE', #3056, .T. ) ;
#16717=EDGE_CURVE ( 'NONE', #20395, #22807, #27090, .T. ) ;
#16730=ADVANCED_FACE ( 'NONE', ( #684 ), #225, .T. ) ;
#16732=VERTEX_POINT ( 'NONE', #12561 ) ;
#16742=ORIENTED_EDGE ( 'NONE', *, *, #24213, .T. ) ;
#16745=CARTESIAN_POINT ( 'NONE',  ( 50.41431699104522579, 1.130504494894959411, 3.941663789486498537 ) ) ;
#16748=CARTESIAN_POINT ( 'NONE',  ( 57.00381193298470350, 0.7199075706197948232, 1.804244861858284255 ) ) ;
#16750=EDGE_CURVE ( 'NONE', #25510, #24537, #31148, .T. ) ;
#16751=CARTESIAN_POINT ( 'NONE',  ( -54.45996984137642727, -1.500763111530253990, -3.300586169551323668 ) ) ;
#16759=EDGE_CURVE ( 'NONE', #616, #21818, #18002, .T. ) ;
#16761=CARTESIAN_POINT ( 'NONE',  ( -36.81959771849334828, -0.5763363385013906548, 5.380853831843025681 ) ) ;
#16762=VERTEX_POINT ( 'NONE', #14930 ) ;
#16766=ORIENTED_EDGE ( 'NONE', *, *, #31267, .F. ) ;
#16767=CARTESIAN_POINT ( 'NONE',  ( -36.00201293083839715, -4.683225679163161459, 2.703237727951724345 ) ) ;
#16769=CARTESIAN_POINT ( 'NONE',  ( 16.10705563471230661, -0.1565107631087817031, -5.407502298984290690 ) ) ;
#16775=DIRECTION ( 'NONE',  ( 1.000000000000000000, 0.000000000000000000, 0.000000000000000000 ) ) ;
#16776=CARTESIAN_POINT ( 'NONE',  ( 33.47623932017462778, -1.123735532908268331, 5.289358697221549832 ) ) ;
#16781=DIRECTION ( 'NONE',  ( 2.586136946169074517E-16, -1.000000000000000000, 0.000000000000000000 ) ) ;
#16784=ADVANCED_FACE ( 'NONE', ( #19863 ), #29491, .T. ) ;
#16788=CARTESIAN_POINT ( 'NONE',  ( -54.49409853110120139, 1.525884777627348088, -4.047834655405394777 ) ) ;
#16805=VECTOR ( 'NONE', #6722, 1000.000000000000000 ) ;
#16808=DIRECTION ( 'NONE',  ( 0.000000000000000000, 0.000000000000000000, 1.000000000000000000 ) ) ;
#16809=CARTESIAN_POINT ( 'NONE',  ( 15.22780280894127536, -2.525801254963333520, -4.794550361020474050 ) ) ;
#16810=CARTESIAN_POINT ( 'NONE',  ( -36.50489844130380845, 5.244794032782563065, 1.329291831544308300 ) ) ;
#16811=CARTESIAN_POINT ( 'NONE',  ( 15.87128154250933676, -4.872353571451259135, 2.347449169364598021 ) ) ;
#16814=EDGE_LOOP ( 'NONE', ( #8977, #28737, #12583, #1105 ) ) ;
#16818=CARTESIAN_POINT ( 'NONE',  ( 57.03920447585827702, 0.8156862745098039102, -2.468735688885368429 ) ) ;
#16821=EDGE_LOOP ( 'NONE', ( #6750, #4491, #13525, #2339 ) ) ;
#16826=VERTEX_POINT ( 'NONE', #9887 ) ;
#16828=EDGE_CURVE ( 'NONE', #10689, #3458, #4859, .T. ) ;
#16833=CARTESIAN_POINT ( 'NONE',  ( -54.49865678108456279, -1.537045020190658251, 3.323865043138457320 ) ) ;
#16834=CARTESIAN_POINT ( 'NONE',  ( -44.49999999999997868, -1.500000000000000222, -3.300094695611020867 ) ) ;
#16838=CARTESIAN_POINT ( 'NONE',  ( 47.04676887726569134, -4.276948283761179859, 0.9210528638641409804 ) ) ;
#16840=CARTESIAN_POINT ( 'NONE',  ( 15.03925126672132784, 4.804073783693472599, -2.042134687550301475 ) ) ;
#16841=CARTESIAN_POINT ( 'NONE',  ( 54.40000000000001990, 4.041334437186265510E-16, 3.299999999999999822 ) ) ;
#16843=DIRECTION ( 'NONE',  ( -1.000000000000000000, -0.000000000000000000, -0.000000000000000000 ) ) ;
#16845=DIRECTION ( 'NONE',  ( 1.387778780781445676E-14, 8.673617379884035472E-16, 1.000000000000000000 ) ) ;
#16848=EDGE_CURVE ( 'NONE', #28914, #560, #15976, .T. ) ;
#16851=EDGE_CURVE ( 'NONE', #26599, #7189, #22765, .T. ) ;
#16853=EDGE_CURVE ( 'NONE', #29689, #18916, #3350, .T. ) ;
#16863=CARTESIAN_POINT ( 'NONE',  ( 48.50000000000002132, 1.391941090707534023, -3.850000000000022737 ) ) ;
#16866=ORIENTED_EDGE ( 'NONE', *, *, #28233, .F. ) ;
#16867=DIRECTION ( 'NONE',  ( 1.000000000000000000, 0.000000000000000000, 0.000000000000000000 ) ) ;
#16872=CARTESIAN_POINT ( 'NONE',  ( 57.00914817631336717, 0.7715555436188452632, 1.736293111776144205 ) ) ;
#16874=DIRECTION ( 'NONE',  ( 1.000000000000000000, 0.000000000000000000, 0.000000000000000000 ) ) ;
#16877=CIRCLE ( 'NONE', #8748, 4.100000000000022737 ) ;
#16883=ORIENTED_EDGE ( 'NONE', *, *, #10176, .T. ) ;
#16884=FACE_OUTER_BOUND ( 'NONE', #18016, .T. ) ;
#16893=ORIENTED_EDGE ( 'NONE', *, *, #13, .F. ) ;
#16894=CARTESIAN_POINT ( 'NONE',  ( 50.35370852371426764, 1.309359793766484925, 3.864871860988134955 ) ) ;
#16895=ORIENTED_EDGE ( 'NONE', *, *, #12404, .F. ) ;
#16896=CARTESIAN_POINT ( 'NONE',  ( 57.02114622761336449, -0.7499999999999982236, 1.778341845356538498 ) ) ;
#16897=CARTESIAN_POINT ( 'NONE',  ( 57.00965563974653350, 0.7295352771400042124, 1.796193723857490321 ) ) ;
#16898=ADVANCED_FACE ( 'NONE', ( #29821 ), #10972, .F. ) ;
#16899=CARTESIAN_POINT ( 'NONE',  ( 56.95000076968187130, 0.7321971888534951622, -1.754073505128400878 ) ) ;
#16900=VECTOR ( 'NONE', #6351, 1000.000000000000000 ) ;
#16903=FACE_OUTER_BOUND ( 'NONE', #8884, .T. ) ;
#16908=ORIENTED_EDGE ( 'NONE', *, *, #1862, .T. ) ;
#16912=AXIS2_PLACEMENT_3D ( 'NONE', #148, #26576, #7725 ) ;
#16914=ADVANCED_FACE ( 'NONE', ( #25226, #27760 ), #3544, .T. ) ;
#16917=EDGE_CURVE ( 'NONE', #7081, #20639, #15729, .T. ) ;
#16918=CARTESIAN_POINT ( 'NONE',  ( 16.07512358269906372, -0.3169205264062066596, -5.400007398663871250 ) ) ;
#16925=DIRECTION ( 'NONE',  ( -1.000000000000000000, -2.586136946169074517E-16, 0.000000000000000000 ) ) ;
#16930=CARTESIAN_POINT ( 'NONE',  ( 36.50000000000002132, 0.000000000000000000, -1.850000000000000089 ) ) ;
#16931=CARTESIAN_POINT ( 'NONE',  ( 46.92012738450930698, -4.254270342444942621, -1.021450466989925587 ) ) ;
#16932=CARTESIAN_POINT ( 'NONE',  ( 15.71019289815287934, -2.413203405699221094, -4.840238007535771381 ) ) ;
#16937=CARTESIAN_POINT ( 'NONE',  ( 36.50000000000002132, 0.000000000000000000, 0.000000000000000000 ) ) ;
#16940=ORIENTED_EDGE ( 'NONE', *, *, #28015, .F. ) ;
#16942=CARTESIAN_POINT ( 'NONE',  ( 15.66436536804551416, -3.496282614933964528, 4.130238739723520958 ) ) ;
#16950=CARTESIAN_POINT ( 'NONE',  ( 51.80000000000001847, 1.734723475976807094E-15, 0.000000000000000000 ) ) ;
#16952=CARTESIAN_POINT ( 'NONE',  ( 50.38154193469294739, -1.153441674035701636, -3.890342980189690270 ) ) ;
#16958=CYLINDRICAL_SURFACE ( 'NONE', #9469, 4.375000000000000000 ) ;
#16959=DIRECTION ( 'NONE',  ( 1.000000000000000000, 2.586136946169074517E-16, -0.000000000000000000 ) ) ;
#16963=AXIS2_PLACEMENT_3D ( 'NONE', #23770, #30728, #30546 ) ;
#16966=EDGE_LOOP ( 'NONE', ( #6517, #28768, #8295, #18012 ) ) ;
#16971=CARTESIAN_POINT ( 'NONE',  ( -35.85663232820584057, -4.945493884734809775, 1.606888370749721684 ) ) ;
#16975=VERTEX_POINT ( 'NONE', #23649 ) ;
#16976=CIRCLE ( 'NONE', #11390, 0.1000000000000002554 ) ;
#16979=ORIENTED_EDGE ( 'NONE', *, *, #26722, .F. ) ;
#16989=CARTESIAN_POINT ( 'NONE',  ( -36.68866260399460799, 0.7269167730135268624, -5.359285300587757206 ) ) ;
#16990=CIRCLE ( 'NONE', #26082, 0.09999999999999986677 ) ;
#16991=CARTESIAN_POINT ( 'NONE',  ( 47.00000000000002842, -4.131056160354152240, 1.100000000000000311 ) ) ;
#16992=CARTESIAN_POINT ( 'NONE',  ( 48.50000000000002132, 1.391941090707534023, -3.850000000000022737 ) ) ;
#16994=CARTESIAN_POINT ( 'NONE',  ( 15.44631504820159407, 4.878538113278890975, -1.812957040858052871 ) ) ;
#17001=CARTESIAN_POINT ( 'NONE',  ( 48.33019736648184050, -1.141995257496313476, 3.938405479918980490 ) ) ;
#17002=CARTESIAN_POINT ( 'NONE',  ( 48.45343659158886851, -1.329326705022595645, -3.861343257506216098 ) ) ;
#17005=ORIENTED_EDGE ( 'NONE', *, *, #12146, .F. ) ;
#17006=CARTESIAN_POINT ( 'NONE',  ( 33.47623932017462778, -1.123735532908292978, -5.289358697221544503 ) ) ;
#17007=ORIENTED_EDGE ( 'NONE', *, *, #11006, .F. ) ;
#17011=ORIENTED_EDGE ( 'NONE', *, *, #29980, .T. ) ;
#17016=PLANE ( 'NONE',  #30327 ) ;
#17022=CIRCLE ( 'NONE', #3347, 0.4576450603546999840 ) ;
#17023=LINE ( 'NONE', #2750, #5064 ) ;
#17024=EDGE_LOOP ( 'NONE', ( #23176, #21154, #1595, #27742, #7860, #11657, #27859, #21916, #28801, #23206 ) ) ;
#17028=CARTESIAN_POINT ( 'NONE',  ( -54.49983703358571319, -1.542636180423125225, 4.059406436927349482 ) ) ;
#17032=CARTESIAN_POINT ( 'NONE',  ( 57.05000000000001847, -0.7500000000000000000, 2.421260002560649660 ) ) ;
#17035=CARTESIAN_POINT ( 'NONE',  ( -36.11780688638208403, -4.018128186975085114, 3.618665893506928910 ) ) ;
#17037=CIRCLE ( 'NONE', #29157, 0.05000000000000012768 ) ;
#17046=ORIENTED_EDGE ( 'NONE', *, *, #10176, .F. ) ;
#17047=CARTESIAN_POINT ( 'NONE',  ( 51.87241998857975744, 0.05807428590527900780, -4.370869202345071258 ) ) ;
#17048=VERTEX_POINT ( 'NONE', #18419 ) ;
#17051=CYLINDRICAL_SURFACE ( 'NONE', #21831, 0.09999999999999982514 ) ;
#17054=CARTESIAN_POINT ( 'NONE',  ( -35.98994760229917489, 2.686240678228295042, 4.475885392924250361 ) ) ;
#17055=EDGE_LOOP ( 'NONE', ( #18433, #21877 ) ) ;
#17066=LINE ( 'NONE', #2492, #7173 ) ;
#17072=EDGE_CURVE ( 'NONE', #7548, #560, #16488, .T. ) ;
#17077=DIRECTION ( 'NONE',  ( -1.000000000000000000, -0.000000000000000000, -0.000000000000000000 ) ) ;
#17078=ORIENTED_EDGE ( 'NONE', *, *, #529, .T. ) ;
#17081=CARTESIAN_POINT ( 'NONE',  ( -36.38139716712352367, -2.291889356120137222, -4.901871067649458347 ) ) ;
#17085=EDGE_CURVE ( 'NONE', #30343, #13205, #8733, .T. ) ;
#17086=CARTESIAN_POINT ( 'NONE',  ( -36.72207054450174013, -4.892019442464210499, 2.306425897666011693 ) ) ;
#17087=CIRCLE ( 'NONE', #11489, 0.09999999999999993616 ) ;
#17102=CARTESIAN_POINT ( 'NONE',  ( 15.03925126672132961, -1.123735532908273216, 5.289358697221548944 ) ) ;
#17103=CARTESIAN_POINT ( 'NONE',  ( 15.90468948301723273, -2.602043737612640406, -4.741394629686820572 ) ) ;
#17105=DIRECTION ( 'NONE',  ( 1.000000000000000000, 9.742518634817534591E-17, 4.338815227941629246E-17 ) ) ;
#17111=VECTOR ( 'NONE', #7457, 1000.000000000000000 ) ;
#17120=EDGE_CURVE ( 'NONE', #8353, #28219, #6373, .T. ) ;
#17136=CARTESIAN_POINT ( 'NONE',  ( -36.31414349454748702, -4.963067629822554672, -1.552801941062300628 ) ) ;
#17139=ORIENTED_EDGE ( 'NONE', *, *, #16190, .F. ) ;
#17140=ORIENTED_EDGE ( 'NONE', *, *, #30353, .F. ) ;
#17149=FACE_OUTER_BOUND ( 'NONE', #27903, .T. ) ;
#17152=CARTESIAN_POINT ( 'NONE',  ( 16.07512358269905661, 5.037778396015567317, -1.970103387723833865 ) ) ;
#17158=CARTESIAN_POINT ( 'NONE',  ( 33.47623932017462778, 4.683225679163371957, -2.703237727951181668 ) ) ;
#17159=PLANE ( 'NONE',  #29780 ) ;
#17165=ORIENTED_EDGE ( 'NONE', *, *, #15982, .T. ) ;
#17166=ADVANCED_FACE ( 'NONE', ( #12359 ), #5343, .T. ) ;
#17168=CARTESIAN_POINT ( 'NONE',  ( 15.22842924604220016, 5.340403874105067672, 0.9205822089998703106 ) ) ;
#17175=DIRECTION ( 'NONE',  ( 0.000000000000000000, -1.000000000000000000, 0.000000000000000000 ) ) ;
#17180=CARTESIAN_POINT ( 'NONE',  ( 51.74297196358455153, -4.175266387598156825, -1.009028806847065196 ) ) ;
#17181=EDGE_CURVE ( 'NONE', #28219, #19112, #20540, .T. ) ;
#17185=EDGE_CURVE ( 'NONE', #11967, #17261, #11410, .T. ) ;
#17187=VECTOR ( 'NONE', #11774, 1000.000000000000000 ) ;
#17191=AXIS2_PLACEMENT_3D ( 'NONE', #16296, #6955, #23892 ) ;
#17197=DIRECTION ( 'NONE',  ( 1.000000000000000000, 0.000000000000000000, 0.000000000000000000 ) ) ;
#17203=ORIENTED_EDGE ( 'NONE', *, *, #30353, .T. ) ;
#17209=ADVANCED_FACE ( 'NONE', ( #17286 ), #24104, .T. ) ;
#17217=ADVANCED_FACE ( 'NONE', ( #7768 ), #11906, .T. ) ;
#17218=CIRCLE ( 'NONE', #11138, 3.200000000000000178 ) ;
#17220=CARTESIAN_POINT ( 'NONE',  ( 50.37823977475586190, 1.183413901109590105, -3.885761703493072261 ) ) ;
#17221=CARTESIAN_POINT ( 'NONE',  ( 15.32752150720754258, -5.374748457514303190, -0.5963382560600449800 ) ) ;
#17227=VERTEX_POINT ( 'NONE', #12077 ) ;
#17229=VERTEX_POINT ( 'NONE', #17432 ) ;
#17236=DIRECTION ( 'NONE',  ( 0.000000000000000000, 0.000000000000000000, -1.000000000000000000 ) ) ;
#17237=TOROIDAL_SURFACE ( 'NONE', #29856, 4.349999999999997868, 0.05000000000000000278 ) ;
#17239=DIRECTION ( 'NONE',  ( 0.000000000000000000, -0.9875000000000001554, -0.1576190026614806561 ) ) ;
#17241=CARTESIAN_POINT ( 'NONE',  ( -54.45981523601835761, -1.500740478982482973, -4.030402907299741599 ) ) ;
#17249=DIRECTION ( 'NONE',  ( 0.000000000000000000, 0.000000000000000000, -1.000000000000000000 ) ) ;
#17255=LINE ( 'NONE', #24067, #17994 ) ;
#17259=ORIENTED_EDGE ( 'NONE', *, *, #29386, .F. ) ;
#17261=VERTEX_POINT ( 'NONE', #4941 ) ;
#17263=CARTESIAN_POINT ( 'NONE',  ( 57.00875904852982501, 0.7282698412063691729, -2.435189460583063514 ) ) ;
#17265=CARTESIAN_POINT ( 'NONE',  ( 58.50000000000001421, -0.8000000000000000444, 2.421260002560649660 ) ) ;
#17270=B_SPLINE_CURVE_WITH_KNOTS ( 'NONE', 3,
 ( #22146, #10096, #19766, #22299, #17538, #29397, #7859, #7709, #14987, #24654 ),
 .UNSPECIFIED., .F., .F.,
 ( 4, 2, 2, 2, 4 ),
 ( 0.000000000000000000, 0.0004363777631660865864, 0.0006545666447491310181, 0.0007636610855406569202, 0.0008727555263321828223 ),
 .UNSPECIFIED. ) ;
#17271=VECTOR ( 'NONE', #1219, 1000.000000000000000 ) ;
#17274=CARTESIAN_POINT ( 'NONE',  ( 57.00000000000001421, -0.7256347085964565125, -1.800308733460772359 ) ) ;
#17280=ORIENTED_EDGE ( 'NONE', *, *, #29471, .F. ) ;
#17281=ADVANCED_FACE ( 'NONE', ( #29776 ), #6572, .T. ) ;
#17285=CARTESIAN_POINT ( 'NONE',  ( 48.41523095594689607, -1.115727354199206323, -3.895947837398489266 ) ) ;
#17286=FACE_OUTER_BOUND ( 'NONE', #27335, .T. ) ;
#17287=CARTESIAN_POINT ( 'NONE',  ( 51.75297847264299378, -4.174452932061539556, -1.011256013762273920 ) ) ;
#17291=CARTESIAN_POINT ( 'NONE',  ( -36.22818246778668083, -0.6967302926296108367, -5.374298406428810182 ) ) ;
#17294=CARTESIAN_POINT ( 'NONE',  ( 15.30042582489633318, 4.683225673666406408, -2.703237737474395441 ) ) ;
#17296=VERTEX_POINT ( 'NONE', #20451 ) ;
#17297=( BOUNDED_SURFACE ( )  B_SPLINE_SURFACE ( 3, 2, ( 
 ( #14525, #21210, #23728 ),
 ( #1687, #11350, #21038 ),
 ( #18662, #28311, #6618 ),
 ( #4228, #120, #7699 ),
 ( #17220, #12602, #19609 ),
 ( #424, #19440, #12152 ),
 ( #21830, #24645, #27004 ),
 ( #14975, #5641, #12287 ),
 ( #24477, #2498, #17357 ),
 ( #5167, #29388, #22431 ) ),
 .UNSPECIFIED., .F., .F., .T. ) 
 B_SPLINE_SURFACE_WITH_KNOTS ( ( 4, 2, 2, 2, 4 ),
 ( 3, 3 ),
 ( 0.0004005301535625022482, 0.0008279283193725973976, 0.001041627402277645054, 0.001148476943730168936, 0.001255326485182692601 ),
 ( 0.000000000000000000, 1.000000000000000000 ),
 .UNSPECIFIED. ) 
 GEOMETRIC_REPRESENTATION_ITEM ( )  RATIONAL_B_SPLINE_SURFACE ( (
 ( 1.000000000000000000, 0.7071067811865505703, 1.000000000000000000),
 ( 1.000000000000000000, 0.7463463187144504518, 1.000000000000000000),
 ( 1.000000000000000000, 0.7946150999565705364, 1.000000000000000000),
 ( 1.000000000000000000, 0.8720431506958310486, 1.000000000000000000),
 ( 1.000000000000000000, 0.8987780092778684393, 1.000000000000000000),
 ( 1.000000000000000000, 0.9375340664365204857, 1.000000000000000000),
 ( 1.000000000000000000, 0.9504270566176310497, 1.000000000000000000),
 ( 1.000000000000000000, 0.9732249474031181569, 1.000000000000000000),
 ( 1.000000000000000000, 0.9839441327696822892, 1.000000000000000000),
 ( 1.000000000000000000, 0.9842509842514762797, 1.000000000000000000) ) ) 
 REPRESENTATION_ITEM ( '' )  SURFACE ( )  );
#17300=CARTESIAN_POINT ( 'NONE',  ( 15.41080140630239192, 3.722599991951259124, -3.938370952810016590 ) ) ;
#17306=ORIENTED_EDGE ( 'NONE', *, *, #30119, .F. ) ;
#17308=DIRECTION ( 'NONE',  ( 2.586136946169074517E-16, -1.000000000000000000, 0.000000000000000000 ) ) ;
#17319=ORIENTED_EDGE ( 'NONE', *, *, #26681, .F. ) ;
#17322=CARTESIAN_POINT ( 'NONE',  ( -54.47328085509070661, -1.505517457405397996, 4.033720452520547894 ) ) ;
#17324=CARTESIAN_POINT ( 'NONE',  ( 58.50000000000001421, 0.000000000000000000, 0.000000000000000000 ) ) ;
#17326=CARTESIAN_POINT ( 'NONE',  ( -36.31414349454756518, -3.010474646410484123, 4.240315621469648910 ) ) ;
#17327=PLANE ( 'NONE',  #2773 ) ;
#17332=ORIENTED_EDGE ( 'NONE', *, *, #13887, .F. ) ;
#17340=CARTESIAN_POINT ( 'NONE',  ( 47.00000000000002132, 1.734723475976807094E-15, 0.000000000000000000 ) ) ;
#17353=CARTESIAN_POINT ( 'NONE',  ( 15.22842924604237780, -5.340403874104624471, -0.9205822090001011260 ) ) ;
#17356=CARTESIAN_POINT ( 'NONE',  ( 50.50000000000002132, 2.428612866367529932E-14, 0.000000000000000000 ) ) ;
#17357=CARTESIAN_POINT ( 'NONE',  ( 50.33755732750839940, 1.426738769040801769, -3.843750315111145621 ) ) ;
#17358=AXIS2_PLACEMENT_3D ( 'NONE', #17368, #5652, #19913 ) ;
#17360=CARTESIAN_POINT ( 'NONE',  ( 16.08093158123430655, -5.047763082740431173, -1.943828653492548630 ) ) ;
#17365=DIRECTION ( 'NONE',  ( 0.000000000000000000, 1.000000000000000000, 1.532429380227459806E-15 ) ) ;
#17368=CARTESIAN_POINT ( 'NONE',  ( -39.16187796471576377, -1.705048840508494473E-14, 0.000000000000000000 ) ) ;
#17371=DIRECTION ( 'NONE',  ( -1.000000000000000000, -0.000000000000000000, -0.000000000000000000 ) ) ;
#17372=CARTESIAN_POINT ( 'NONE',  ( 58.45000000000001705, 0.7500000000000000000, -1.778341924377873751 ) ) ;
#17373=PLANE ( 'NONE',  #22126 ) ;
#17375=ADVANCED_FACE ( 'NONE', ( #23138 ), #1426, .T. ) ;
#17378=CARTESIAN_POINT ( 'NONE',  ( 56.95000000000001705, 0.000000000000000000, 2.549999999999999822 ) ) ;
#17386=AXIS2_PLACEMENT_3D ( 'NONE', #8951, #8361, #18042 ) ;
#17387=CARTESIAN_POINT ( 'NONE',  ( 15.32766723174653478, -2.228024565339382868, -4.927420728799232208 ) ) ;
#17389=CARTESIAN_POINT ( 'NONE',  ( 57.05000000000001847, 0.7500000000000000000, 1.778341924377873751 ) ) ;
#17391=DIRECTION ( 'NONE',  ( 0.000000000000000000, -1.000000000000000000, 0.000000000000000000 ) ) ;
#17392=CARTESIAN_POINT ( 'NONE',  ( 16.10660252424457184, 0.2875137064282154986, 5.407399902318745788 ) ) ;
#17393=ORIENTED_EDGE ( 'NONE', *, *, #3047, .T. ) ;
#17394=CARTESIAN_POINT ( 'NONE',  ( 15.81621483022863117, -3.777141534544287804, 3.869853550719713375 ) ) ;
#17398=CARTESIAN_POINT ( 'NONE',  ( 15.18463186935388087, 1.123735532908831436, -5.289358697221507200 ) ) ;
#17405=ORIENTED_EDGE ( 'NONE', *, *, #26283, .T. ) ;
#17411=CARTESIAN_POINT ( 'NONE',  ( 15.29449157529458958, -3.378578820314290354, -3.972872285093437927 ) ) ;
#17415=CIRCLE ( 'NONE', #8303, 4.350000000000019185 ) ;
#17416=ORIENTED_EDGE ( 'NONE', *, *, #6509, .F. ) ;
#17419=VERTEX_POINT ( 'NONE', #13753 ) ;
#17421=CARTESIAN_POINT ( 'NONE',  ( -54.44999999999997442, -1.499999999999999556, -3.300094695611020867 ) ) ;
#17425=DIRECTION ( 'NONE',  ( 0.000000000000000000, -1.000000000000000000, 0.000000000000000000 ) ) ;
#17426=CIRCLE ( 'NONE', #25508, 2.649999999999999911 ) ;
#17429=AXIS2_PLACEMENT_3D ( 'NONE', #7646, #17458, #17308 ) ;
#17432=CARTESIAN_POINT ( 'NONE',  ( -54.44999999999997442, 0.000000000000000000, 4.700000000000000178 ) ) ;
#17434=CARTESIAN_POINT ( 'NONE',  ( 51.80595691730878372, -4.272100939101181716, -0.9440912809989533416 ) ) ;
#17444=CARTESIAN_POINT ( 'NONE',  ( 15.41170998834799022, 4.895911367890965593, -2.323639554370032112 ) ) ;
#17445=LINE ( 'NONE', #9714, #20566 ) ;
#17447=CARTESIAN_POINT ( 'NONE',  ( 50.39865716130687190, -0.9106118309512859499, -3.923752762110600312 ) ) ;
#17450=CARTESIAN_POINT ( 'NONE',  ( 15.66436536804550705, 3.496282614933925448, -4.130238739723488095 ) ) ;
#17453=ORIENTED_EDGE ( 'NONE', *, *, #5756, .T. ) ;
#17455=ADVANCED_FACE ( 'NONE', ( #5204 ), #11936, .T. ) ;
#17457=TOROIDAL_SURFACE ( 'NONE', #31106, 2.549999999999999822, 0.05000000000000000278 ) ;
#17458=DIRECTION ( 'NONE',  ( -1.000000000000000000, -2.586136946169074517E-16, 0.000000000000000000 ) ) ;
#17460=ORIENTED_EDGE ( 'NONE', *, *, #16543, .F. ) ;
#17461=CARTESIAN_POINT ( 'NONE',  ( 15.95705409078463433, 5.298557911012508725, 1.088945631943511128 ) ) ;
#17466=CARTESIAN_POINT ( 'NONE',  ( 54.50000000000002132, -0.003244837758135472351, 4.274998768541100169 ) ) ;
#17470=VECTOR ( 'NONE', #21401, 1000.000000000000000 ) ;
#17473=AXIS2_PLACEMENT_3D ( 'NONE', #15878, #4313, #6232 ) ;
#17478=B_SPLINE_CURVE_WITH_KNOTS ( 'NONE', 3,
 ( #18160, #24828, #18458, #759, #25411, #10422, #17392, #28096, #29420, #27036, #15016, #16080, #12634, #17562, #22318, #6110 ),
 .UNSPECIFIED., .F., .F.,
 ( 4, 2, 2, 2, 2, 2, 2, 4 ),
 ( 1.748223473168675632E-18, 0.0004351083927046447584, 0.0008702167854092877821, 0.001740433570818574263, 0.002175541963523217395, 0.002610650356227860094, 0.003045758748932503226, 0.003480867141637146792 ),
 .UNSPECIFIED. ) ;
#17480=CARTESIAN_POINT ( 'NONE',  ( 57.01990854087920013, -0.7399312420039723115, 2.427820937803477630 ) ) ;
#17485=CARTESIAN_POINT ( 'NONE',  ( -36.58413561666692715, -3.261791109367169206, 4.314133646218629714 ) ) ;
#17489=FACE_OUTER_BOUND ( 'NONE', #14594, .T. ) ;
#17493=AXIS2_PLACEMENT_3D ( 'NONE', #9846, #5238, #12523 ) ;
#17502=ORIENTED_EDGE ( 'NONE', *, *, #16363, .F. ) ;
#17504=ORIENTED_EDGE ( 'NONE', *, *, #1348, .T. ) ;
#17506=AXIS2_PLACEMENT_3D ( 'NONE', #6543, #28235, #11915 ) ;
#17508=ORIENTED_EDGE ( 'NONE', *, *, #248, .F. ) ;
#17514=CARTESIAN_POINT ( 'NONE',  ( 15.95705409078465564, -5.298557911012522936, -1.088945631943473602 ) ) ;
#17517=DIRECTION ( 'NONE',  ( -1.000000000000000000, -0.000000000000000000, -0.000000000000000000 ) ) ;
#17526=AXIS2_PLACEMENT_3D ( 'NONE', #1190, #30627, #28427 ) ;
#17528=DIRECTION ( 'NONE',  ( 0.000000000000000000, 0.000000000000000000, -1.000000000000000000 ) ) ;
#17534=CARTESIAN_POINT ( 'NONE',  ( -35.85663232820597557, -2.525801270006294619, -4.794550352686338002 ) ) ;
#17538=CARTESIAN_POINT ( 'NONE',  ( 50.45683212279337226, 1.211455355144567703, -3.917539841352833285 ) ) ;
#17545=AXIS2_PLACEMENT_3D ( 'NONE', #21876, #17, #19339 ) ;
#17547=DIRECTION ( 'NONE',  ( 1.000000000000000000, 0.000000000000000000, 0.000000000000000000 ) ) ;
#17558=DIRECTION ( 'NONE',  ( 0.000000000000000000, -0.1576190026614809614, -0.9875000000000001554 ) ) ;
#17562=CARTESIAN_POINT ( 'NONE',  ( 15.32766723174653123, -1.093755498983960628, 5.295967089285813501 ) ) ;
#17565=CARTESIAN_POINT ( 'NONE',  ( 15.41170998834774686, -2.595074437874647533, 4.757608386865062045 ) ) ;
#17578=VECTOR ( 'NONE', #27179, 1000.000000000000000 ) ;
#17583=DIRECTION ( 'NONE',  ( -1.000000000000000000, -2.586136946169074517E-16, 0.000000000000000000 ) ) ;
#17587=DIRECTION ( 'NONE',  ( 0.000000000000000000, 0.000000000000000000, -1.000000000000000000 ) ) ;
#17593=EDGE_CURVE ( 'NONE', #27011, #26152, #1510, .T. ) ;
#17594=CARTESIAN_POINT ( 'NONE',  ( -36.26369610968610147, -4.878538113278866106, -1.812957040858122149 ) ) ;
#17602=FACE_OUTER_BOUND ( 'NONE', #13728, .T. ) ;
#17604=CARTESIAN_POINT ( 'NONE',  ( 15.98305126557428579, -0.5375162698822371077, 5.381098085087400840 ) ) ;
#17608=CARTESIAN_POINT ( 'NONE',  ( 15.03925126672133139, -5.377732432866646484, -0.5657657256215582464 ) ) ;
#17609=AXIS2_PLACEMENT_3D ( 'NONE', #20866, #6283, #10872 ) ;
#17610=LINE ( 'NONE', #22359, #31198 ) ;
#17611=CARTESIAN_POINT ( 'NONE',  ( 15.59140265158955962, -3.917459231545690646, 3.727878977586795095 ) ) ;
#17614=ORIENTED_EDGE ( 'NONE', *, *, #2709, .T. ) ;
#17615=CARTESIAN_POINT ( 'NONE',  ( 50.49731436448253419, -0.9333771270347004378, -3.994943142064449670 ) ) ;
#17618=CARTESIAN_POINT ( 'NONE',  ( 15.76675455518197566, 3.095036031508724861, -4.435288302043498554 ) ) ;
#17626=DIRECTION ( 'NONE',  ( 1.000000000000000000, 0.000000000000000000, 0.000000000000000000 ) ) ;
#17630=CARTESIAN_POINT ( 'NONE',  ( 15.32766723174652945, 5.374753047227047276, -0.5963205376973405025 ) ) ;
#17633=CARTESIAN_POINT ( 'NONE',  ( 36.50000000000002132, 0.000000000000000000, 0.000000000000000000 ) ) ;
#17639=AXIS2_PLACEMENT_3D ( 'NONE', #26907, #5216, #16808 ) ;
#17650=B_SPLINE_CURVE_WITH_KNOTS ( 'NONE', 3,
 ( #13624, #3823, #23166, #20327, #10952, #3369, #22852, #29958, #8719, #16629, #1449, #8265, #18402, #25210, #1287, #6968 ),
 .UNSPECIFIED., .F., .F.,
 ( 4, 2, 2, 2, 2, 2, 2, 4 ),
 ( 1.734723475976807094E-18, 0.0004351083927046425358, 0.0008702167854092833369, 0.001740433570818564289, 0.002175541963523204819, 0.002610650356227844915, 0.003045758748932485445, 0.003480867141637125975 ),
 .UNSPECIFIED. ) ;
#17653=DIRECTION ( 'NONE',  ( 0.000000000000000000, 0.000000000000000000, -1.000000000000000000 ) ) ;
#17657=EDGE_LOOP ( 'NONE', ( #28547, #1914, #1169, #12814 ) ) ;
#17659=ORIENTED_EDGE ( 'NONE', *, *, #16234, .F. ) ;
#17661=EDGE_LOOP ( 'NONE', ( #28281, #17771, #4288, #22891 ) ) ;
#17664=DIRECTION ( 'NONE',  ( 1.000000000000000000, -0.000000000000000000, -0.000000000000000000 ) ) ;
#17666=VERTEX_POINT ( 'NONE', #23994 ) ;
#17669=ORIENTED_EDGE ( 'NONE', *, *, #11830, .F. ) ;
#17670=ADVANCED_FACE ( 'NONE', ( #7210 ), #6896, .F. ) ;
#17672=ORIENTED_EDGE ( 'NONE', *, *, #23017, .F. ) ;
#17675=VECTOR ( 'NONE', #18856, 1000.000000000000000 ) ;
#17678=( BOUNDED_SURFACE ( )  B_SPLINE_SURFACE ( 3, 2, ( 
 ( #29320, #19829, #47 ),
 ( #5244, #12676, #9849 ),
 ( #26640, #17291, #9710 ),
 ( #14436, #7943, #14751 ),
 ( #19521, #5409, #26934 ),
 ( #7772, #29171, #5100 ),
 ( #15064, #10307, #29615 ),
 ( #4945, #12526, #19976 ),
 ( #4776, #14894, #24111 ),
 ( #2420, #12083, #19682 ),
 ( #24411, #2579, #22052 ),
 ( #21758, #29009, #7318 ),
 ( #16989, #349, #14603 ),
 ( #10018, #20620, #25489 ),
 ( #1429, #1123, #23144 ),
 ( #22834, #5715, #17911 ) ),
 .UNSPECIFIED., .F., .F., .T. ) 
 B_SPLINE_SURFACE_WITH_KNOTS ( ( 4, 2, 2, 2, 2, 2, 2, 4 ),
 ( 3, 3 ),
 ( 0.001780502285214246314, 0.002558945925323777206, 0.002753556835351159658, 0.002948167745378542544, 0.003337389565433307882, 0.003726611385488073219, 0.004115833205542838991, 0.004894276845652369666 ),
 ( 0.000000000000000000, 1.000000000000000000 ),
 .UNSPECIFIED. ) 
 GEOMETRIC_REPRESENTATION_ITEM ( )  RATIONAL_B_SPLINE_SURFACE ( (
 ( 1.000000000000000000, 0.9418517008537227175, 1.000000000000000000),
 ( 1.000000000000000000, 0.9417987965884626611, 1.000000000000000000),
 ( 1.000000000000000000, 0.9418198861734660143, 1.000000000000000000),
 ( 1.000000000000000000, 0.9434060303845427375, 1.000000000000000000),
 ( 1.000000000000000000, 0.9437939819947938069, 1.000000000000000000),
 ( 1.000000000000000000, 0.9445989566713008934, 1.000000000000000000),
 ( 1.000000000000000000, 0.9450169930049703293, 1.000000000000000000),
 ( 1.000000000000000000, 0.9461610507673812176, 1.000000000000000000),
 ( 1.000000000000000000, 0.9467217966427053932, 1.000000000000000000),
 ( 1.000000000000000000, 0.9467345476124492398, 1.000000000000000000),
 ( 1.000000000000000000, 0.9461964028053072573, 1.000000000000000000),
 ( 1.000000000000000000, 0.9446801822473688270, 1.000000000000000000),
 ( 1.000000000000000000, 0.9437582546536396055, 1.000000000000000000),
 ( 1.000000000000000000, 0.9418129560295979141, 1.000000000000000000),
 ( 1.000000000000000000, 0.9418016889777250933, 1.000000000000000000),
 ( 1.000000000000000000, 0.9418517008537231616, 1.000000000000000000) ) ) 
 REPRESENTATION_ITEM ( '' )  SURFACE ( )  );
#17679=VECTOR ( 'NONE', #7116, 1000.000000000000000 ) ;
#17680=CARTESIAN_POINT ( 'NONE',  ( 15.48609859788817289, -4.910307320510440832, -1.715181477143186806 ) ) ;
#17694=CARTESIAN_POINT ( 'NONE',  ( -35.85663232820592583, -2.686240680702151273, -4.475885388010727439 ) ) ;
#17700=CARTESIAN_POINT ( 'NONE',  ( 15.03925126672132784, -0.7747498368337625285, -5.363501452440939232 ) ) ;
#17702=DIRECTION ( 'NONE',  ( -1.000000000000000000, -4.678365685400771632E-16, -1.520093157366894206E-16 ) ) ;
#17709=CARTESIAN_POINT ( 'NONE',  ( 58.50000000000001421, 0.000000000000000000, 2.600000000000000089 ) ) ;
#17721=DIRECTION ( 'NONE',  ( 0.000000000000000000, -1.000000000000000000, 0.000000000000000000 ) ) ;
#17724=EDGE_CURVE ( 'NONE', #5429, #30315, #1251, .T. ) ;
#17726=CARTESIAN_POINT ( 'NONE',  ( 15.67083574136752944, -2.849134329833925783, 4.601168830303218549 ) ) ;
#17731=CARTESIAN_POINT ( 'NONE',  ( -35.98952425903319607, 0.4576450703117207475, 5.200000005133905923 ) ) ;
#17735=CARTESIAN_POINT ( 'NONE',  ( -35.85663232820584057, 0.9159215771349434876, -4.311190327366002606 ) ) ;
#17736=ORIENTED_EDGE ( 'NONE', *, *, #7992, .T. ) ;
#17738=CARTESIAN_POINT ( 'NONE',  ( 50.49739899587713410, -0.9326869175216284669, 3.995127421239668575 ) ) ;
#17739=CARTESIAN_POINT ( 'NONE',  ( 15.49676243306307910, -3.010474646410361110, -4.240315621469747498 ) ) ;
#17741=VERTEX_POINT ( 'NONE', #11650 ) ;
#17744=ADVANCED_FACE ( 'NONE', ( #4823 ), #14171, .F. ) ;
#17750=DIRECTION ( 'NONE',  ( 0.000000000000000000, 0.000000000000000000, 1.000000000000000000 ) ) ;
#17756=VERTEX_POINT ( 'NONE', #10198 ) ;
#17757=AXIS2_PLACEMENT_3D ( 'NONE', #26889, #24675, #13103 ) ;
#17758=EDGE_CURVE ( 'NONE', #6720, #28184, #3784, .T. ) ;
#17762=CARTESIAN_POINT ( 'NONE',  ( 15.74504787372188730, -0.2143423494566188969, 5.404929114625703690 ) ) ;
#17766=ADVANCED_FACE ( 'NONE', ( #2615, #12407 ), #17327, .T. ) ;
#17769=LINE ( 'NONE', #15543, #24609 ) ;
#17771=ORIENTED_EDGE ( 'NONE', *, *, #21900, .F. ) ;
#17772=CARTESIAN_POINT ( 'NONE',  ( 50.36610310744725183, -1.399562922973020429, -3.853849143137397792 ) ) ;
#17775=CARTESIAN_POINT ( 'NONE',  ( 15.22842924604220194, 2.525801262578962536, -4.794550356816757564 ) ) ;
#17778=ORIENTED_EDGE ( 'NONE', *, *, #9024, .T. ) ;
#17783=CARTESIAN_POINT ( 'NONE',  ( 15.97944027357902463, -5.289443499204827148, 1.131445731060769955 ) ) ;
#17787=DIRECTION ( 'NONE',  ( 0.000000000000000000, 0.000000000000000000, -1.000000000000000000 ) ) ;
#17788=DIRECTION ( 'NONE',  ( 0.000000000000000000, -5.942513678379226626E-16, -1.000000000000000000 ) ) ;
#17797=CARTESIAN_POINT ( 'NONE',  ( 50.40000000000001990, 2.428612866367529932E-14, -4.000000000000022204 ) ) ;
#17801=CARTESIAN_POINT ( 'NONE',  ( 51.80000000000835314, -4.135416958146860722, -1.091811499727122881 ) ) ;
#17803=DIRECTION ( 'NONE',  ( 0.000000000000000000, 2.818925648462304271E-14, -1.000000000000000000 ) ) ;
#17804=CARTESIAN_POINT ( 'NONE',  ( 56.96931127949304141, -0.7396072067343685275, -1.750137474527811321 ) ) ;
#17811=EDGE_CURVE ( 'NONE', #15656, #10936, #22492, .T. ) ;
#17827=ORIENTED_EDGE ( 'NONE', *, *, #21006, .F. ) ;
#17833=LINE ( 'NONE', #24632, #9642 ) ;
#17835=CARTESIAN_POINT ( 'NONE',  ( 15.17214319754844887, -4.804073785499189064, -2.042134698606595133 ) ) ;
#17845=CARTESIAN_POINT ( 'NONE',  ( 57.05000000000001847, -0.7500000000000000000, 1.778341924377873751 ) ) ;
#17848=ORIENTED_EDGE ( 'NONE', *, *, #13737, .T. ) ;
#17858=ORIENTED_EDGE ( 'NONE', *, *, #23017, .T. ) ;
#17861=CARTESIAN_POINT ( 'NONE',  ( 57.03577985506672832, -0.7479400494557524315, -1.780189605359982608 ) ) ;
#17865=FACE_OUTER_BOUND ( 'NONE', #31102, .T. ) ;
#17868=CARTESIAN_POINT ( 'NONE',  ( 56.98303665332567647, -0.7553445069156616842, 1.743428900644034885 ) ) ;
#17874=EDGE_LOOP ( 'NONE', ( #18473, #2637 ) ) ;
#17877=EDGE_CURVE ( 'NONE', #30656, #5143, #24306, .T. ) ;
#17888=CARTESIAN_POINT ( 'NONE',  ( 56.95000000000001705, -0.6999999999999999556, 2.452039967047845437 ) ) ;
#17892=FACE_OUTER_BOUND ( 'NONE', #22656, .T. ) ;
#17907=CARTESIAN_POINT ( 'NONE',  ( 16.07279755198631932, -0.3252614978954516678, 5.399488438498854848 ) ) ;
#17908=CARTESIAN_POINT ( 'NONE',  ( 57.04126813003668417, -0.7492316407094400388, -2.421767203557310122 ) ) ;
#17911=CARTESIAN_POINT ( 'NONE',  ( -35.85663232820592583, 0.4576450603546802776, -5.200000000000000178 ) ) ;
#17913=EDGE_CURVE ( 'NONE', #29917, #11630, #27535, .T. ) ;
#17916=CARTESIAN_POINT ( 'NONE',  ( 17.21035195517768557, -2.471857751707525626E-15, 0.000000000000000000 ) ) ;
#17922=CARTESIAN_POINT ( 'NONE',  ( 15.03925126672132961, 2.686240680702205008, -4.475885388010691912 ) ) ;
#17925=ORIENTED_EDGE ( 'NONE', *, *, #23146, .T. ) ;
#17927=CARTESIAN_POINT ( 'NONE',  ( 47.02229336006145388, -4.163003037071927537, 1.036150823695777934 ) ) ;
#17931=CARTESIAN_POINT ( 'NONE',  ( 48.30000000000001847, 2.428612866367529932E-14, 0.000000000000000000 ) ) ;
#17932=ORIENTED_EDGE ( 'NONE', *, *, #16717, .T. ) ;
#17935=ORIENTED_EDGE ( 'NONE', *, *, #17185, .T. ) ;
#17936=DIRECTION ( 'NONE',  ( 0.000000000000000000, 0.000000000000000000, -1.000000000000000000 ) ) ;
#17940=DIRECTION ( 'NONE',  ( 1.520093157366863638E-16, -0.5877852522924685852, -0.8090169943749507819 ) ) ;
#17947=CARTESIAN_POINT ( 'NONE',  ( 57.03951379057714632, -0.7794871794871794934, -1.732743413496389939 ) ) ;
#17954=AXIS2_PLACEMENT_3D ( 'NONE', #21346, #9621, #30975 ) ;
#17956=DIRECTION ( 'NONE',  ( -1.000000000000000000, -0.000000000000000000, 0.000000000000000000 ) ) ;
#17962=CARTESIAN_POINT ( 'NONE',  ( 47.00000000000002132, -1.426739617975173013, -3.843750000000023093 ) ) ;
#17963=VERTEX_POINT ( 'NONE', #30122 ) ;
#17968=DIRECTION ( 'NONE',  ( 1.000000000000000000, -0.000000000000000000, -0.000000000000000000 ) ) ;
#17973=ORIENTED_EDGE ( 'NONE', *, *, #17913, .F. ) ;
#17974=VECTOR ( 'NONE', #15375, 1000.000000000000000 ) ;
#17978=FACE_OUTER_BOUND ( 'NONE', #2944, .T. ) ;
#17980=CARTESIAN_POINT ( 'NONE',  ( 58.45000000000001705, 0.7794871794871796045, -1.732743413496389939 ) ) ;
#17982=CARTESIAN_POINT ( 'NONE',  ( 47.04711921876768344, -4.174487749534351089, -1.011178756798956524 ) ) ;
#17988=CARTESIAN_POINT ( 'NONE',  ( 48.41852494697948828, 1.153996415704716449, 3.890257736381618869 ) ) ;
#17990=CARTESIAN_POINT ( 'NONE',  ( 47.10000000000002274, -3.826179070414207573, 1.000000000000000222 ) ) ;
#17994=VECTOR ( 'NONE', #2382, 1000.000000000000000 ) ;
#18002=CIRCLE ( 'NONE', #10425, 4.275000000000000355 ) ;
#18008=CARTESIAN_POINT ( 'NONE',  ( 15.29449157529457004, -0.3981319440501629447, -5.199999999410266582 ) ) ;
#18012=ORIENTED_EDGE ( 'NONE', *, *, #8640, .F. ) ;
#18015=AXIS2_PLACEMENT_3D ( 'NONE', #11688, #18507, #6302 ) ;
#18016=EDGE_LOOP ( 'NONE', ( #3160, #16365, #19741, #10238 ) ) ;
#18018=FACE_OUTER_BOUND ( 'NONE', #14908, .T. ) ;
#18019=DIRECTION ( 'NONE',  ( 1.000000000000000000, 4.678365685400771632E-16, 1.520093157366894206E-16 ) ) ;
#18020=ORIENTED_EDGE ( 'NONE', *, *, #6526, .F. ) ;
#18028=DIRECTION ( 'NONE',  ( 0.000000000000000000, -0.3589743589743593088, 0.9333474217026304087 ) ) ;
#18031=CIRCLE ( 'NONE', #14492, 0.7500000000000001110 ) ;
#18034=CIRCLE ( 'NONE', #27623, 5.407411300779133789 ) ;
#18036=CARTESIAN_POINT ( 'NONE',  ( 16.10705563471229951, 3.305069970238123211, 4.282766538619565466 ) ) ;
#18037=CARTESIAN_POINT ( 'NONE',  ( 46.90000000000001279, 2.270506450603774156E-15, 4.375000000000000000 ) ) ;
#18038=EDGE_CURVE ( 'NONE', #21791, #21815, #5313, .T. ) ;
#18042=DIRECTION ( 'NONE',  ( 0.000000000000000000, -1.000000000000000000, 0.000000000000000000 ) ) ;
#18061=ORIENTED_EDGE ( 'NONE', *, *, #22187, .F. ) ;
#18062=CIRCLE ( 'NONE', #11473, 1.000000000000000000 ) ;
#18064=DIRECTION ( 'NONE',  ( 1.000000000000000000, 1.293068473084537258E-16, 0.000000000000000000 ) ) ;
#18067=CARTESIAN_POINT ( 'NONE',  ( -36.11780688638071268, -4.683225673667320343, -2.703237737472844238 ) ) ;
#18075=AXIS2_PLACEMENT_3D ( 'NONE', #13884, #30855, #6780 ) ;
#18078=CARTESIAN_POINT ( 'NONE',  ( 15.94709373951305054, -0.6031025731807454493, 5.374022845360696188 ) ) ;
#18080=AXIS2_PLACEMENT_3D ( 'NONE', #9658, #12464, #7579 ) ;
#18081=EDGE_CURVE ( 'NONE', #7189, #6093, #29085, .T. ) ;
#18086=CARTESIAN_POINT ( 'NONE',  ( 50.50000000000002132, 0.6462379109120995890, 4.048750000000023164 ) ) ;
#18090=CARTESIAN_POINT ( 'NONE',  ( 50.38719906715036245, -1.295960864328750128, -3.889961360030737669 ) ) ;
#18092=CIRCLE ( 'NONE', #22139, 0.04999999999999969746 ) ;
#18105=LINE ( 'NONE', #10794, #11760 ) ;
#18106=CARTESIAN_POINT ( 'NONE',  ( -45.15971931043468146, 0.000000000000000000, 4.700000000000000178 ) ) ;
#18113=ORIENTED_EDGE ( 'NONE', *, *, #15444, .F. ) ;
#18114=CARTESIAN_POINT ( 'NONE',  ( 56.96706223141283942, 0.7377629956704406800, -1.750942290135934831 ) ) ;
#18123=CARTESIAN_POINT ( 'NONE',  ( 47.10000000000002274, -3.826179070414207573, 1.000000000000000222 ) ) ;
#18125=EDGE_CURVE ( 'NONE', #618, #25510, #19222, .T. ) ;
#18126=CIRCLE ( 'NONE', #19572, 1.899999999999999911 ) ;
#18127=DIRECTION ( 'NONE',  ( -1.000000000000000000, -2.586136946169074517E-16, 0.000000000000000000 ) ) ;
#18131=DIRECTION ( 'NONE',  ( 1.520093157366878676E-16, -0.5877852522924743583, 0.8090169943749466741 ) ) ;
#18133=CARTESIAN_POINT ( 'NONE',  ( 48.34282069333976040, -1.210123066480733200, 3.917958458743180827 ) ) ;
#18134=ORIENTED_EDGE ( 'NONE', *, *, #22563, .T. ) ;
#18138=ORIENTED_EDGE ( 'NONE', *, *, #27272, .F. ) ;
#18140=( LENGTH_UNIT ( ) NAMED_UNIT ( * ) SI_UNIT ( .MILLI., .METRE. ) );
#18143=CARTESIAN_POINT ( 'NONE',  ( -54.49999999999997868, -4.179189514726506793, -0.8999999999999998002 ) ) ;
#18144=EDGE_LOOP ( 'NONE', ( #19510, #2301, #1147, #879 ) ) ;
#18148=ORIENTED_EDGE ( 'NONE', *, *, #25906, .F. ) ;
#18150=EDGE_CURVE ( 'NONE', #19150, #13242, #25017, .T. ) ;
#18154=EDGE_CURVE ( 'NONE', #25147, #19387, #4302, .T. ) ;
#18159=CARTESIAN_POINT ( 'NONE',  ( -44.49999999999998579, -1.843099986694572142E-14, 0.000000000000000000 ) ) ;
#18160=CARTESIAN_POINT ( 'NONE',  ( 15.03925126672132961, 1.123735532908305634, 5.289358697221540950 ) ) ;
#18164=CARTESIAN_POINT ( 'NONE',  ( 58.50000000000001421, 0.000000000000000000, 0.000000000000000000 ) ) ;
#18165=CARTESIAN_POINT ( 'NONE',  ( 57.01637874260923411, 0.7374533274050908416, -1.789443367489095049 ) ) ;
#18177=ORIENTED_EDGE ( 'NONE', *, *, #5323, .F. ) ;
#18186=CARTESIAN_POINT ( 'NONE',  ( 57.03449256411899881, -0.7475344026195360758, -1.780552047803072302 ) ) ;
#18187=ORIENTED_EDGE ( 'NONE', *, *, #30622, .F. ) ;
#18188=CARTESIAN_POINT ( 'NONE',  ( 50.32838854698020725, 1.409900272549312827, 3.850000494969507248 ) ) ;
#18189=CARTESIAN_POINT ( 'NONE',  ( -35.85663232820584767, 4.383220986679467579, -0.4611378927914189241 ) ) ;
#18192=CARTESIAN_POINT ( 'NONE',  ( -36.30424252565939724, 4.979756346315198812, -1.501439362221551166 ) ) ;
#18198=CARTESIAN_POINT ( 'NONE',  ( -54.44999999999997442, 1.499999999999999556, -3.300094695611021312 ) ) ;
#18200=CARTESIAN_POINT ( 'NONE',  ( 15.03925126672125501, 2.525801270006243548, 4.794550352686353101 ) ) ;
#18201=SHAPE_REPRESENTATION ( 'Body', ( #9018 ), #23745 ) ;
#18204=CARTESIAN_POINT ( 'NONE',  ( 51.70000000000001705, -4.276948333784438283, 0.9210526315789470120 ) ) ;
#18205=EDGE_CURVE ( 'NONE', #23306, #4483, #26795, .T. ) ;
#18207=CARTESIAN_POINT ( 'NONE',  ( -35.85663232820579793, 1.123735532908286316, 5.289358697221541838 ) ) ;
#18208=CARTESIAN_POINT ( 'NONE',  ( 48.42201677308601404, 1.327156576403744959, -3.879406274192464643 ) ) ;
#18209=ADVANCED_FACE ( 'NONE', ( #17149 ), #17678, .T. ) ;
#18214=VERTEX_POINT ( 'NONE', #17608 ) ;
#18215=EDGE_CURVE ( 'NONE', #26599, #4962, #15430, .T. ) ;
#18218=DIRECTION ( 'NONE',  ( 1.000000000000000000, 0.000000000000000000, -4.738179285253040686E-16 ) ) ;
#18220=ORIENTED_EDGE ( 'NONE', *, *, #568, .T. ) ;
#18221=DIRECTION ( 'NONE',  ( 0.000000000000000000, 1.000000000000000000, 0.000000000000000000 ) ) ;
#18222=VECTOR ( 'NONE', #6249, 1000.000000000000000 ) ;
#18227=CARTESIAN_POINT ( 'NONE',  ( -36.04581030752632387, -4.861582136949317068, -2.394243986684321701 ) ) ;
#18230=CARTESIAN_POINT ( 'NONE',  ( 56.95000000000001705, -0.7137254901960785602, 2.500119182087999548 ) ) ;
#18235=CARTESIAN_POINT ( 'NONE',  ( 15.41170998834797246, 0.6969927240736308871, 5.374332520738719587 ) ) ;
#18246=CARTESIAN_POINT ( 'NONE',  ( -36.92398358572908990, 3.410993390446889872, -4.205682099886818293 ) ) ;
#18252=CARTESIAN_POINT ( 'NONE',  ( 47.00572760024188312, -4.149162114478044394, 1.064915450748001424 ) ) ;
#18258=ORIENTED_EDGE ( 'NONE', *, *, #22542, .T. ) ;
#18263=ORIENTED_EDGE ( 'NONE', *, *, #30205, .T. ) ;
#18264=CARTESIAN_POINT ( 'NONE',  ( 56.99280487254718253, 0.7628505807388673565, -1.740142286037820618 ) ) ;
#18266=VERTEX_POINT ( 'NONE', #25190 ) ;
#18270=CARTESIAN_POINT ( 'NONE',  ( -44.49999999999997868, 4.700000000000000178, 0.000000000000000000 ) ) ;
#18272=CARTESIAN_POINT ( 'NONE',  ( -35.85663232820584057, 4.018128179617551865, -3.618665901676622720 ) ) ;
#18278=CARTESIAN_POINT ( 'NONE',  ( 56.95000000000001705, 0.7255611966503594523, 2.496740365009429752 ) ) ;
#18279=CARTESIAN_POINT ( 'NONE',  ( 48.30268969835653792, -0.9327905306641465222, 3.995066436131524235 ) ) ;
#18285=DIRECTION ( 'NONE',  ( -1.000000000000000000, -0.000000000000000000, -0.000000000000000000 ) ) ;
#18288=CARTESIAN_POINT ( 'NONE',  ( 56.95118308248727601, 0.7317690799413573144, -2.494914055551520793 ) ) ;
#18297=CARTESIAN_POINT ( 'NONE',  ( 36.55000000000001847, 0.000000000000000000, 0.000000000000000000 ) ) ;
#18299=ORIENTED_EDGE ( 'NONE', *, *, #4292, .T. ) ;
#18303=CARTESIAN_POINT ( 'NONE',  ( 15.18459684427939926, 4.018128179617495022, 3.618665901676702656 ) ) ;
#18312=AXIS2_PLACEMENT_3D ( 'NONE', #78, #19400, #29042 ) ;
#18314=FACE_OUTER_BOUND ( 'NONE', #24886, .T. ) ;
#18315=ADVANCED_FACE ( 'NONE', ( #25344 ), #20771, .T. ) ;
#18320=ORIENTED_EDGE ( 'NONE', *, *, #6943, .F. ) ;
#18332=EDGE_CURVE ( 'NONE', #27746, #24537, #23610, .T. ) ;
#18333=ORIENTED_EDGE ( 'NONE', *, *, #18991, .F. ) ;
#18334=DIRECTION ( 'NONE',  ( 1.000000000000000000, 0.000000000000000000, -0.000000000000000000 ) ) ;
#18339=CARTESIAN_POINT ( 'NONE',  ( -36.22909104983143180, 5.326676561279607647, -0.9978806102894379748 ) ) ;
#18341=CARTESIAN_POINT ( 'NONE',  ( -36.00197790576392265, -4.018128179617563411, 3.618665901676646701 ) ) ;
#18344=ADVANCED_FACE ( 'NONE', ( #31027 ), #23441, .T. ) ;
#18346=CYLINDRICAL_SURFACE ( 'NONE', #23096, 1.000000000000000000 ) ;
#18354=ORIENTED_EDGE ( 'NONE', *, *, #16828, .T. ) ;
#18371=CARTESIAN_POINT ( 'NONE',  ( 57.05000000000001847, -0.8156862745098041323, 2.468735688885368873 ) ) ;
#18375=ADVANCED_FACE ( 'NONE', ( #6502 ), #14090, .F. ) ;
#18376=CARTESIAN_POINT ( 'NONE',  ( 47.03019939778821623, -4.166995010554928491, -1.027517533905029090 ) ) ;
#18378=CARTESIAN_POINT ( 'NONE',  ( -36.22955757456080761, 2.840625797034106448, -4.363718033548086517 ) ) ;
#18379=CARTESIAN_POINT ( 'NONE',  ( 58.45000000000001705, -0.8156862745098041323, -2.468735688885368873 ) ) ;
#18385=AXIS2_PLACEMENT_3D ( 'NONE', #10940, #27883, #1437 ) ;
#18390=CARTESIAN_POINT ( 'NONE',  ( 50.40000000000001279, -0.6462379109120511833, -4.048750000000022276 ) ) ;
#18391=B_SPLINE_CURVE_WITH_KNOTS ( 'NONE', 3,
 ( #29368, #21810, #9905, #9756, #29509, #12271, #27154, #240, #99, #10361, #8001, #19879, #701, #20038, #29682, #5149 ),
 .UNSPECIFIED., .F., .F.,
 ( 4, 2, 2, 2, 2, 2, 2, 4 ),
 ( 1.738108305489988542E-18, 0.0004351083927046406927, 0.0008702167854092796506, 0.001740433570818558217, 0.002175541963523197446, 0.002610650356227837109, 0.003045758748932476771, 0.003480867141637116434 ),
 .UNSPECIFIED. ) ;
#18392=CARTESIAN_POINT ( 'NONE',  ( -54.49999999999997868, 9.184850993605150903E-17, 0.7500000000000001110 ) ) ;
#18395=CARTESIAN_POINT ( 'NONE',  ( 15.22780280894164129, -5.340403875751315255, 0.9205822004573636086 ) ) ;
#18396=VERTEX_POINT ( 'NONE', #16649 ) ;
#18398=DIRECTION ( 'NONE',  ( 1.000000000000000000, 0.000000000000000000, 0.000000000000000000 ) ) ;
#18399=ORIENTED_EDGE ( 'NONE', *, *, #8503, .T. ) ;
#18402=CARTESIAN_POINT ( 'NONE',  ( 15.59140265158955607, 3.917459231545712850, -3.727878977586764009 ) ) ;
#18408=ORIENTED_EDGE ( 'NONE', *, *, #30476, .T. ) ;
#18417=CARTESIAN_POINT ( 'NONE',  ( 56.95349779155813508, -0.7404564066163630276, 2.492333105726597164 ) ) ;
#18419=CARTESIAN_POINT ( 'NONE',  ( 57.05000000000001847, 0.8156862745098041323, 2.468735688885368873 ) ) ;
#18421=CARTESIAN_POINT ( 'NONE',  ( -54.49999999999997868, -1.550000000000000044, 3.300094695611020867 ) ) ;
#18422=CARTESIAN_POINT ( 'NONE',  ( -36.79682133506354091, 4.944296796129599159, -2.193698057025677439 ) ) ;
#18423=DIRECTION ( 'NONE',  ( 0.000000000000000000, 0.000000000000000000, 1.000000000000000000 ) ) ;
#18424=DIRECTION ( 'NONE',  ( -1.520093157366847861E-16, 0.5877852522924624790, 0.8090169943749551118 ) ) ;
#18425=CARTESIAN_POINT ( 'NONE',  ( 58.45000000000001705, 0.8000000000000001554, -1.778341924377873973 ) ) ;
#18429=CARTESIAN_POINT ( 'NONE',  ( 56.95000000000001705, 0.7137254901960784492, -2.500119182087999548 ) ) ;
#18430=AXIS2_PLACEMENT_3D ( 'NONE', #2396, #7001, #4920 ) ;
#18432=B_SPLINE_CURVE_WITH_KNOTS ( 'NONE', 3,
 ( #15202, #3166, #787, #10456, #14876, #20135, #5227, #7462, #29766, #27390, #5699, #15350, #9831, #21887, #19498, #328 ),
 .UNSPECIFIED., .F., .F.,
 ( 4, 3, 3, 3, 3, 4 ),
 ( 0.000000000000000000, 3.843454199181276345E-05, 7.602611568626176531E-05, 0.0001118455301991774195, 0.0001459326773459513119, 0.0001653157283245150629 ),
 .UNSPECIFIED. ) ;
#18433=ORIENTED_EDGE ( 'NONE', *, *, #2171, .T. ) ;
#18436=ORIENTED_EDGE ( 'NONE', *, *, #20198, .F. ) ;
#18441=CARTESIAN_POINT ( 'NONE',  ( 56.99824518417612751, 0.8016297048612398557, -2.473345119325445651 ) ) ;
#18444=CARTESIAN_POINT ( 'NONE',  ( 58.45000000000001705, -0.7794871794871796045, -1.732743413496389939 ) ) ;
#18445=ORIENTED_EDGE ( 'NONE', *, *, #18215, .T. ) ;
#18455=EDGE_CURVE ( 'NONE', #12071, #26911, #21003, .T. ) ;
#18458=CARTESIAN_POINT ( 'NONE',  ( 15.32752150720753725, 1.093737229520479692, 5.295968199484769379 ) ) ;
#18459=CIRCLE ( 'NONE', #4286, 1.000000000000000000 ) ;
#18460=CARTESIAN_POINT ( 'NONE',  ( 57.03828022491683924, -0.8151581666669124315, -2.468910358759941914 ) ) ;
#18465=CARTESIAN_POINT ( 'NONE',  ( 57.00000000000001421, 0.7059996929583092218, -1.815412393553804460 ) ) ;
#18473=ORIENTED_EDGE ( 'NONE', *, *, #4082, .T. ) ;
#18475=ORIENTED_EDGE ( 'NONE', *, *, #29371, .F. ) ;
#18482=CARTESIAN_POINT ( 'NONE',  ( -35.85663232820581925, 3.426725943139507624, 3.937891353488775170 ) ) ;
#18486=CARTESIAN_POINT ( 'NONE',  ( 57.05000000000001847, -0.7500000000000000000, -1.778341924377873751 ) ) ;
#18487=ORIENTED_EDGE ( 'NONE', *, *, #29531, .T. ) ;
#18488=CARTESIAN_POINT ( 'NONE',  ( 57.00000000000001421, 0.6999999999999999556, -2.452039967047845437 ) ) ;
#18491=VERTEX_POINT ( 'NONE', #26895 ) ;
#18494=EDGE_CURVE ( 'NONE', #12299, #8533, #20538, .T. ) ;
#18497=ADVANCED_FACE ( 'NONE', ( #31197 ), #9526, .T. ) ;
#18507=DIRECTION ( 'NONE',  ( 0.000000000000000000, -1.000000000000000000, 0.000000000000000000 ) ) ;
#18508=CARTESIAN_POINT ( 'NONE',  ( -36.30347965937240673, 0.1138661108245775516, 5.199999999057504319 ) ) ;
#18510=ORIENTED_EDGE ( 'NONE', *, *, #28677, .T. ) ;
#18512=ORIENTED_EDGE ( 'NONE', *, *, #12120, .F. ) ;
#18514=CARTESIAN_POINT ( 'NONE',  ( 48.40000000000002700, 0.6304760106459517122, 3.950000000000022826 ) ) ;
#18523=DIRECTION ( 'NONE',  ( 0.000000000000000000, 0.000000000000000000, 1.000000000000000000 ) ) ;
#18527=AXIS2_PLACEMENT_3D ( 'NONE', #23244, #30195, #21023 ) ;
#18528=TOROIDAL_SURFACE ( 'NONE', #5376, 4.350000000000019185, 0.05000000000000000278 ) ;
#18539=AXIS2_PLACEMENT_3D ( 'NONE', #15390, #25039, #3370 ) ;
#18545=AXIS2_PLACEMENT_3D ( 'NONE', #29053, #27296, #3076 ) ;
#18546=CARTESIAN_POINT ( 'NONE',  ( 15.03925126672132784, 3.817150320980643663, 2.203324261490567704 ) ) ;
#18552=ORIENTED_EDGE ( 'NONE', *, *, #6648, .F. ) ;
#18554=DIRECTION ( 'NONE',  ( -1.000000000000000000, -0.000000000000000000, -0.000000000000000000 ) ) ;
#18557=CARTESIAN_POINT ( 'NONE',  ( -35.85663232820583346, -5.377732432866659806, -0.5657657256215629094 ) ) ;
#18566=ORIENTED_EDGE ( 'NONE', *, *, #12321, .T. ) ;
#18570=CYLINDRICAL_SURFACE ( 'NONE', #29318, 1.000000000000000000 ) ;
#18572=VERTEX_POINT ( 'NONE', #19646 ) ;
#18577=AXIS2_PLACEMENT_3D ( 'NONE', #19678, #2719, #7770 ) ;
#18579=VECTOR ( 'NONE', #14568, 1000.000000000000000 ) ;
#18584=CARTESIAN_POINT ( 'NONE',  ( -36.14490256869206064, 5.374748457514291644, -0.5963382560599886917 ) ) ;
#18586=AXIS2_PLACEMENT_3D ( 'NONE', #15820, #18523, #25472 ) ;
#18589=CARTESIAN_POINT ( 'NONE',  ( 15.86395258069111414, 5.320649567603495278, -0.9667173501063296426 ) ) ;
#18590=DIRECTION ( 'NONE',  ( 0.000000000000000000, 0.000000000000000000, -1.000000000000000000 ) ) ;
#18593=DIRECTION ( 'NONE',  ( 0.000000000000000000, 0.000000000000000000, -1.000000000000000000 ) ) ;
#18594=ORIENTED_EDGE ( 'NONE', *, *, #16759, .F. ) ;
#18596=CARTESIAN_POINT ( 'NONE',  ( 50.40000000000001990, -0.6462379109120509613, 4.048750000000022276 ) ) ;
#18597=EDGE_CURVE ( 'NONE', #26864, #25905, #17255, .T. ) ;
#18603=CIRCLE ( 'NONE', #7452, 0.4576450603546999840 ) ;
#18604=DIRECTION ( 'NONE',  ( 0.000000000000000000, 1.000000000000000000, 0.000000000000000000 ) ) ;
#18607=ORIENTED_EDGE ( 'NONE', *, *, #12479, .F. ) ;
#18615=CARTESIAN_POINT ( 'NONE',  ( -35.85663232820584057, -3.426725943139554698, -3.937891353488750301 ) ) ;
#18617=EDGE_LOOP ( 'NONE', ( #22144, #11255, #25087, #25714 ) ) ;
#18622=CARTESIAN_POINT ( 'NONE',  ( 47.01037571208187416, -4.157296476791674245, -1.048491968755484560 ) ) ;
#18624=CARTESIAN_POINT ( 'NONE',  ( 15.03925126672132784, 4.683225679163368405, -2.703237727951182112 ) ) ;
#18636=EDGE_CURVE ( 'NONE', #18736, #20389, #7877, .T. ) ;
#18642=CARTESIAN_POINT ( 'NONE',  ( -36.26369610968607304, 2.881190829692216848, 4.334245811858008501 ) ) ;
#18644=ORIENTED_EDGE ( 'NONE', *, *, #27542, .F. ) ;
#18650=FACE_OUTER_BOUND ( 'NONE', #29482, .T. ) ;
#18653=CARTESIAN_POINT ( 'NONE',  ( -35.85663232820595425, 5.340403872473318714, -0.9205822173395590280 ) ) ;
#18662=CARTESIAN_POINT ( 'NONE',  ( 50.39869454013827976, 0.9107929593200400076, -3.923749358243191043 ) ) ;
#18668=CARTESIAN_POINT ( 'NONE',  ( -36.25997906085252254, 0.2181161761758398654, 5.200000001420970186 ) ) ;
#18669=LINE ( 'NONE', #30997, #15022 ) ;
#18679=FACE_BOUND ( 'NONE', #1177, .T. ) ;
#18682=DIRECTION ( 'NONE',  ( -1.000000000000000000, 0.000000000000000000, 0.000000000000000000 ) ) ;
#18687=CARTESIAN_POINT ( 'NONE',  ( -36.40878371307408656, 3.917459231545620035, 3.727878977586848386 ) ) ;
#18692=CARTESIAN_POINT ( 'NONE',  ( -54.47710365256552478, 1.507983431629474014, -4.035431478432994545 ) ) ;
#18693=CIRCLE ( 'NONE', #28788, 4.100000000000022737 ) ;
#18695=CARTESIAN_POINT ( 'NONE',  ( 57.05000000000001847, -0.7500000000000000000, 1.778341924377873751 ) ) ;
#18697=AXIS2_PLACEMENT_3D ( 'NONE', #6788, #9178, #11851 ) ;
#18699=CARTESIAN_POINT ( 'NONE',  ( -44.49999999999997868, 1.499999999999999556, -4.029888335921975262 ) ) ;
#18703=CARTESIAN_POINT ( 'NONE',  ( 15.32766723174653301, 1.093755498983968399, -5.295967089285809948 ) ) ;
#18704=CIRCLE ( 'NONE', #10105, 0.4576450603546982632 ) ;
#18713=EDGE_CURVE ( 'NONE', #6507, #31094, #612, .T. ) ;
#18715=DIRECTION ( 'NONE',  ( 1.000000000000000000, 2.586136946169074517E-16, -0.000000000000000000 ) ) ;
#18717=CARTESIAN_POINT ( 'NONE',  ( -36.25997906085275702, 5.012895491272595372, 1.399447560527683931 ) ) ;
#18720=ORIENTED_EDGE ( 'NONE', *, *, #20074, .F. ) ;
#18721=CARTESIAN_POINT ( 'NONE',  ( -36.30424252565902776, -4.979756346315149962, 1.501439362221238083 ) ) ;
#18722=CARTESIAN_POINT ( 'NONE',  ( 50.40000000000001279, -0.7619326981554289668, 3.939508824314739144 ) ) ;
#18730=EDGE_CURVE ( 'NONE', #22370, #518, #21169, .T. ) ;
#18736=VERTEX_POINT ( 'NONE', #5529 ) ;
#18739=CARTESIAN_POINT ( 'NONE',  ( 56.97354279652698494, -0.7803351525568237301, 2.480154250529269522 ) ) ;
#18742=ADVANCED_FACE ( 'NONE', ( #15182 ), #24834, .F. ) ;
#18748=DIRECTION ( 'NONE',  ( 1.000000000000000000, 0.000000000000000000, 0.000000000000000000 ) ) ;
#18750=CARTESIAN_POINT ( 'NONE',  ( 56.99032252660322939, 0.7964187825544630783, 2.475026498169530687 ) ) ;
#18751=B_SPLINE_CURVE_WITH_KNOTS ( 'NONE', 3,
 ( #25531, #21135, #30766, #9075, #13326, #23190, #30438, #18750, #11277, #1617, #23021, #25388, #6696, #11611, #18278, #16357 ),
 .UNSPECIFIED., .F., .F.,
 ( 4, 3, 3, 3, 3, 4 ),
 ( 0.000000000000000000, 1.754151282668922588E-05, 5.222880005687533889E-05, 8.869434694929045231E-05, 0.0001259176481356621589, 0.0001632567749836554797 ),
 .UNSPECIFIED. ) ;
#18753=CARTESIAN_POINT ( 'NONE',  ( 50.34130827207516745, 1.344780351710889610, -3.858600739747802599 ) ) ;
#18755=CARTESIAN_POINT ( 'NONE',  ( 47.00000000000002132, -1.391941090707485396, -3.750000000000022649 ) ) ;
#18762=ORIENTED_EDGE ( 'NONE', *, *, #9032, .F. ) ;
#18769=DIRECTION ( 'NONE',  ( 0.000000000000000000, 0.000000000000000000, -1.000000000000000000 ) ) ;
#18770=CARTESIAN_POINT ( 'NONE',  ( 57.00000000000001421, 0.6999999999999999556, 2.489477856900920383 ) ) ;
#18771=ORIENTED_EDGE ( 'NONE', *, *, #969, .T. ) ;
#18773=LINE ( 'NONE', #16384, #16805 ) ;
#18775=CARTESIAN_POINT ( 'NONE',  ( 56.95000000000001705, -0.7255611966503594523, -2.496740365009429752 ) ) ;
#18777=AXIS2_PLACEMENT_3D ( 'NONE', #16971, #19963, #10000 ) ;
#18784=CARTESIAN_POINT ( 'NONE',  ( 57.03469936322583322, 0.7478111487523275702, -1.780306085601951027 ) ) ;
#18785=CARTESIAN_POINT ( 'NONE',  ( -35.85663232820579793, -2.199885893005965709, 4.939696249117681681 ) ) ;
#18794=VERTEX_POINT ( 'NONE', #9313 ) ;
#18802=ORIENTED_EDGE ( 'NONE', *, *, #4075, .F. ) ;
#18806=ORIENTED_EDGE ( 'NONE', *, *, #5826, .T. ) ;
#18807=CARTESIAN_POINT ( 'NONE',  ( -36.89831264271881395, 5.226279933021899637, 1.394410282272850132 ) ) ;
#18812=CARTESIAN_POINT ( 'NONE',  ( -36.14490256869205353, 1.093737229520459486, -5.295968199484771155 ) ) ;
#18816=CARTESIAN_POINT ( 'NONE',  ( 51.88150799779677413, 0.02572195732724835704, 4.373259675815027947 ) ) ;
#18820=CARTESIAN_POINT ( 'NONE',  ( 58.45000000000001705, 0.8000000000000000444, 2.421260002560650104 ) ) ;
#18824=B_SPLINE_CURVE_WITH_KNOTS ( 'NONE', 3,
 ( #23293, #31194, #28188, #6500, #28500, #9029, #25810, #23440, #1727, #11395, #4266, #21084, #30724, #18703, #17398, #22173 ),
 .UNSPECIFIED., .F., .F.,
 ( 4, 2, 2, 2, 2, 2, 2, 4 ),
 ( 1.748223473168675632E-18, 0.0004351083927046442705, 0.0008702167854092868063, 0.001740433570818572312, 0.002175541963523215227, 0.002610650356227857492, 0.003045758748932500190, 0.003480867141637142888 ),
 .UNSPECIFIED. ) ;
#18827=CARTESIAN_POINT ( 'NONE',  ( -36.89017861347081606, 0.3252614978953461411, 5.399488438498862841 ) ) ;
#18828=CARTESIAN_POINT ( 'NONE',  ( 48.41509867277373047, 1.114141714781645254, -3.896173399896523559 ) ) ;
#18830=EDGE_CURVE ( 'NONE', #26982, #14402, #30843, .T. ) ;
#18836=CARTESIAN_POINT ( 'NONE',  ( 57.05000000000001847, -0.6999999999999999556, 0.000000000000000000 ) ) ;
#18837=ORIENTED_EDGE ( 'NONE', *, *, #31135, .F. ) ;
#18838=ORIENTED_EDGE ( 'NONE', *, *, #22298, .F. ) ;
#18839=CARTESIAN_POINT ( 'NONE',  ( -35.85663232820584057, -0.4576450603547173035, -5.200000000000000178 ) ) ;
#18841=DIRECTION ( 'NONE',  ( 0.000000000000000000, 0.000000000000000000, -1.000000000000000000 ) ) ;
#18849=( BOUNDED_SURFACE ( )  B_SPLINE_SURFACE ( 3, 2, ( 
 ( #22048, #7769, #14747 ),
 ( #15216, #3029, #9847 ),
 ( #17287, #7480, #17434 ),
 ( #12524, #496, #24407 ),
 ( #27083, #10155, #3180 ),
 ( #5404, #2718, #19822 ) ),
 .UNSPECIFIED., .F., .F., .F. ) 
 B_SPLINE_SURFACE_WITH_KNOTS ( ( 4, 2, 4 ),
 ( 3, 3 ),
 ( 0.0001319104779587709254, 0.0002905946498119449514, 0.0004492788216651189773 ),
 ( 0.000000000000000000, 1.000000000000000000 ),
 .UNSPECIFIED. ) 
 GEOMETRIC_REPRESENTATION_ITEM ( )  RATIONAL_B_SPLINE_SURFACE ( (
 ( 1.000000000000000000, 0.7779866052154992273, 1.000000000000000000),
 ( 1.000000000000000000, 0.7780052684394707097, 1.000000000000000000),
 ( 1.000000000000000000, 0.7724636952541394930, 1.000000000000000000),
 ( 1.000000000000000000, 0.7490013934200028256, 1.000000000000000000),
 ( 1.000000000000000000, 0.7305684325697047177, 1.000000000000000000),
 ( 1.000000000000000000, 0.7071067811865716646, 1.000000000000000000) ) ) 
 REPRESENTATION_ITEM ( '' )  SURFACE ( )  );
#18851=CARTESIAN_POINT ( 'NONE',  ( -54.47328085509070661, 1.505517457405397774, -4.033720452520548783 ) ) ;
#18855=CARTESIAN_POINT ( 'NONE',  ( -36.26369610968610147, 3.231775792180371809, -4.079530926931222545 ) ) ;
#18856=DIRECTION ( 'NONE',  ( 0.9913331294122580406, 0.1313720918981625962, 0.000000000000000000 ) ) ;
#18858=CARTESIAN_POINT ( 'NONE',  ( 57.00103033359725657, -0.7116617362530316404, -2.445288145576760552 ) ) ;
#18859=CYLINDRICAL_SURFACE ( 'NONE', #9984, 4.299999999999998046 ) ;
#18861=DIRECTION ( 'NONE',  ( 0.000000000000000000, 0.000000000000000000, -1.000000000000000000 ) ) ;
#18869=CARTESIAN_POINT ( 'NONE',  ( 15.45522337368515764, -2.900433254920993242, -4.320265374240207734 ) ) ;
#18870=CARTESIAN_POINT ( 'NONE',  ( -36.38012252111052902, 5.369990034204258578, 0.6654225812210384783 ) ) ;
#18871=CARTESIAN_POINT ( 'NONE',  ( 15.94709373951294218, -5.297368390263452298, 1.087079755157607242 ) ) ;
#18874=CARTESIAN_POINT ( 'NONE',  ( 48.46289871413547701, 1.426739617975221863, 3.843750000000023981 ) ) ;
#18875=PLANE ( 'NONE',  #693 ) ;
#18896=CARTESIAN_POINT ( 'NONE',  ( 58.45000000000001705, 0.8000000000000000444, -2.421260002560650104 ) ) ;
#18897=FACE_OUTER_BOUND ( 'NONE', #15817, .T. ) ;
#18899=CARTESIAN_POINT ( 'NONE',  ( 15.03925126672125145, 5.340403872473335589, -0.9205822173395469266 ) ) ;
#18904=ORIENTED_EDGE ( 'NONE', *, *, #28988, .T. ) ;
#18905=DIRECTION ( 'NONE',  ( 0.000000000000000000, 0.000000000000000000, -1.000000000000000000 ) ) ;
#18916=VERTEX_POINT ( 'NONE', #23259 ) ;
#18918=CARTESIAN_POINT ( 'NONE',  ( 15.29384114148383667, 4.822476035523743931, 1.985498375066824472 ) ) ;
#18926=ORIENTED_EDGE ( 'NONE', *, *, #11089, .F. ) ;
#18927=ORIENTED_EDGE ( 'NONE', *, *, #15994, .F. ) ;
#18930=CYLINDRICAL_SURFACE ( 'NONE', #23877, 1.000000000000000000 ) ;
#18937=CARTESIAN_POINT ( 'NONE',  ( 57.02888841125436414, 0.7778303923484506388, 1.733491207451775207 ) ) ;
#18942=FACE_OUTER_BOUND ( 'NONE', #12920, .T. ) ;
#18944=DIRECTION ( 'NONE',  ( 0.000000000000000000, 0.000000000000000000, 1.000000000000000000 ) ) ;
#18947=CIRCLE ( 'NONE', #31062, 30.00000000000000355 ) ;
#18948=CARTESIAN_POINT ( 'NONE',  ( 51.81783829102215577, 0.6462660169415540556, -4.286374879252671910 ) ) ;
#18953=CARTESIAN_POINT ( 'NONE',  ( -36.63359589171323449, 3.777141534544248724, 3.869853550719733359 ) ) ;
#18957=CARTESIAN_POINT ( 'NONE',  ( 50.40000000000001990, -0.6304760106459028624, 3.950000000000022826 ) ) ;
#18961=CARTESIAN_POINT ( 'NONE',  ( -36.79682133506354091, 5.289443499204790733, 1.131445731060841453 ) ) ;
#18962=CARTESIAN_POINT ( 'NONE',  ( 33.47623932017462778, 4.683225679163328437, 2.703237727951257607 ) ) ;
#18965=CARTESIAN_POINT ( 'NONE',  ( 57.05000000000001137, -0.7500000000000001110, 1.778341924377885963 ) ) ;
#18967=CARTESIAN_POINT ( 'NONE',  ( -54.44999999999997442, -1.500000000000000222, -3.300094695611020867 ) ) ;
#18984=CARTESIAN_POINT ( 'NONE',  ( -36.40878371307407235, -4.755985070912294610, 2.573747172434699859 ) ) ;
#18985=EDGE_LOOP ( 'NONE', ( #25760, #7757, #21192, #26315 ) ) ;
#18991=EDGE_CURVE ( 'NONE', #7548, #4176, #23557, .T. ) ;
#18992=ORIENTED_EDGE ( 'NONE', *, *, #27001, .F. ) ;
#18996=CARTESIAN_POINT ( 'NONE',  ( 57.05000000000001847, 0.6999999999999999556, 0.000000000000000000 ) ) ;
#19003=CARTESIAN_POINT ( 'NONE',  ( -36.14504829323104929, 3.997758138077510015, 3.641634024966127203 ) ) ;
#19004=AXIS2_PLACEMENT_3D ( 'NONE', #20959, #4484, #11612 ) ;
#19012=CARTESIAN_POINT ( 'NONE',  ( -36.58413561666603186, 3.261791109367091934, -4.314133646218116347 ) ) ;
#19022=CARTESIAN_POINT ( 'NONE',  ( -35.85663232820584057, 4.804073783693418420, 2.042134687550397398 ) ) ;
#19024=CARTESIAN_POINT ( 'NONE',  ( 15.03925126672122836, -2.199885893005920856, -4.939696249117695892 ) ) ;
#19025=CARTESIAN_POINT ( 'NONE',  ( -36.89250464418361020, 5.037778396015492710, 1.970103387723980415 ) ) ;
#19030=DIRECTION ( 'NONE',  ( 1.000000000000000000, 1.293068473084537258E-16, 0.000000000000000000 ) ) ;
#19031=EDGE_CURVE ( 'NONE', #3728, #25822, #1319, .T. ) ;
#19032=ORIENTED_EDGE ( 'NONE', *, *, #20072, .T. ) ;
#19034=CARTESIAN_POINT ( 'NONE',  ( 57.01079425239058196, -0.7499991164627679563, -1.746008812021272227 ) ) ;
#19035=CARTESIAN_POINT ( 'NONE',  ( 57.05000000000001847, 0.7500000000000000000, -2.421260002560649660 ) ) ;
#19039=PRESENTATION_STYLE_ASSIGNMENT (( #21580 ) ) ;
#19042=ORIENTED_EDGE ( 'NONE', *, *, #25179, .F. ) ;
#19045=ORIENTED_EDGE ( 'NONE', *, *, #23836, .T. ) ;
#19054=AXIS2_PLACEMENT_3D ( 'NONE', #17356, #27003, #14974 ) ;
#19058=DIRECTION ( 'NONE',  ( 1.000000000000000000, -0.000000000000000000, -0.000000000000000000 ) ) ;
#19060=CARTESIAN_POINT ( 'NONE',  ( 48.30000000000001847, 0.6462379109121000331, 4.048750000000023164 ) ) ;
#19061=CARTESIAN_POINT ( 'NONE',  ( 15.68751737981905592, 5.244794032782712279, -1.329291831544122005 ) ) ;
#19065=ORIENTED_EDGE ( 'NONE', *, *, #350, .F. ) ;
#19069=CIRCLE ( 'NONE', #4384, 3.625000000000028866 ) ;
#19076=ORIENTED_EDGE ( 'NONE', *, *, #17181, .T. ) ;
#19077=VECTOR ( 'NONE', #23805, 1000.000000000000000 ) ;
#19079=CARTESIAN_POINT ( 'NONE',  ( 15.03925126672122303, 4.683225679163316890, 2.703237727951268710 ) ) ;
#19081=VECTOR ( 'NONE', #27043, 1000.000000000000000 ) ;
#19084=EDGE_LOOP ( 'NONE', ( #25252, #14156, #4650, #14772 ) ) ;
#19086=CIRCLE ( 'NONE', #5917, 5.407411300779133789 ) ;
#19087=VECTOR ( 'NONE', #7060, 1000.000000000000000 ) ;
#19089=DIRECTION ( 'NONE',  ( 0.000000000000000000, -1.000000000000000000, 0.000000000000000000 ) ) ;
#19090=ORIENTED_EDGE ( 'NONE', *, *, #27756, .T. ) ;
#19091=EDGE_CURVE ( 'NONE', #24584, #29689, #16615, .T. ) ;
#19092=CARTESIAN_POINT ( 'NONE',  ( -35.85663232820583346, -3.817150320980684075, 2.203324261490539282 ) ) ;
#19094=CARTESIAN_POINT ( 'NONE',  ( 15.03925126672132961, -3.426725943139530717, -3.937891353488757851 ) ) ;
#19101=DIRECTION ( 'NONE',  ( 0.000000000000000000, 0.000000000000000000, 1.000000000000000000 ) ) ;
#19104=ADVANCED_FACE ( 'NONE', ( #3587 ), #29639, .T. ) ;
#19107=VECTOR ( 'NONE', #21852, 1000.000000000000000 ) ;
#19108=CARTESIAN_POINT ( 'NONE',  ( -54.44999999999997442, 0.000000000000000000, 0.000000000000000000 ) ) ;
#19112=VERTEX_POINT ( 'NONE', #27650 ) ;
#19113=EDGE_CURVE ( 'NONE', #27607, #3125, #7896, .T. ) ;
#19116=EDGE_CURVE ( 'NONE', #27954, #21791, #31165, .T. ) ;
#19119=CARTESIAN_POINT ( 'NONE',  ( 48.50000000000002132, 1.391941090707534023, 3.750000000000022649 ) ) ;
#19122=ORIENTED_EDGE ( 'NONE', *, *, #19942, .T. ) ;
#19124=CYLINDRICAL_SURFACE ( 'NONE', #14882, 0.7500000000000001110 ) ;
#19126=ORIENTED_EDGE ( 'NONE', *, *, #24118, .T. ) ;
#19130=CARTESIAN_POINT ( 'NONE',  ( -36.92405921417682890, 5.187083072802322725, 1.534568794951225001 ) ) ;
#19148=CARTESIAN_POINT ( 'NONE',  ( 51.80000000000001847, 1.734723475976807094E-15, 0.000000000000000000 ) ) ;
#19150=VERTEX_POINT ( 'NONE', #24801 ) ;
#19156=ORIENTED_EDGE ( 'NONE', *, *, #5485, .T. ) ;
#19157=EDGE_CURVE ( 'NONE', #26099, #19552, #27111, .T. ) ;
#19158=CARTESIAN_POINT ( 'NONE',  ( 15.17214319754860696, 0.4576450703117014296, -5.200000005133889047 ) ) ;
#19160=DIRECTION ( 'NONE',  ( -0.000000000000000000, 1.000000000000000000, 1.532429380227459806E-15 ) ) ;
#19164=DIRECTION ( 'NONE',  ( 0.000000000000000000, 1.000000000000000000, 0.000000000000000000 ) ) ;
#19165=CARTESIAN_POINT ( 'NONE',  ( -54.44999999999997442, 1.499999999999999556, 3.300094695611021756 ) ) ;
#19168=ORIENTED_EDGE ( 'NONE', *, *, #2688, .F. ) ;
#19173=CARTESIAN_POINT ( 'NONE',  ( -44.49999999999997868, 0.000000000000000000, 2.168404344971008868E-14 ) ) ;
#19175=( BOUNDED_SURFACE ( )  B_SPLINE_SURFACE ( 3, 2, ( 
 ( #19694, #12235, #26182 ),
 ( #56, #14294, #5109 ),
 ( #9719, #21919, #4788 ),
 ( #9573, #14610, #11922 ),
 ( #16693, #7330, #2104 ),
 ( #2431, #16525, #14446 ),
 ( #19231, #7496, #17001 ),
 ( #19535, #2257, #21443 ),
 ( #12091, #23963, #21769 ),
 ( #28872, #24420, #31249 ) ),
 .UNSPECIFIED., .F., .F., .F. ) 
 B_SPLINE_SURFACE_WITH_KNOTS ( ( 4, 2, 2, 2, 4 ),
 ( 3, 3 ),
 ( 0.0002526260074104870901, 0.0003606909493797115550, 0.0004687558913489359657, 0.0006848857752873848412, 0.001117145543164282592 ),
 ( 0.000000000000000000, 1.000000000000000000 ),
 .UNSPECIFIED. ) 
 GEOMETRIC_REPRESENTATION_ITEM ( )  RATIONAL_B_SPLINE_SURFACE ( (
 ( 1.000000000000000000, 0.9842509842511785179, 1.000000000000000000),
 ( 1.000000000000000000, 0.9838268088398656186, 1.000000000000000000),
 ( 1.000000000000000000, 0.9731519947952637084, 1.000000000000000000),
 ( 1.000000000000000000, 0.9499473078865111608, 1.000000000000000000),
 ( 1.000000000000000000, 0.9371632344323036490, 1.000000000000000000),
 ( 1.000000000000000000, 0.8981767195496310752, 1.000000000000000000),
 ( 1.000000000000000000, 0.8714317066438556081, 1.000000000000000000),
 ( 1.000000000000000000, 0.7945716934681391619, 1.000000000000000000),
 ( 1.000000000000000000, 0.7462340517456872435, 1.000000000000000000),
 ( 1.000000000000000000, 0.7071067811865260344, 1.000000000000000000) ) ) 
 REPRESENTATION_ITEM ( '' )  SURFACE ( )  );
#19179=CARTESIAN_POINT ( 'NONE',  ( 57.01256279823148532, -0.7331429619035759737, 1.793127402884417965 ) ) ;
#19180=CARTESIAN_POINT ( 'NONE',  ( 16.10705563471231017, -3.051830235922889489, 4.466755975380364063 ) ) ;
#19185=CARTESIAN_POINT ( 'NONE',  ( 57.00500393873097238, -0.7225500701544015358, -2.438740121660158078 ) ) ;
#19186=FACE_OUTER_BOUND ( 'NONE', #24726, .T. ) ;
#19187=CARTESIAN_POINT ( 'NONE',  ( -35.85663232820584057, 1.793057972834756431, 4.026191436120398315 ) ) ;
#19193=AXIS2_PLACEMENT_3D ( 'NONE', #1778, #8455, #25391 ) ;
#19197=CARTESIAN_POINT ( 'NONE',  ( -36.27260443516981780, 5.005099703116275833, 1.423440526322142574 ) ) ;
#19198=CARTESIAN_POINT ( 'NONE',  ( 15.41586008885037806, -4.863061488092547791, 1.860589201779584867 ) ) ;
#19201=DIRECTION ( 'NONE',  ( -1.000000000000000000, -0.000000000000000000, -0.000000000000000000 ) ) ;
#19202=ORIENTED_EDGE ( 'NONE', *, *, #17877, .F. ) ;
#19206=ORIENTED_EDGE ( 'NONE', *, *, #15827, .T. ) ;
#19207=CARTESIAN_POINT ( 'NONE',  ( 48.30000000000001847, 2.428612866367529932E-14, 0.000000000000000000 ) ) ;
#19208=EDGE_LOOP ( 'NONE', ( #17203, #9622, #3243, #4832 ) ) ;
#19222=LINE ( 'NONE', #8899, #14921 ) ;
#19225=CARTESIAN_POINT ( 'NONE',  ( 15.03925126672127632, 5.086913985776164715, -1.171642053949048856 ) ) ;
#19227=ORIENTED_EDGE ( 'NONE', *, *, #16750, .T. ) ;
#19228=CARTESIAN_POINT ( 'NONE',  ( 15.03925126672133139, -4.804073783693434407, -2.042134687550376526 ) ) ;
#19231=CARTESIAN_POINT ( 'NONE',  ( 48.41509867277373047, -1.114141714781589521, 3.896173399896524003 ) ) ;
#19232=CARTESIAN_POINT ( 'NONE',  ( 48.49162684147595570, -1.391941090707504269, -3.850000000000020517 ) ) ;
#19237=CIRCLE ( 'NONE', #7580, 0.05000000000000012768 ) ;
#19238=VERTEX_POINT ( 'NONE', #11315 ) ;
#19245=CIRCLE ( 'NONE', #8586, 0.04999999999999991257 ) ;
#19246=CARTESIAN_POINT ( 'NONE',  ( 48.40116939571130672, -0.8930800907915671383, 3.925677024646228475 ) ) ;
#19248=ORIENTED_EDGE ( 'NONE', *, *, #12393, .F. ) ;
#19257=ORIENTED_EDGE ( 'NONE', *, *, #18830, .F. ) ;
#19258=DIRECTION ( 'NONE',  ( 0.000000000000000000, 0.000000000000000000, -1.000000000000000000 ) ) ;
#19262=CARTESIAN_POINT ( 'NONE',  ( -36.42771574642715393, -2.777216423307978133, 4.646230875016813755 ) ) ;
#19270=EDGE_CURVE ( 'NONE', #15970, #15422, #6389, .T. ) ;
#19272=ORIENTED_EDGE ( 'NONE', *, *, #18081, .F. ) ;
#19275=LINE ( 'NONE', #2306, #10463 ) ;
#19277=VERTEX_POINT ( 'NONE', #4197 ) ;
#19278=ORIENTED_EDGE ( 'NONE', *, *, #9830, .T. ) ;
#19279=DIRECTION ( 'NONE',  ( 0.000000000000000000, 0.000000000000000000, 1.000000000000000000 ) ) ;
#19283=CARTESIAN_POINT ( 'NONE',  ( 50.40000000000001279, 0.7707709757764751313, 3.938803467580343831 ) ) ;
#19287=CARTESIAN_POINT ( 'NONE',  ( 57.01635142493560693, 0.7373792903891465134, 1.789496335369930025 ) ) ;
#19292=EDGE_CURVE ( 'NONE', #20389, #28184, #23088, .T. ) ;
#19293=CARTESIAN_POINT ( 'NONE',  ( 48.40000000000001990, 1.391941090707534245, 3.850000000000022737 ) ) ;
#19297=AXIS2_PLACEMENT_3D ( 'NONE', #13087, #22613, #22773 ) ;
#19298=CARTESIAN_POINT ( 'NONE',  ( -36.92405921417685732, 0.1434351685890311867, 5.407416993630365987 ) ) ;
#19301=CARTESIAN_POINT ( 'NONE',  ( -54.49181037333889321, 1.522049374736507144, 3.314263409011526385 ) ) ;
#19303=VERTEX_POINT ( 'NONE', #16095 ) ;
#19305=CARTESIAN_POINT ( 'NONE',  ( -54.48478889579405404, 1.513794642953540270, 4.039462313877656641 ) ) ;
#19306=EDGE_LOOP ( 'NONE', ( #26920, #8622, #24144, #2315 ) ) ;
#19310=EDGE_LOOP ( 'NONE', ( #30346, #6057, #4139, #18187 ) ) ;
#19311=DIRECTION ( 'NONE',  ( 0.000000000000000000, 0.000000000000000000, 1.000000000000000000 ) ) ;
#19318=CARTESIAN_POINT ( 'NONE',  ( 47.04570146981701129, -4.276948333784440059, -0.9210526315789477891 ) ) ;
#19320=CARTESIAN_POINT ( 'NONE',  ( 15.59055531549693718, -3.917775493694396260, -3.727542820438248583 ) ) ;
#19324=CARTESIAN_POINT ( 'NONE',  ( 58.45000000000001705, 0.8000000000000000444, 2.421260002560649660 ) ) ;
#19328=CARTESIAN_POINT ( 'NONE',  ( 15.68751737981906302, -3.461789369942958050, 4.158232265984262988 ) ) ;
#19329=ADVANCED_FACE ( 'NONE', ( #18314 ), #5557, .T. ) ;
#19330=CARTESIAN_POINT ( 'NONE',  ( 48.46374521131294699, 1.419210040599422795, -3.846553521706499446 ) ) ;
#19339=DIRECTION ( 'NONE',  ( 0.000000000000000000, 1.000000000000000000, 0.000000000000000000 ) ) ;
#19340=ORIENTED_EDGE ( 'NONE', *, *, #24213, .F. ) ;
#19346=CYLINDRICAL_SURFACE ( 'NONE', #27775, 0.05000000000000143219 ) ;
#19347=DIRECTION ( 'NONE',  ( 1.000000000000000000, 5.570239943078649173E-15, -9.650165233620068940E-15 ) ) ;
#19368=DIRECTION ( 'NONE',  ( 0.000000000000000000, 0.000000000000000000, 1.000000000000000000 ) ) ;
#19371=CIRCLE ( 'NONE', #25424, 0.04999999999999991257 ) ;
#19372=CARTESIAN_POINT ( 'NONE',  ( 48.48434962373865886, 1.386108502191577108, -3.851082811767820413 ) ) ;
#19373=CARTESIAN_POINT ( 'NONE',  ( 54.40000000000001990, 1.029992063861229212E-15, -4.375000000000002665 ) ) ;
#19378=CARTESIAN_POINT ( 'NONE',  ( 56.95000000000001705, 0.000000000000000000, 0.000000000000000000 ) ) ;
#19381=ORIENTED_EDGE ( 'NONE', *, *, #18597, .T. ) ;
#19383=ORIENTED_EDGE ( 'NONE', *, *, #21151, .F. ) ;
#19387=VERTEX_POINT ( 'NONE', #7948 ) ;
#19389=CARTESIAN_POINT ( 'NONE',  ( 15.66436536804550883, 5.008501212420992665, 2.048848402342041908 ) ) ;
#19392=CARTESIAN_POINT ( 'NONE',  ( 48.41298237836545582, -1.088467210617550807, 3.899823238510139678 ) ) ;
#19395=CARTESIAN_POINT ( 'NONE',  ( 54.40000000000001990, -1.084202172485504434E-16, 4.374999999999999112 ) ) ;
#19400=DIRECTION ( 'NONE',  ( 0.000000000000000000, -0.9615843008030765526, -0.2745098039215693730 ) ) ;
#19404=DIRECTION ( 'NONE',  ( 0.000000000000000000, 0.000000000000000000, -1.000000000000000000 ) ) ;
#19405=EDGE_CURVE ( 'NONE', #16179, #10988, #17445, .T. ) ;
#19406=CARTESIAN_POINT ( 'NONE',  ( -36.30424252565905618, -3.146183597690385803, 4.141717300434374138 ) ) ;
#19413=VECTOR ( 'NONE', #10485, 1000.000000000000000 ) ;
#19415=CARTESIAN_POINT ( 'NONE',  ( 51.88138499675474691, 0.02607891777379810205, -4.373234472033241893 ) ) ;
#19422=ORIENTED_EDGE ( 'NONE', *, *, #6943, .T. ) ;
#19424=VERTEX_POINT ( 'NONE', #194 ) ;
#19433=CARTESIAN_POINT ( 'NONE',  ( 57.02114622761336449, 0.7499999999999982236, -1.778341845356538498 ) ) ;
#19439=CARTESIAN_POINT ( 'NONE',  ( -54.44999999999997442, -6.938893903907228378E-14, 0.000000000000000000 ) ) ;
#19440=CARTESIAN_POINT ( 'NONE',  ( 50.38693217303928407, 1.296871156637316114, -3.889656364559859192 ) ) ;
#19444=CARTESIAN_POINT ( 'NONE',  ( -54.44999999999997442, -1.499999999999999556, -4.029888335921975262 ) ) ;
#19446=CARTESIAN_POINT ( 'NONE',  ( -36.11187263677957304, -2.734387802834445047, -4.440904455451657462 ) ) ;
#19454=CARTESIAN_POINT ( 'NONE',  ( -36.50489844130355266, -5.024465639092029257, 2.007392901578141320 ) ) ;
#19460=DIRECTION ( 'NONE',  ( 0.000000000000000000, 0.000000000000000000, -1.000000000000000000 ) ) ;
#19462=CARTESIAN_POINT ( 'NONE',  ( -54.48118151432741030, -1.510613940323803916, -4.037256667234632168 ) ) ;
#19470=DIRECTION ( 'NONE',  ( -1.000000000000000000, 0.000000000000000000, 0.000000000000000000 ) ) ;
#19473=ORIENTED_EDGE ( 'NONE', *, *, #19916, .T. ) ;
#19478=CARTESIAN_POINT ( 'NONE',  ( 58.45000000000001705, 0.8000000000000000444, -1.778341924377873751 ) ) ;
#19479=VECTOR ( 'NONE', #14585, 1000.000000000000000 ) ;
#19480=DIRECTION ( 'NONE',  ( 0.000000000000000000, 1.000000000000000000, 0.000000000000000000 ) ) ;
#19488=CARTESIAN_POINT ( 'NONE',  ( 15.57907767661744991, -2.743848709681487197, -4.666930520580701014 ) ) ;
#19490=DIRECTION ( 'NONE',  ( -1.000000000000000000, -0.000000000000000000, -0.000000000000000000 ) ) ;
#19498=CARTESIAN_POINT ( 'NONE',  ( 51.70652201333279407, -4.179189514726790122, 0.9999999999996741495 ) ) ;
#19501=EDGE_LOOP ( 'NONE', ( #7962, #11074, #23789, #5433 ) ) ;
#19503=FACE_OUTER_BOUND ( 'NONE', #22663, .T. ) ;
#19505=( NAMED_UNIT ( * ) PLANE_ANGLE_UNIT ( ) SI_UNIT ( $, .RADIAN. ) );
#19510=ORIENTED_EDGE ( 'NONE', *, *, #17724, .F. ) ;
#19511=ORIENTED_EDGE ( 'NONE', *, *, #6526, .T. ) ;
#19515=CARTESIAN_POINT ( 'NONE',  ( -54.49181037333889321, -1.522049374736507588, 3.314263409011525496 ) ) ;
#19516=TOROIDAL_SURFACE ( 'NONE', #22046, 4.000000000000022204, 0.1000000000000000056 ) ;
#19521=CARTESIAN_POINT ( 'NONE',  ( -36.68133364217572989, -0.7247683022691534527, -5.358970532132250497 ) ) ;
#19523=EDGE_CURVE ( 'NONE', #4176, #24464, #1126, .T. ) ;
#19524=CARTESIAN_POINT ( 'NONE',  ( 46.90000006803324339, -4.241636233590472926, 1.073352279313351865 ) ) ;
#19525=CARTESIAN_POINT ( 'NONE',  ( 15.03925126672132961, -4.018128179617543871, 3.618665901676652918 ) ) ;
#19527=CARTESIAN_POINT ( 'NONE',  ( 54.49989931805382071, -0.003076767800981534788, -4.280178505497699959 ) ) ;
#19531=CARTESIAN_POINT ( 'NONE',  ( 33.47623932017462778, 5.407411300779134677, 0.000000000000000000 ) ) ;
#19535=CARTESIAN_POINT ( 'NONE',  ( 48.40134283869316789, -0.9106118309512859499, 3.923752762110600312 ) ) ;
#19540=VECTOR ( 'NONE', #23570, 1000.000000000000000 ) ;
#19541=ORIENTED_EDGE ( 'NONE', *, *, #23961, .T. ) ;
#19552=VERTEX_POINT ( 'NONE', #812 ) ;
#19558=TOROIDAL_SURFACE ( 'NONE', #7912, 1.949999999999999956, 0.05000000000000000278 ) ;
#19562=CARTESIAN_POINT ( 'NONE',  ( -54.49853245345825314, -1.536420219664552445, 4.055116445457032981 ) ) ;
#19566=CONICAL_SURFACE ( 'NONE', #20137, 5.407411300779140895, 0.1317529408396977408 ) ;
#19567=CARTESIAN_POINT ( 'NONE',  ( -35.85663232820583346, 4.383220986680242071, -0.4611378927884229317 ) ) ;
#19572=AXIS2_PLACEMENT_3D ( 'NONE', #19378, #7183, #29181 ) ;
#19579=CIRCLE ( 'NONE', #2363, 30.00000000000000355 ) ;
#19580=ORIENTED_EDGE ( 'NONE', *, *, #5592, .T. ) ;
#19581=ORIENTED_EDGE ( 'NONE', *, *, #6648, .T. ) ;
#19582=CIRCLE ( 'NONE', #1359, 0.09999999999999982514 ) ;
#19594=ORIENTED_EDGE ( 'NONE', *, *, #29980, .F. ) ;
#19599=CARTESIAN_POINT ( 'NONE',  ( 58.45000000000001705, 0.000000000000000000, 0.000000000000000000 ) ) ;
#19602=CARTESIAN_POINT ( 'NONE',  ( 15.39414421509785669, -4.855742670514252346, -1.883114206442395133 ) ) ;
#19608=AXIS2_PLACEMENT_3D ( 'NONE', #8442, #5922, #25848 ) ;
#19609=CARTESIAN_POINT ( 'NONE',  ( 50.45647961155643912, 1.212999249975939886, -3.917061424767716016 ) ) ;
#19613=ORIENTED_EDGE ( 'NONE', *, *, #1351, .T. ) ;
#19615=TOROIDAL_SURFACE ( 'NONE', #9518, 4.275000000000000355, 0.1000000000000000056 ) ;
#19616=CARTESIAN_POINT ( 'NONE',  ( -36.50489844130311212, -3.461789369942962047, -4.158232265984187492 ) ) ;
#19619=CIRCLE ( 'NONE', #30744, 0.05000000000000017625 ) ;
#19620=EDGE_LOOP ( 'NONE', ( #29884, #23226, #5542, #4564, #14317 ) ) ;
#19621=CARTESIAN_POINT ( 'NONE',  ( 15.95705409078464498, -0.6016956010317232595, -5.375730734456591442 ) ) ;
#19626=CIRCLE ( 'NONE', #7475, 5.407411300779133789 ) ;
#19627=EDGE_CURVE ( 'NONE', #2253, #12845, #17037, .T. ) ;
#19628=DIRECTION ( 'NONE',  ( 0.000000000000000000, 0.1576190026614809614, -0.9875000000000001554 ) ) ;
#19631=VERTEX_POINT ( 'NONE', #21092 ) ;
#19633=CARTESIAN_POINT ( 'NONE',  ( -35.85663232820584057, 2.686240680702099759, 4.475885388010746979 ) ) ;
#19634=CARTESIAN_POINT ( 'NONE',  ( 56.96706223141283942, -0.7377629956704406800, 1.750942290135934831 ) ) ;
#19638=CARTESIAN_POINT ( 'NONE',  ( 57.05000000000001847, -0.7500000000000000000, -2.421260002560649660 ) ) ;
#19642=CARTESIAN_POINT ( 'NONE',  ( 16.07279755198632287, -3.436881753486524360, 4.177093996075195825 ) ) ;
#19643=DIRECTION ( 'NONE',  ( 1.000000000000000000, 0.000000000000000000, 0.000000000000000000 ) ) ;
#19646=CARTESIAN_POINT ( 'NONE',  ( -54.49999999999997868, -1.549999999999999600, -3.332135201338624952 ) ) ;
#19647=B_SPLINE_CURVE_WITH_KNOTS ( 'NONE', 3,
 ( #21234, #19318, #21535, #16931, #7122, #14070 ),
 .UNSPECIFIED., .F., .F.,
 ( 4, 2, 4 ),
 ( 0.000000000000000000, 0.0001620412083492963143, 0.0003240824166985928996 ),
 .UNSPECIFIED. ) ;
#19650=CARTESIAN_POINT ( 'NONE',  ( 50.39883060428874018, -0.8930800907915671383, -3.925677024646228475 ) ) ;
#19659=AXIS2_PLACEMENT_3D ( 'NONE', #5372, #22183, #469 ) ;
#19665=CARTESIAN_POINT ( 'NONE',  ( 57.00000000000001421, -0.6820512820512794061, -1.773360101234991326 ) ) ;
#19667=CARTESIAN_POINT ( 'NONE',  ( -36.58413561666647951, -5.110933801299883505, -1.769007076670894740 ) ) ;
#19676=CARTESIAN_POINT ( 'NONE',  ( -54.49999477219272848, -1.549165129012789688, 3.331602747802265174 ) ) ;
#19678=CARTESIAN_POINT ( 'NONE',  ( 15.03925126672132961, 3.275050215668611653, -2.949461045527567382 ) ) ;
#19680=EDGE_CURVE ( 'NONE', #23625, #11505, #4444, .T. ) ;
#19682=CARTESIAN_POINT ( 'NONE',  ( -36.31440869660544735, 0.05469410396133651819, -5.200000001157072838 ) ) ;
#19685=EDGE_CURVE ( 'NONE', #25246, #28315, #21559, .T. ) ;
#19687=CARTESIAN_POINT ( 'NONE',  ( -35.85663232820583346, -5.377732432866661583, 0.5657657256215455899 ) ) ;
#19688=CARTESIAN_POINT ( 'NONE',  ( 15.61552784268242178, 4.977698683490556775, -2.127480166903953585 ) ) ;
#19691=LINE ( 'NONE', #14291, #24052 ) ;
#19694=CARTESIAN_POINT ( 'NONE',  ( 48.50000000000178346, -1.391941090720833607, 3.849999999997240074 ) ) ;
#19698=DIRECTION ( 'NONE',  ( -1.000000000000000000, -2.586136946169074517E-16, 0.000000000000000000 ) ) ;
#19700=ORIENTED_EDGE ( 'NONE', *, *, #18494, .F. ) ;
#19716=CARTESIAN_POINT ( 'NONE',  ( 51.79898443072417535, -4.139722501993201575, -1.083525984490930183 ) ) ;
#19717=EDGE_CURVE ( 'NONE', #1490, #21976, #5202, .T. ) ;
#19718=CARTESIAN_POINT ( 'NONE',  ( -54.46895629856896903, -1.503487923075246480, 4.032311158269683560 ) ) ;
#19720=DIRECTION ( 'NONE',  ( 0.000000000000000000, 0.000000000000000000, -1.000000000000000000 ) ) ;
#19721=CARTESIAN_POINT ( 'NONE',  ( 57.01182421275571954, 0.7322894606377696736, 2.432677346698721266 ) ) ;
#19725=EDGE_CURVE ( 'NONE', #4123, #27607, #16017, .T. ) ;
#19729=CARTESIAN_POINT ( 'NONE',  ( 51.75857864376271777, -3.767600426651517953, 1.000000000000000222 ) ) ;
#19730=VECTOR ( 'NONE', #30375, 1000.000000000000000 ) ;
#19734=VECTOR ( 'NONE', #26350, 1000.000000000000000 ) ;
#19740=CARTESIAN_POINT ( 'NONE',  ( -36.11780688638206982, 2.199885882962476114, 4.939696253590518005 ) ) ;
#19741=ORIENTED_EDGE ( 'NONE', *, *, #21672, .F. ) ;
#19746=EDGE_LOOP ( 'NONE', ( #11118, #20642, #19272, #1293 ) ) ;
#19752=ADVANCED_FACE ( 'NONE', ( #5212 ), #21724, .T. ) ;
#19753=CARTESIAN_POINT ( 'NONE',  ( 15.66436536804540403, -5.008501212420952697, -2.048848402342096087 ) ) ;
#19759=CARTESIAN_POINT ( 'NONE',  ( -35.85663232820580504, -3.779372838781780430, -3.883777296072560947 ) ) ;
#19763=CARTESIAN_POINT ( 'NONE',  ( -36.77443515226830328, -2.672993279333732541, -4.702725322014769560 ) ) ;
#19766=CARTESIAN_POINT ( 'NONE',  ( 50.49739899587714831, 0.9326869175216770946, -3.995127421239667687 ) ) ;
#19769=CARTESIAN_POINT ( 'NONE',  ( -36.25997906085252254, -4.878092280899822164, 1.814329181850224071 ) ) ;
#19771=DIRECTION ( 'NONE',  ( 0.000000000000000000, 0.000000000000000000, 1.000000000000000000 ) ) ;
#19776=CARTESIAN_POINT ( 'NONE',  ( 33.47623932017462778, -4.683225679163332877, -2.703237727951242508 ) ) ;
#19777=PLANE ( 'NONE',  #5849 ) ;
#19779=CARTESIAN_POINT ( 'NONE',  ( 57.01359174706111332, -0.7734660154240907692, 1.735448526467797459 ) ) ;
#19788=CARTESIAN_POINT ( 'NONE',  ( 15.03925126672125678, -3.779372838781788868, 3.883777296072539187 ) ) ;
#19789=CYLINDRICAL_SURFACE ( 'NONE', #8381, 0.7500000000000001110 ) ;
#19812=ORIENTED_EDGE ( 'NONE', *, *, #19405, .F. ) ;
#19820=CARTESIAN_POINT ( 'NONE',  ( 48.50000000000002132, -1.409901620910170461, -3.850000000000021849 ) ) ;
#19821=DIRECTION ( 'NONE',  ( 0.000000000000000000, 0.000000000000000000, -1.000000000000000000 ) ) ;
#19822=CARTESIAN_POINT ( 'NONE',  ( 51.90000000000001279, -4.227689052994015206, -1.125730994152047693 ) ) ;
#19825=VECTOR ( 'NONE', #23688, 1000.000000000000000 ) ;
#19829=CARTESIAN_POINT ( 'NONE',  ( -35.85663232820580504, -0.7747498368337907282, -5.363501452440941009 ) ) ;
#19834=LINE ( 'NONE', #3354, #17974 ) ;
#19838=CARTESIAN_POINT ( 'NONE',  ( 57.00873807961998097, 0.7491996424029042645, 2.489992076190610248 ) ) ;
#19839=VERTEX_POINT ( 'NONE', #23875 ) ;
#19845=CARTESIAN_POINT ( 'NONE',  ( 16.08093158123428523, 5.226279933021939605, -1.394410282272748880 ) ) ;
#19847=B_SPLINE_CURVE_WITH_KNOTS ( 'NONE', 3,
 ( #13770, #18722, #28208, #11415, #16009, #25825, #25672, #1924, #21413, #9365, #11587, #30742, #30899, #25977 ),
 .UNSPECIFIED., .F., .F.,
 ( 4, 2, 2, 2, 2, 2, 4 ),
 ( 0.000000000000000000, 0.0003953907277084696219, 0.0005930860915627040805, 0.0006919337734898216080, 0.0007413576144533806428, 0.0007660695349351557149, 0.0007907814554169307871 ),
 .UNSPECIFIED. ) ;
#19848=CARTESIAN_POINT ( 'NONE',  ( 46.90000000000001279, -4.227689052994015206, 1.125730994152046582 ) ) ;
#19852=CARTESIAN_POINT ( 'NONE',  ( 54.47883572522132312, -0.001215825626424074960, 4.337530305537235620 ) ) ;
#19855=EDGE_CURVE ( 'NONE', #30058, #27746, #6614, .T. ) ;
#19856=PLANE ( 'NONE',  #14377 ) ;
#19858=CARTESIAN_POINT ( 'NONE',  ( 51.77013903953137230, -4.166824046520646974, -1.027859347733066420 ) ) ;
#19861=DIRECTION ( 'NONE',  ( -1.000000000000000000, -0.000000000000000000, -0.000000000000000000 ) ) ;
#19863=FACE_OUTER_BOUND ( 'NONE', #17657, .T. ) ;
#19864=CARTESIAN_POINT ( 'NONE',  ( 57.03008957414009217, 0.7461961634598838211, 2.423767181580114727 ) ) ;
#19870=CARTESIAN_POINT ( 'NONE',  ( -54.49999477219272848, 1.549165129012789466, -3.331602747802265174 ) ) ;
#19879=CARTESIAN_POINT ( 'NONE',  ( 15.71019289815286513, 4.797343084509189559, 2.497389432264014886 ) ) ;
#19881=ORIENTED_EDGE ( 'NONE', *, *, #12606, .T. ) ;
#19886=EDGE_CURVE ( 'NONE', #8533, #7645, #30157, .T. ) ;
#19891=DIRECTION ( 'NONE',  ( 0.000000000000000000, 0.000000000000000000, 1.000000000000000000 ) ) ;
#19892=EDGE_CURVE ( 'NONE', #5273, #13582, #4481, .T. ) ;
#19899=CARTESIAN_POINT ( 'NONE',  ( 48.30268969835653081, 0.9327905306641951499, -3.995066436131523346 ) ) ;
#19900=FACE_OUTER_BOUND ( 'NONE', #27383, .T. ) ;
#19902=VECTOR ( 'NONE', #467, 1000.000000000000000 ) ;
#19907=ORIENTED_EDGE ( 'NONE', *, *, #23961, .F. ) ;
#19910=DIRECTION ( 'NONE',  ( 0.000000000000000000, -0.000000000000000000, -1.000000000000000000 ) ) ;
#19913=DIRECTION ( 'NONE',  ( 0.000000000000000000, 1.000000000000000000, 0.000000000000000000 ) ) ;
#19916=EDGE_CURVE ( 'NONE', #3969, #9980, #7927, .T. ) ;
#19918=DIRECTION ( 'NONE',  ( 1.000000000000000000, 3.125586771759065906E-16, 0.000000000000000000 ) ) ;
#19919=CARTESIAN_POINT ( 'NONE',  ( 48.39253357792949117, -1.341874354110733858, -3.874311046529112623 ) ) ;
#19923=CARTESIAN_POINT ( 'NONE',  ( 48.30000000000001847, -0.6304760106459033064, 3.950000000000021938 ) ) ;
#19927=ORIENTED_EDGE ( 'NONE', *, *, #19886, .T. ) ;
#19930=CARTESIAN_POINT ( 'NONE',  ( 57.04071222441830713, -0.7791709056946051204, 1.732885792771923672 ) ) ;
#19938=CARTESIAN_POINT ( 'NONE',  ( 15.74652664997094931, 3.345968172200292745, 4.250076229745635814 ) ) ;
#19942=EDGE_CURVE ( 'NONE', #7645, #9785, #30291, .T. ) ;
#19947=EDGE_LOOP ( 'NONE', ( #8377, #17925, #19381, #28300 ) ) ;
#19952=CARTESIAN_POINT ( 'NONE',  ( 15.48686146417451148, -3.146183597690412448, -4.141717300434339499 ) ) ;
#19953=CARTESIAN_POINT ( 'NONE',  ( 33.47623932017462778, 1.734723475976807489E-15, 0.000000000000000000 ) ) ;
#19954=ORIENTED_EDGE ( 'NONE', *, *, #7271, .T. ) ;
#19962=CIRCLE ( 'NONE', #24999, 0.4576450603546982632 ) ;
#19963=DIRECTION ( 'NONE',  ( 2.459562394685749209E-16, -0.9510565162951544194, 0.3090169943749447312 ) ) ;
#19967=ORIENTED_EDGE ( 'NONE', *, *, #14341, .F. ) ;
#19972=CARTESIAN_POINT ( 'NONE',  ( 15.49702763512084047, 0.05469410396135616914, 5.200000001156997342 ) ) ;
#19976=CARTESIAN_POINT ( 'NONE',  ( -36.30347965937283305, -0.1138661108242699921, -5.199999999057708600 ) ) ;
#19979=CARTESIAN_POINT ( 'NONE',  ( 48.41845806530710661, 1.153441674035750708, -3.890342980189691158 ) ) ;
#19980=CARTESIAN_POINT ( 'NONE',  ( 15.48686146417449194, 4.911231426340504136, -1.712337380313421198 ) ) ;
#19981=CARTESIAN_POINT ( 'NONE',  ( 57.00000000000001421, -0.6999999999999999556, 2.452039967047845437 ) ) ;
#19994=DIRECTION ( 'NONE',  ( 0.000000000000000000, 0.000000000000000000, -1.000000000000000000 ) ) ;
#19998=CARTESIAN_POINT ( 'NONE',  ( 15.29449157529475301, 5.068523420888873865, 1.228242390833590658 ) ) ;
#20010=ORIENTED_EDGE ( 'NONE', *, *, #19855, .F. ) ;
#20012=CARTESIAN_POINT ( 'NONE',  ( 36.50000000000002132, 0.000000000000000000, 0.000000000000000000 ) ) ;
#20014=DIRECTION ( 'NONE',  ( -1.983166172879301074E-16, 0.9119702176296790030, -0.4102564102564101312 ) ) ;
#20015=CARTESIAN_POINT ( 'NONE',  ( -35.85663232820584057, -3.275050215668596998, 2.949461045527599801 ) ) ;
#20018=CARTESIAN_POINT ( 'NONE',  ( 57.02405634237670284, -0.7430569499193692140, 2.425812863566016997 ) ) ;
#20022=DIRECTION ( 'NONE',  ( 1.000000000000000000, 0.000000000000000000, 0.000000000000000000 ) ) ;
#20025=EDGE_CURVE ( 'NONE', #19387, #13619, #9883, .T. ) ;
#20026=CARTESIAN_POINT ( 'NONE',  ( -54.47366401599046526, 1.505709097230404359, -3.303769268891089794 ) ) ;
#20030=CARTESIAN_POINT ( 'NONE',  ( -54.49999999999997868, 1.549999999999999600, 3.332135201338624952 ) ) ;
#20032=B_SPLINE_CURVE_WITH_KNOTS ( 'NONE', 3,
 ( #5339, #290, #19930, #2985, #9959, #19779, #29415, #24672, #17868, #754, #19634, #15321, #10582, #20258, #10260, #598 ),
 .UNSPECIFIED., .F., .F.,
 ( 4, 3, 3, 3, 3, 4 ),
 ( 0.000000000000000000, 1.391268354954338704E-05, 4.880039988305115829E-05, 8.637315450940535953E-05, 0.0001246458323646918982, 0.0001626605312951481396 ),
 .UNSPECIFIED. ) ;
#20033=AXIS2_PLACEMENT_3D ( 'NONE', #1907, #30723, #21397 ) ;
#20034=ORIENTED_EDGE ( 'NONE', *, *, #19627, .F. ) ;
#20035=ORIENTED_EDGE ( 'NONE', *, *, #10892, .F. ) ;
#20038=CARTESIAN_POINT ( 'NONE',  ( 15.32766723174652768, 4.698774973472825245, 2.676767126782138462 ) ) ;
#20045=AXIS2_PLACEMENT_3D ( 'NONE', #10517, #8440, #20490 ) ;
#20046=B_SPLINE_CURVE_WITH_KNOTS ( 'NONE', 3,
 ( #14442, #12531, #19527, #27091, #29012, #2582, #14898, #15068, #24724, #2881, #3036, #12086, #12681, #22361, #21762, #7490, #50, #9713, #19373 ),
 .UNSPECIFIED., .F., .F.,
 ( 4, 3, 3, 3, 3, 3, 4 ),
 ( -7.770771407263729990E-06, 0.000000000000000000, 1.441088071712340062E-05, 4.839392028739892171E-05, 8.235972512776415120E-05, 0.0001163176750529216742, 0.0001502761185964958737 ),
 .UNSPECIFIED. ) ;
#20049=EDGE_CURVE ( 'NONE', #31043, #16826, #31115, .T. ) ;
#20055=DIRECTION ( 'NONE',  ( 0.000000000000000000, 0.000000000000000000, -1.000000000000000000 ) ) ;
#20058=CARTESIAN_POINT ( 'NONE',  ( 15.76623786017542628, -5.109611055794812451, -1.772889539330472441 ) ) ;
#20063=CARTESIAN_POINT ( 'NONE',  ( 51.90000000000001279, -4.241634596362392706, -1.073358427932568526 ) ) ;
#20067=CARTESIAN_POINT ( 'NONE',  ( -36.63359589171324870, -3.777141534544250501, -3.869853550719763557 ) ) ;
#20070=AXIS2_PLACEMENT_3D ( 'NONE', #26859, #12753, #22757 ) ;
#20072=EDGE_CURVE ( 'NONE', #15120, #7615, #2791, .T. ) ;
#20073=DIRECTION ( 'NONE',  ( 1.000000000000000000, 0.000000000000000000, 0.000000000000000000 ) ) ;
#20074=EDGE_CURVE ( 'NONE', #2309, #26302, #16521, .T. ) ;
#20077=CARTESIAN_POINT ( 'NONE',  ( -36.56242893520730064, -3.350344226587728791, -4.246692235172065288 ) ) ;
#20081=ORIENTED_EDGE ( 'NONE', *, *, #23601, .T. ) ;
#20087=ORIENTED_EDGE ( 'NONE', *, *, #19725, .T. ) ;
#20095=CARTESIAN_POINT ( 'NONE',  ( -54.49409853110120139, -1.525884777627348088, -4.047834655405394777 ) ) ;
#20106=ADVANCED_FACE ( 'NONE', ( #31069 ), #15441, .T. ) ;
#20107=ORIENTED_EDGE ( 'NONE', *, *, #31173, .T. ) ;
#20109=CARTESIAN_POINT ( 'NONE',  ( 15.29954477411524749, 2.199885872770226403, 4.939696258129626649 ) ) ;
#20116=EDGE_CURVE ( 'NONE', #22540, #5072, #30609, .T. ) ;
#20117=CARTESIAN_POINT ( 'NONE',  ( -35.98952425903316765, 4.804073785499212157, -2.042134698606532517 ) ) ;
#20118=CARTESIAN_POINT ( 'NONE',  ( -36.11692583559979397, 1.123735554575555406, 5.289358692618281843 ) ) ;
#20119=CARTESIAN_POINT ( 'NONE',  ( 48.41280093284954944, 1.295960864328840279, -3.889961360030776749 ) ) ;
#20128=DIRECTION ( 'NONE',  ( 0.000000000000000000, 0.000000000000000000, 1.000000000000000000 ) ) ;
#20135=CARTESIAN_POINT ( 'NONE',  ( 51.78448386883093235, -4.158727452193214269, 1.045216533296355665 ) ) ;
#20137=AXIS2_PLACEMENT_3D ( 'NONE', #3176, #8549, #641 ) ;
#20140=AXIS2_PLACEMENT_3D ( 'NONE', #26023, #21788, #4334 ) ;
#20145=EDGE_CURVE ( 'NONE', #20943, #3021, #27062, .T. ) ;
#20151=CARTESIAN_POINT ( 'NONE',  ( 33.47623932017462778, -5.377732432866642043, -0.5657657256215583574 ) ) ;
#20154=AXIS2_PLACEMENT_3D ( 'NONE', #1972, #28738, #14465 ) ;
#20160=CARTESIAN_POINT ( 'NONE',  ( 50.35370852371426764, -1.309359793766436519, -3.864871860988134955 ) ) ;
#20162=CARTESIAN_POINT ( 'NONE',  ( 15.56274145962646571, 3.953287617511378471, -3.694739123711352047 ) ) ;
#20165=VERTEX_POINT ( 'NONE', #4955 ) ;
#20169=CARTESIAN_POINT ( 'NONE',  ( 15.32752150720754436, -4.698781674909509931, 2.676750094560135906 ) ) ;
#20170=ORIENTED_EDGE ( 'NONE', *, *, #11832, .F. ) ;
#20172=CARTESIAN_POINT ( 'NONE',  ( 15.71019289815286513, 5.349060760730924180, -0.7993770229878035538 ) ) ;
#20179=ORIENTED_EDGE ( 'NONE', *, *, #9608, .F. ) ;
#20180=CARTESIAN_POINT ( 'NONE',  ( 57.03612573316699041, 0.7785448249619018046, -1.733167030474859205 ) ) ;
#20181=LINE ( 'NONE', #15397, #15719 ) ;
#20184=VERTEX_POINT ( 'NONE', #19228 ) ;
#20186=EDGE_CURVE ( 'NONE', #20985, #8353, #25550, .T. ) ;
#20187=CIRCLE ( 'NONE', #23224, 1.000000000000000000 ) ;
#20196=B_SPLINE_CURVE_WITH_KNOTS ( 'NONE', 3,
 ( #28496, #6649, #9191, #2202, #6800, #26117, #19179, #31021, #30537, #8844, #28182, #16153, #25804, #4111, #13750, #1720, #11389, #30719, #18695 ),
 .UNSPECIFIED., .F., .F.,
 ( 4, 3, 3, 3, 3, 3, 4 ),
 ( 0.000000000000000000, 2.270809125664990461E-05, 4.499850898804030560E-05, 6.557565265601914873E-05, 7.920624315363274039E-05, 8.325821076725717102E-05, 9.013793637923205450E-05 ),
 .UNSPECIFIED. ) ;
#20197=CARTESIAN_POINT ( 'NONE',  ( 50.50000000000002132, -0.6462379109120514054, -4.048750000000023164 ) ) ;
#20198=EDGE_CURVE ( 'NONE', #9408, #26742, #19691, .T. ) ;
#20200=CARTESIAN_POINT ( 'NONE',  ( 48.46374521131294699, -1.419210040599374612, 3.846553521706499001 ) ) ;
#20202=CARTESIAN_POINT ( 'NONE',  ( -54.49454330418567594, 1.526701536696945638, 3.317245250669464518 ) ) ;
#20214=EDGE_LOOP ( 'NONE', ( #8194, #17848, #829, #9493, #16766, #16387, #3485, #14830, #747, #12296 ) ) ;
#20215=DIRECTION ( 'NONE',  ( -0.000000000000000000, -1.000000000000000000, -0.000000000000000000 ) ) ;
#20223=CIRCLE ( 'NONE', #9077, 3.200000000000000178 ) ;
#20224=CARTESIAN_POINT ( 'NONE',  ( 15.41080140630285022, -4.895960019030861865, -2.323379425334049397 ) ) ;
#20229=CARTESIAN_POINT ( 'NONE',  ( 48.45869172792486523, 1.344780351710889610, 3.858600739747802599 ) ) ;
#20232=CIRCLE ( 'NONE', #11120, 1.850000000000000089 ) ;
#20234=PLANE ( 'NONE',  #24642 ) ;
#20241=ORIENTED_EDGE ( 'NONE', *, *, #7620, .F. ) ;
#20243=CARTESIAN_POINT ( 'NONE',  ( 15.61552784268253902, -0.4851603899461495728, -5.391500295856416436 ) ) ;
#20244=CARTESIAN_POINT ( 'NONE',  ( -36.23324115033480552, -5.027926281937912023, 1.353187539901980152 ) ) ;
#20245=DIRECTION ( 'NONE',  ( 1.000000000000000000, 0.000000000000000000, 0.000000000000000000 ) ) ;
#20251=DIRECTION ( 'NONE',  ( 0.000000000000000000, 0.000000000000000000, 1.000000000000000000 ) ) ;
#20252=EDGE_LOOP ( 'NONE', ( #26312, #9366, #19967, #21952 ) ) ;
#20258=CARTESIAN_POINT ( 'NONE',  ( 56.95220615073115056, -0.7055010433615873655, 1.764201441664152270 ) ) ;
#20259=FACE_OUTER_BOUND ( 'NONE', #20821, .T. ) ;
#20264=EDGE_CURVE ( 'NONE', #1297, #1993, #508, .T. ) ;
#20269=FACE_OUTER_BOUND ( 'NONE', #12123, .T. ) ;
#20271=DIRECTION ( 'NONE',  ( -1.000000000000000000, -0.000000000000000000, -0.000000000000000000 ) ) ;
#20274=CIRCLE ( 'NONE', #6610, 1.000000000000000000 ) ;
#20281=CARTESIAN_POINT ( 'NONE',  ( 15.03925126672132961, -3.426725943139531605, -3.937891353488756963 ) ) ;
#20292=LINE ( 'NONE', #6032, #22354 ) ;
#20304=CARTESIAN_POINT ( 'NONE',  ( 15.22780280894163063, -0.7747498539018873309, 5.363501450340581123 ) ) ;
#20315=CARTESIAN_POINT ( 'NONE',  ( -36.52679053911622020, 3.858136107555827810, -3.790289750283414527 ) ) ;
#20318=PLANE ( 'NONE',  #889 ) ;
#20324=EDGE_CURVE ( 'NONE', #17296, #8955, #266, .T. ) ;
#20327=CARTESIAN_POINT ( 'NONE',  ( 15.59055531549694074, 2.334444681449764136, -4.877899991435246108 ) ) ;
#20331=CARTESIAN_POINT ( 'NONE',  ( -54.49999999999997868, 0.000000000000000000, 0.000000000000000000 ) ) ;
#20332=CIRCLE ( 'NONE', #2108, 0.05000000000000008604 ) ;
#20344=CARTESIAN_POINT ( 'NONE',  ( -44.49999999999999289, -1.499999999999999556, -4.029888335921975262 ) ) ;
#20350=DIRECTION ( 'NONE',  ( 0.000000000000000000, 0.1576190026614809614, 0.9875000000000001554 ) ) ;
#20355=ORIENTED_EDGE ( 'NONE', *, *, #5828, .F. ) ;
#20359=EDGE_CURVE ( 'NONE', #24008, #9539, #19834, .T. ) ;
#20361=VERTEX_POINT ( 'NONE', #1128 ) ;
#20370=VERTEX_POINT ( 'NONE', #27096 ) ;
#20371=( BOUNDED_CURVE ( )  B_SPLINE_CURVE ( 3, ( #17990, #6118, #28103, #3434 ),
 .UNSPECIFIED., .F., .T. ) 
 B_SPLINE_CURVE_WITH_KNOTS ( ( 4, 4 ),
 ( 1.570796326794895892, 3.141592653589791784 ),
 .UNSPECIFIED. ) 
 CURVE ( )  GEOMETRIC_REPRESENTATION_ITEM ( )  RATIONAL_B_SPLINE_CURVE ( ( 1.000000000000000000, 0.8047378541243652705, 0.8047378541243652705, 1.000000000000000000 ) ) 
 REPRESENTATION_ITEM ( '' )  );
#20374=VECTOR ( 'NONE', #1142, 1000.000000000000000 ) ;
#20375=DIRECTION ( 'NONE',  ( -1.000000000000000000, -0.000000000000000000, -0.000000000000000000 ) ) ;
#20376=EDGE_CURVE ( 'NONE', #15713, #13616, #29789, .T. ) ;
#20381=CARTESIAN_POINT ( 'NONE',  ( 48.45343659158886851, 1.329326705022644051, 3.861343257506216098 ) ) ;
#20384=DIRECTION ( 'NONE',  ( -1.000000000000000000, -3.385297212316223527E-16, -2.459562394685754633E-16 ) ) ;
#20389=VERTEX_POINT ( 'NONE', #7950 ) ;
#20395=VERTEX_POINT ( 'NONE', #27413 ) ;
#20399=LINE ( 'NONE', #8338, #12145 ) ;
#20402=CARTESIAN_POINT ( 'NONE',  ( 57.00000000000001421, -0.7049799947465446026, -1.816196764953787124 ) ) ;
#20404=DIRECTION ( 'NONE',  ( 0.000000000000000000, 0.000000000000000000, -1.000000000000000000 ) ) ;
#20405=CARTESIAN_POINT ( 'NONE',  ( 56.95000000000001705, 0.000000000000000000, 0.000000000000000000 ) ) ;
#20406=DIRECTION ( 'NONE',  ( -0.000000000000000000, 0.2573099415204678775, -0.9663289263986324373 ) ) ;
#20408=CARTESIAN_POINT ( 'NONE',  ( -36.68866260399460799, 5.321612844166190293, -0.9647713018066405022 ) ) ;
#20410=EDGE_CURVE ( 'NONE', #26590, #8076, #5854, .T. ) ;
#20411=CARTESIAN_POINT ( 'NONE',  ( -36.00201293083839005, -2.199885893005511850, 4.939696249117965898 ) ) ;
#20417=CARTESIAN_POINT ( 'NONE',  ( 15.49676243306307200, 3.010474646410398414, 4.240315621469719076 ) ) ;
#20421=FACE_OUTER_BOUND ( 'NONE', #28223, .T. ) ;
#20426=ADVANCED_FACE ( 'NONE', ( #13005 ), #12038, .T. ) ;
#20431=CARTESIAN_POINT ( 'NONE',  ( 48.44664364291948999, 1.310522848978987298, 3.864668279552719632 ) ) ;
#20432=LINE ( 'NONE', #6021, #19730 ) ;
#20439=CARTESIAN_POINT ( 'NONE',  ( 33.47623932017462778, 1.734723475976807094E-15, 0.000000000000000000 ) ) ;
#20447=CARTESIAN_POINT ( 'NONE',  ( 47.00000000000002132, -4.137078223593629644, -1.088692053889325440 ) ) ;
#20451=CARTESIAN_POINT ( 'NONE',  ( 15.03925126672132961, -2.199885893005945725, 4.939696249117685234 ) ) ;
#20459=DIRECTION ( 'NONE',  ( 0.000000000000000000, 0.000000000000000000, -1.000000000000000000 ) ) ;
#20461=ORIENTED_EDGE ( 'NONE', *, *, #26690, .T. ) ;
#20465=CARTESIAN_POINT ( 'NONE',  ( -36.40793637698146057, 3.917775493694425570, -3.727542820438198401 ) ) ;
#20466=CARTESIAN_POINT ( 'NONE',  ( 15.03925126672125501, 3.779372838781817290, -3.883777296072506324 ) ) ;
#20468=DIRECTION ( 'NONE',  ( 1.000000000000000000, 0.000000000000000000, -0.000000000000000000 ) ) ;
#20471=B_SPLINE_CURVE_WITH_KNOTS ( 'NONE', 3,
 ( #2162, #24016, #26719, #28775, #5011, #11825, #2491, #29382, #7694, #14195, #19287, #23869, #16897, #21500, #16748, #26392, #4692, #26539, #2321 ),
 .UNSPECIFIED., .F., .F.,
 ( 4, 3, 3, 3, 3, 3, 4 ),
 ( 0.000000000000000000, 1.379880695094091716E-05, 1.586212677361243252E-05, 3.248035412973974761E-05, 5.074149073291455770E-05, 7.133938104856671239E-05, 9.012192312893275124E-05 ),
 .UNSPECIFIED. ) ;
#20476=FACE_OUTER_BOUND ( 'NONE', #14062, .T. ) ;
#20477=ORIENTED_EDGE ( 'NONE', *, *, #248, .T. ) ;
#20478=CARTESIAN_POINT ( 'NONE',  ( 44.98443556292537693, -3.726179070414207928, -1.100000000000000089 ) ) ;
#20480=EDGE_LOOP ( 'NONE', ( #4166, #9212, #11008, #14803 ) ) ;
#20484=CARTESIAN_POINT ( 'NONE',  ( 57.05000000000001847, 0.7794871794871796045, -1.732743413496389939 ) ) ;
#20490=DIRECTION ( 'NONE',  ( 0.000000000000000000, 0.000000000000000000, -1.000000000000000000 ) ) ;
#20491=MECHANICAL_DESIGN_GEOMETRIC_PRESENTATION_REPRESENTATION('',(#26026),#1740);
#20500=DIRECTION ( 'NONE',  ( 1.000000000000000000, 0.000000000000000000, -0.000000000000000000 ) ) ;
#20501=B_SPLINE_CURVE_WITH_KNOTS ( 'NONE', 3,
 ( #22792, #11525, #11343, #21028, #2163, #16271, #16598, #26074, #21201, #4694, #11826, #14035, #30667, #30833, #9303, #11679, #16751, #4385, #18967 ),
 .UNSPECIFIED., .F., .F.,
 ( 4, 3, 3, 3, 3, 3, 4 ),
 ( -1.485273975135215818E-06, 0.000000000000000000, 2.074191569004179043E-05, 3.882553518188196033E-05, 5.450508821808581838E-05, 6.929665250580413082E-05, 8.415228772525333491E-05 ),
 .UNSPECIFIED. ) ;
#20504=AXIS2_PLACEMENT_3D ( 'NONE', #10497, #2738, #3199 ) ;
#20506=DIRECTION ( 'NONE',  ( 1.000000000000000000, 0.000000000000000000, 0.000000000000000000 ) ) ;
#20507=ADVANCED_FACE ( 'NONE', ( #8706 ), #20917, .T. ) ;
#20510=ORIENTED_EDGE ( 'NONE', *, *, #8640, .T. ) ;
#20511=SURFACE_SIDE_STYLE ('',( #13660 ) ) ;
#20512=DIRECTION ( 'NONE',  ( 1.000000000000000000, 0.000000000000000000, 0.000000000000000000 ) ) ;
#20526=CARTESIAN_POINT ( 'NONE',  ( 47.03773326306244940, -4.256154442720823994, -1.015631899367381408 ) ) ;
#20538=CIRCLE ( 'NONE', #9409, 4.275000000000000355 ) ;
#20540=CIRCLE ( 'NONE', #17493, 1.899999999999999911 ) ;
#20541=DIRECTION ( 'NONE',  ( -0.000000000000000000, -0.000000000000000000, 1.000000000000000000 ) ) ;
#20544=AXIS2_PLACEMENT_3D ( 'NONE', #11835, #12290, #31149 ) ;
#20547=ORIENTED_EDGE ( 'NONE', *, *, #27619, .F. ) ;
#20548=EDGE_CURVE ( 'NONE', #9481, #20395, #24074, .T. ) ;
#20553=CARTESIAN_POINT ( 'NONE',  ( -35.85663232820592583, -5.086913985776160274, 1.171642053949097262 ) ) ;
#20560=ORIENTED_EDGE ( 'NONE', *, *, #1688, .F. ) ;
#20561=CARTESIAN_POINT ( 'NONE',  ( 50.29999999999825633, 1.391941090720882235, 3.849999999997240074 ) ) ;
#20563=CYLINDRICAL_SURFACE ( 'NONE', #18527, 0.09999999999999982514 ) ;
#20564=ORIENTED_EDGE ( 'NONE', *, *, #21330, .F. ) ;
#20565=CARTESIAN_POINT ( 'NONE',  ( -36.22955757456081471, 4.863043649742752272, -1.860644097022596588 ) ) ;
#20566=VECTOR ( 'NONE', #27258, 1000.000000000000000 ) ;
#20568=CARTESIAN_POINT ( 'NONE',  ( -35.85663232820584057, -2.199885893005967041, 4.939696249117680793 ) ) ;
#20570=CARTESIAN_POINT ( 'NONE',  ( 47.10000000000002274, -4.259181259350203419, 0.9999999999999995559 ) ) ;
#20571=CARTESIAN_POINT ( 'NONE',  ( 57.00000000000001421, 0.6999999999999999556, -1.820027472320129736 ) ) ;
#20577=CARTESIAN_POINT ( 'NONE',  ( 15.29384114148384022, 2.734418404389609147, 4.440882220947752757 ) ) ;
#20579=CARTESIAN_POINT ( 'NONE',  ( 47.00000000000002132, -3.826179070414207573, -1.000000000000000000 ) ) ;
#20583=AXIS2_PLACEMENT_3D ( 'NONE', #18755, #15458, #6701 ) ;
#20585=CARTESIAN_POINT ( 'NONE',  ( 48.46185180831791683, 1.426738236278596972, -3.843750512866276559 ) ) ;
#20586=EDGE_LOOP ( 'NONE', ( #15463, #15865, #14650, #6821 ) ) ;
#20590=VERTEX_POINT ( 'NONE', #19022 ) ;
#20593=CARTESIAN_POINT ( 'NONE',  ( 48.30000000000001847, 2.428612866367529932E-14, -4.100000000000022737 ) ) ;
#20595=ORIENTED_EDGE ( 'NONE', *, *, #10551, .F. ) ;
#20597=FACE_OUTER_BOUND ( 'NONE', #12574, .T. ) ;
#20599=DIRECTION ( 'NONE',  ( 1.000000000000000000, -0.000000000000000000, -0.000000000000000000 ) ) ;
#20611=CARTESIAN_POINT ( 'NONE',  ( 47.03912372675481635, -4.170474612306438011, -1.019817338724548605 ) ) ;
#20612=AXIS2_PLACEMENT_3D ( 'NONE', #13575, #3935, #4236 ) ;
#20615=CARTESIAN_POINT ( 'NONE',  ( 15.41217651307625047, -0.2668145608218825959, 5.199999998579027505 ) ) ;
#20617=AXIS2_PLACEMENT_3D ( 'NONE', #22923, #5508, #20251 ) ;
#20619=DIRECTION ( 'NONE',  ( 1.000000000000000000, 3.385297212316223527E-16, 2.459562394685754633E-16 ) ) ;
#20620=CARTESIAN_POINT ( 'NONE',  ( -36.22909104983143180, 0.6969927240739536289, -5.374332520738267505 ) ) ;
#20621=CIRCLE ( 'NONE', #21652, 4.700000000000000178 ) ;
#20631=DIRECTION ( 'NONE',  ( 0.000000000000000000, 1.532429380227459806E-15, -1.000000000000000000 ) ) ;
#20632=ORIENTED_EDGE ( 'NONE', *, *, #21461, .F. ) ;
#20636=EDGE_LOOP ( 'NONE', ( #478, #3292, #7219, #19580 ) ) ;
#20637=DIRECTION ( 'NONE',  ( 0.000000000000000000, 0.000000000000000000, 1.000000000000000000 ) ) ;
#20639=VERTEX_POINT ( 'NONE', #26600 ) ;
#20642=ORIENTED_EDGE ( 'NONE', *, *, #28568, .F. ) ;
#20652=EDGE_CURVE ( 'NONE', #14026, #22708, #4198, .T. ) ;
#20656=EDGE_CURVE ( 'NONE', #30388, #28184, #2217, .T. ) ;
#20676=ORIENTED_EDGE ( 'NONE', *, *, #13274, .F. ) ;
#20679=AXIS2_PLACEMENT_3D ( 'NONE', #6512, #16170, #25818 ) ;
#20683=CARTESIAN_POINT ( 'NONE',  ( -35.85663232820584057, -2.686240680702168593, 4.475885388010719446 ) ) ;
#20689=ORIENTED_EDGE ( 'NONE', *, *, #20359, .T. ) ;
#20690=CARTESIAN_POINT ( 'NONE',  ( 46.90000000000002700, -4.227689052994015206, -1.125730994152046138 ) ) ;
#20692=LINE ( 'NONE', #8767, #10886 ) ;
#20698=CARTESIAN_POINT ( 'NONE',  ( 57.00529107662529782, 0.7231510886217332734, -1.801575813826951533 ) ) ;
#20701=CARTESIAN_POINT ( 'NONE',  ( 56.95000000000001705, 0.7000000000000000666, 2.452039967047845437 ) ) ;
#20713=DIRECTION ( 'NONE',  ( 0.000000000000000000, -0.1576190026614809614, -0.9875000000000001554 ) ) ;
#20715=ADVANCED_FACE ( 'NONE', ( #949 ), #10439, .F. ) ;
#20724=ORIENTED_EDGE ( 'NONE', *, *, #16828, .F. ) ;
#20725=CARTESIAN_POINT ( 'NONE',  ( -36.31440869660545445, 4.962395293451402623, -1.554871187131892318 ) ) ;
#20730=CARTESIAN_POINT ( 'NONE',  ( -35.85663232820584767, 4.383220986679566167, 0.4611378927910952386 ) ) ;
#20732=CARTESIAN_POINT ( 'NONE',  ( 15.41170998834775219, 3.722832355337220456, 3.938244298533839505 ) ) ;
#20737=LINE ( 'NONE', #27372, #958 ) ;
#20745=CARTESIAN_POINT ( 'NONE',  ( 48.40130545986176003, 0.9107929593200400076, 3.923749358243191043 ) ) ;
#20747=ORIENTED_EDGE ( 'NONE', *, *, #23377, .T. ) ;
#20750=DIRECTION ( 'NONE',  ( 0.000000000000000000, 0.000000000000000000, -1.000000000000000000 ) ) ;
#20751=CIRCLE ( 'NONE', #23255, 0.05000000000000012768 ) ;
#20752=ADVANCED_FACE ( 'NONE', ( #3310 ), #10744, .T. ) ;
#20755=ORIENTED_EDGE ( 'NONE', *, *, #6748, .F. ) ;
#20757=CARTESIAN_POINT ( 'NONE',  ( 57.00000000000001421, -0.7500000000000000000, 2.421260002560649660 ) ) ;
#20764=CARTESIAN_POINT ( 'NONE',  ( 47.05865997105815524, -4.175606900721715142, -1.008275291528680784 ) ) ;
#20765=CARTESIAN_POINT ( 'NONE',  ( -36.80043232705877898, 2.728070298465809618, -4.669343935538267765 ) ) ;
#20771=CYLINDRICAL_SURFACE ( 'NONE', #31114, 0.05000000000000012768 ) ;
#20772=DIRECTION ( 'NONE',  ( -1.000000000000000000, -2.586136946169074517E-16, 0.000000000000000000 ) ) ;
#20779=DIRECTION ( 'NONE',  ( 0.000000000000000000, 0.000000000000000000, 1.000000000000000000 ) ) ;
#20782=DIRECTION ( 'NONE',  ( -1.293068473084537258E-16, 1.000000000000000000, 0.000000000000000000 ) ) ;
#20783=EDGE_CURVE ( 'NONE', #6738, #20184, #12961, .T. ) ;
#20791=CIRCLE ( 'NONE', #9150, 3.625000000000000444 ) ;
#20800=DIRECTION ( 'NONE',  ( 0.000000000000000000, 0.000000000000000000, -1.000000000000000000 ) ) ;
#20804=CARTESIAN_POINT ( 'NONE',  ( -35.85663232820584057, 3.056483311920803025, 4.206888370749761741 ) ) ;
#20808=CARTESIAN_POINT ( 'NONE',  ( 56.95000043478394502, 0.7674401070440159955, -2.484784916619714679 ) ) ;
#20815=SURFACE_STYLE_USAGE ( .BOTH. , #20511 ) ;
#20818=CARTESIAN_POINT ( 'NONE',  ( 50.50000000000002132, 2.428612866367529932E-14, 0.000000000000000000 ) ) ;
#20821=EDGE_LOOP ( 'NONE', ( #28694, #27234, #13503, #4884 ) ) ;
#20827=ORIENTED_EDGE ( 'NONE', *, *, #14885, .F. ) ;
#20837=CARTESIAN_POINT ( 'NONE',  ( 15.97944027357901042, 2.710596767400014429, 4.680923748383045258 ) ) ;
#20840=CARTESIAN_POINT ( 'NONE',  ( 57.00320971560400096, 0.7176258130632211518, -1.806074485252040285 ) ) ;
#20855=EDGE_CURVE ( 'NONE', #8913, #3555, #4239, .T. ) ;
#20860=ADVANCED_FACE ( 'NONE', ( #25316 ), #15670, .F. ) ;
#20861=ORIENTED_EDGE ( 'NONE', *, *, #14651, .F. ) ;
#20866=CARTESIAN_POINT ( 'NONE',  ( 34.50000000000001421, 0.000000000000000000, 0.000000000000000000 ) ) ;
#20867=CYLINDRICAL_SURFACE ( 'NONE', #25642, 1.000000000000000000 ) ;
#20870=CARTESIAN_POINT ( 'NONE',  ( -36.92362342067168868, 5.092377074781550661, -1.825725187625013346 ) ) ;
#20873=CARTESIAN_POINT ( 'NONE',  ( 56.95000000000001705, 0.6820512820512817376, 1.773360101234997988 ) ) ;
#20882=LINE ( 'NONE', #30511, #16400 ) ;
#20884=CARTESIAN_POINT ( 'NONE',  ( 48.37893541770432648, 0.9199776782966302413, -3.998258245321878235 ) ) ;
#20887=ORIENTED_EDGE ( 'NONE', *, *, #15693, .F. ) ;
#20889=CARTESIAN_POINT ( 'NONE',  ( 48.38950019258942348, 0.7811435014053292880, 4.027217152859519089 ) ) ;
#20891=EDGE_LOOP ( 'NONE', ( #5286, #22202, #138, #29816 ) ) ;
#20900=DIRECTION ( 'NONE',  ( 1.000000000000000000, 0.000000000000000000, 0.000000000000000000 ) ) ;
#20908=CARTESIAN_POINT ( 'NONE',  ( -36.77443515226919857, 3.646557212684436777, -3.995389720703250713 ) ) ;
#20912=ADVANCED_FACE ( 'NONE', ( #31158 ), #2345, .T. ) ;
#20913=CARTESIAN_POINT ( 'NONE',  ( 57.01549179440438309, -0.7366256376427431363, -2.429951667075468613 ) ) ;
#20914=CARTESIAN_POINT ( 'NONE',  ( 17.21035195517769267, -2.471857751707523654E-15, 0.000000000000000000 ) ) ;
#20916=EDGE_CURVE ( 'NONE', #10216, #13616, #11202, .T. ) ;
#20917=TOROIDAL_SURFACE ( 'NONE', #5717, 3.299999999999999822, 0.1000000000000000056 ) ;
#20927=CARTESIAN_POINT ( 'NONE',  ( 15.45522337368515409, -5.005099703116265175, 1.423440526321969157 ) ) ;
#20943=VERTEX_POINT ( 'NONE', #26558 ) ;
#20949=CARTESIAN_POINT ( 'NONE',  ( 51.90000000000001279, 1.734723475976807094E-15, -4.275000000000000355 ) ) ;
#20952=EDGE_CURVE ( 'NONE', #24423, #4345, #16877, .T. ) ;
#20957=CARTESIAN_POINT ( 'NONE',  ( 15.41080140630216810, 5.326563020867391529, -0.9981196555231990342 ) ) ;
#20959=CARTESIAN_POINT ( 'NONE',  ( 50.40000000000001990, 2.428612866367529932E-14, 0.000000000000000000 ) ) ;
#20961=CARTESIAN_POINT ( 'NONE',  ( 50.38699024846547303, 1.088846059295805135, -3.899771020632008423 ) ) ;
#20964=CARTESIAN_POINT ( 'NONE',  ( -36.14504829323105639, -1.093755498983980612, -5.295967089285813501 ) ) ;
#20983=CARTESIAN_POINT ( 'NONE',  ( 58.45000000000001705, -0.8000000000000001554, 1.778341924377873973 ) ) ;
#20985=VERTEX_POINT ( 'NONE', #274 ) ;
#20988=AXIS2_PLACEMENT_3D ( 'NONE', #28291, #23538, #21191 ) ;
#20989=CARTESIAN_POINT ( 'NONE',  ( 57.00057550097274373, -0.8023623105721646720, -2.473098203180232879 ) ) ;
#20992=EDGE_CURVE ( 'NONE', #10297, #12844, #21833, .T. ) ;
#21001=DIRECTION ( 'NONE',  ( -1.000000000000000000, -0.000000000000000000, -0.000000000000000000 ) ) ;
#21003=CIRCLE ( 'NONE', #12412, 1.000000000000000000 ) ;
#21006=EDGE_CURVE ( 'NONE', #11687, #19238, #22933, .T. ) ;
#21013=CARTESIAN_POINT ( 'NONE',  ( -36.48821680285229263, 2.849134329833883594, 4.601168830303214108 ) ) ;
#21016=CARTESIAN_POINT ( 'NONE',  ( -54.49999999999997868, 2.270506450603774156E-15, 4.375000000000000000 ) ) ;
#21020=FACE_OUTER_BOUND ( 'NONE', #10543, .T. ) ;
#21021=DIRECTION ( 'NONE',  ( 1.000000000000000000, 0.000000000000000000, 0.000000000000000000 ) ) ;
#21023=DIRECTION ( 'NONE',  ( 0.000000000000000000, 0.000000000000000000, -1.000000000000000000 ) ) ;
#21027=FACE_BOUND ( 'NONE', #12292, .T. ) ;
#21028=CARTESIAN_POINT ( 'NONE',  ( -54.49998431799114940, -1.548747819918198987, -3.331336553795240185 ) ) ;
#21029=CARTESIAN_POINT ( 'NONE',  ( 58.45000000000001705, 0.8000000000000000444, 2.471260002560650371 ) ) ;
#21032=CARTESIAN_POINT ( 'NONE',  ( 51.83867713794252552, 0.3186276668619861807, 4.343079704710790523 ) ) ;
#21033=AXIS2_PLACEMENT_3D ( 'NONE', #3149, #12790, #10432 ) ;
#21034=AXIS2_PLACEMENT_3D ( 'NONE', #9394, #16208, #6854 ) ;
#21035=ADVANCED_FACE ( 'NONE', ( #3118 ), #31011, .T. ) ;
#21036=DIRECTION ( 'NONE',  ( 1.000000000000000000, -0.000000000000000000, -0.000000000000000000 ) ) ;
#21038=CARTESIAN_POINT ( 'NONE',  ( 50.50000002742975624, 0.7904052113207085117, -4.025738854575411807 ) ) ;
#21045=ORIENTED_EDGE ( 'NONE', *, *, #5760, .F. ) ;
#21047=CARTESIAN_POINT ( 'NONE',  ( -36.48821680285185920, -0.3995010896672921419, 5.397102918580241493 ) ) ;
#21053=DIRECTION ( 'NONE',  ( 1.000000000000000000, 0.000000000000000000, 4.738179285253040686E-16 ) ) ;
#21055=EDGE_LOOP ( 'NONE', ( #3309, #20887, #29841, #63 ) ) ;
#21057=ORIENTED_EDGE ( 'NONE', *, *, #30622, .T. ) ;
#21060=AXIS2_PLACEMENT_3D ( 'NONE', #13043, #20500, #27916 ) ;
#21066=CARTESIAN_POINT ( 'NONE',  ( -36.81959771849334828, 2.696520634775258607, 4.691964194339944605 ) ) ;
#21071=CIRCLE ( 'NONE', #1832, 1.000000000000000000 ) ;
#21073=CARTESIAN_POINT ( 'NONE',  ( 50.30000000000001847, -1.391941090707485396, -3.850000000000022737 ) ) ;
#21075=CARTESIAN_POINT ( 'NONE',  ( -35.85663232820583346, -4.683225679163351529, -2.703237727951242952 ) ) ;
#21077=CARTESIAN_POINT ( 'NONE',  ( -35.85663232820601820, 4.018128179617554530, -3.618665901676620500 ) ) ;
#21083=AXIS2_PLACEMENT_3D ( 'NONE', #28722, #2589, #16845 ) ;
#21084=CARTESIAN_POINT ( 'NONE',  ( 15.71019289815287223, 0.8926979523208264933, -5.334280177567949366 ) ) ;
#21090=CIRCLE ( 'NONE', #9444, 3.625000000000028866 ) ;
#21092=CARTESIAN_POINT ( 'NONE',  ( 17.21035195517769267, -5.407411300779135566, 6.622168941172392137E-16 ) ) ;
#21098=DIRECTION ( 'NONE',  ( 1.000000000000000000, 0.000000000000000000, 0.000000000000000000 ) ) ;
#21099=CARTESIAN_POINT ( 'NONE',  ( -36.26369610968610857, 4.878538113278829691, 1.812957040858136804 ) ) ;
#21101=ORIENTED_EDGE ( 'NONE', *, *, #2688, .T. ) ;
#21103=CARTESIAN_POINT ( 'NONE',  ( -36.48174642952978530, -5.008501212420972237, 2.048848402342071218 ) ) ;
#21106=DIRECTION ( 'NONE',  ( 0.000000000000000000, 0.000000000000000000, 1.000000000000000000 ) ) ;
#21107=AXIS2_PLACEMENT_3D ( 'NONE', #23125, #30526, #25793 ) ;
#21112=EDGE_CURVE ( 'NONE', #13515, #25588, #24966, .T. ) ;
#21117=EDGE_CURVE ( 'NONE', #25822, #4862, #17270, .T. ) ;
#21119=ORIENTED_EDGE ( 'NONE', *, *, #3069, .T. ) ;
#21120=AXIS2_PLACEMENT_3D ( 'NONE', #927, #22311, #29887 ) ;
#21130=AXIS2_PLACEMENT_3D ( 'NONE', #21197, #21021, #4378 ) ;
#21133=DIRECTION ( 'NONE',  ( -1.000000000000000000, -0.000000000000000000, -0.000000000000000000 ) ) ;
#21134=CARTESIAN_POINT ( 'NONE',  ( -36.81959771849334828, -2.696520634775307457, -4.691964194339934835 ) ) ;
#21135=CARTESIAN_POINT ( 'NONE',  ( 57.04415282905778639, 0.8156862745098041323, 2.468735688885368873 ) ) ;
#21141=CARTESIAN_POINT ( 'NONE',  ( 47.00000000000002132, 2.478823385132571406E-14, 4.100000000000022737 ) ) ;
#21149=CARTESIAN_POINT ( 'NONE',  ( 15.48609859788819598, 4.910307320510450602, 1.715181477143260969 ) ) ;
#21151=EDGE_CURVE ( 'NONE', #23938, #4123, #12310, .T. ) ;
#21154=ORIENTED_EDGE ( 'NONE', *, *, #25467, .T. ) ;
#21160=ORIENTED_EDGE ( 'NONE', *, *, #18205, .F. ) ;
#21161=AXIS2_PLACEMENT_3D ( 'NONE', #30657, #28297, #20404 ) ;
#21169=B_SPLINE_CURVE_WITH_KNOTS ( 'NONE', 3,
 ( #18204, #27845, #25456, #6156, #22469, #15807 ),
 .UNSPECIFIED., .F., .F.,
 ( 4, 2, 4 ),
 ( 0.000000000000000000, 0.0001620412083492953114, 0.0003240824166985906227 ),
 .UNSPECIFIED. ) ;
#21176=CARTESIAN_POINT ( 'NONE',  ( 46.89999999999999858, -4.241634596362394483, 1.073358427932564529 ) ) ;
#21177=CYLINDRICAL_SURFACE ( 'NONE', #3168, 0.05000000000000012768 ) ;
#21180=CIRCLE ( 'NONE', #7514, 4.000000000000022204 ) ;
#21183=CARTESIAN_POINT ( 'NONE',  ( 51.83857334934266703, 0.3198555306840176748, -4.342911177030791769 ) ) ;
#21186=B_SPLINE_CURVE_WITH_KNOTS ( 'NONE', 3,
 ( #656, #54, #4956, #5417, #5251, #15073, #29328, #22062, #3043, #7639, #24275, #7329, #12686, #2587, #21918, #2884 ),
 .UNSPECIFIED., .F., .F.,
 ( 4, 2, 2, 2, 2, 2, 2, 4 ),
 ( 0.000000000000000000, 0.0004351083927046461137, 0.0008702167854092922273, 0.001740433570818584455, 0.002175541963523229972, 0.002610650356227875706, 0.003045758748932521440, 0.003480867141637167175 ),
 .UNSPECIFIED. ) ;
#21191=DIRECTION ( 'NONE',  ( 0.000000000000000000, 0.000000000000000000, -1.000000000000000000 ) ) ;
#21192=ORIENTED_EDGE ( 'NONE', *, *, #487, .F. ) ;
#21194=DIRECTION ( 'NONE',  ( -1.000000000000000000, 0.000000000000000000, 0.000000000000000000 ) ) ;
#21196=CARTESIAN_POINT ( 'NONE',  ( 50.38490132722630932, 1.114141714781645254, 3.896173399896523559 ) ) ;
#21197=CARTESIAN_POINT ( 'NONE',  ( -35.85663232820584057, -0.9159215771380563309, 4.311190327365815200 ) ) ;
#21201=CARTESIAN_POINT ( 'NONE',  ( -54.49181037333889321, -1.522049374736507144, -3.314263409011525940 ) ) ;
#21205=CARTESIAN_POINT ( 'NONE',  ( 51.80000000000001137, 1.280326109884211361, 4.104114837514009295 ) ) ;
#21210=CARTESIAN_POINT ( 'NONE',  ( 50.40000000000001279, 0.6462379109120997001, -4.048750000000022276 ) ) ;
#21216=CARTESIAN_POINT ( 'NONE',  ( -36.39645873810206211, 0.5233326973447959274, 5.388419908789453316 ) ) ;
#21221=CARTESIAN_POINT ( 'NONE',  ( 15.03925126672132784, 4.945493884734782242, 1.606888370749786521 ) ) ;
#21228=DIRECTION ( 'NONE',  ( 0.000000000000000000, 1.000000000000000000, 0.000000000000000000 ) ) ;
#21234=CARTESIAN_POINT ( 'NONE',  ( 47.10000000000002274, -4.276948333784438283, -0.9210526315789475671 ) ) ;
#21239=CARTESIAN_POINT ( 'NONE',  ( -54.49999999999997868, 1.549999999999999600, -4.064480286580312907 ) ) ;
#21240=ORIENTED_EDGE ( 'NONE', *, *, #19685, .F. ) ;
#21244=CARTESIAN_POINT ( 'NONE',  ( -36.30424252565904908, 3.146183597690369815, -4.141717300434357263 ) ) ;
#21249=CIRCLE ( 'NONE', #14143, 0.4576450603546999840 ) ;
#21254=CIRCLE ( 'NONE', #12124, 0.05000000000000012768 ) ;
#21257=ORIENTED_EDGE ( 'NONE', *, *, #14084, .T. ) ;
#21262=CARTESIAN_POINT ( 'NONE',  ( -36.76447480099743359, 5.297368390263413218, 1.087079755157708272 ) ) ;
#21263=CARTESIAN_POINT ( 'NONE',  ( 15.49676243306310219, -4.963067629822646154, 1.552801941062276425 ) ) ;
#21266=FACE_OUTER_BOUND ( 'NONE', #24257, .T. ) ;
#21267=CARTESIAN_POINT ( 'NONE',  ( 57.05000000000001847, 0.7794871794871796045, -1.732743413496389939 ) ) ;
#21268=ADVANCED_FACE ( 'NONE', ( #4831 ), #27503, .T. ) ;
#21269=EDGE_LOOP ( 'NONE', ( #8164, #19383, #19156, #21045, #1007 ) ) ;
#21272=ORIENTED_EDGE ( 'NONE', *, *, #13024, .F. ) ;
#21280=AXIS2_PLACEMENT_3D ( 'NONE', #20983, #13989, #16073 ) ;
#21288=CARTESIAN_POINT ( 'NONE',  ( -36.89831264271882105, 5.047763082740440055, -1.943828653492478242 ) ) ;
#21291=CARTESIAN_POINT ( 'NONE',  ( 46.99404308269125607, -4.272100939101181716, 0.9440912809989528975 ) ) ;
#21292=DIRECTION ( 'NONE',  ( 0.000000000000000000, -1.000000000000000000, 0.000000000000000000 ) ) ;
#21293=FACE_OUTER_BOUND ( 'NONE', #21335, .T. ) ;
#21304=ORIENTED_EDGE ( 'NONE', *, *, #28431, .T. ) ;
#21310=CARTESIAN_POINT ( 'NONE',  ( 15.17214319754861229, 4.804073785499177518, 2.042134698606610677 ) ) ;
#21315=CARTESIAN_POINT ( 'NONE',  ( 17.21035195517767846, 24.59258869922086532, 0.000000000000000000 ) ) ;
#21324=B_SPLINE_CURVE_WITH_KNOTS ( 'NONE', 3,
 ( #22967, #20447, #1257, #13597, #29929, #5870, #30072, #18376, #20611, #13434, #20764, #23134, #1423, #8093, #11083, #8390 ),
 .UNSPECIFIED., .F., .F.,
 ( 4, 3, 3, 3, 3, 4 ),
 ( 0.000000000000000000, 3.843454199181275667E-05, 7.602611568626176531E-05, 0.0001118455301991773924, 0.0001459326773459512306, 0.0001653157283245149816 ),
 .UNSPECIFIED. ) ;
#21326=CARTESIAN_POINT ( 'NONE',  ( 56.95150694030147775, 0.7014737422875408912, 1.765795469766037185 ) ) ;
#21327=CARTESIAN_POINT ( 'NONE',  ( 57.05000000000001847, 0.7794871794871796045, 1.732743413496389939 ) ) ;
#21330=EDGE_CURVE ( 'NONE', #24678, #26348, #30813, .T. ) ;
#21332=EDGE_CURVE ( 'NONE', #560, #17756, #11551, .T. ) ;
#21333=DIRECTION ( 'NONE',  ( 0.000000000000000000, -2.168404344971008868E-16, -1.000000000000000000 ) ) ;
#21335=EDGE_LOOP ( 'NONE', ( #24570, #7753, #8191, #21257 ) ) ;
#21338=CARTESIAN_POINT ( 'NONE',  ( -54.44999999999997442, 0.000000000000000000, 0.000000000000000000 ) ) ;
#21343=CARTESIAN_POINT ( 'NONE',  ( -35.98952425903311791, 3.426725954212571423, 3.937891351789597039 ) ) ;
#21344=ORIENTED_EDGE ( 'NONE', *, *, #5257, .T. ) ;
#21346=CARTESIAN_POINT ( 'NONE',  ( 56.95000000000001705, 0.6999999999999998446, 1.820027472320129514 ) ) ;
#21348=EDGE_CURVE ( 'NONE', #2309, #11630, #16092, .T. ) ;
#21358=FACE_OUTER_BOUND ( 'NONE', #5543, .T. ) ;
#21360=CARTESIAN_POINT ( 'NONE',  ( 51.88790733220172058, 0.01048319233286296517, 4.374313010691237125 ) ) ;
#21370=CARTESIAN_POINT ( 'NONE',  ( -36.31440869660544735, -0.05469410396133057850, 5.200000001157072838 ) ) ;
#21372=ORIENTED_EDGE ( 'NONE', *, *, #25455, .T. ) ;
#21373=DIRECTION ( 'NONE',  ( -1.000000000000000000, 0.000000000000000000, 0.000000000000000000 ) ) ;
#21374=ORIENTED_EDGE ( 'NONE', *, *, #13531, .T. ) ;
#21376=CARTESIAN_POINT ( 'NONE',  ( -35.85663232820584057, 1.123735532908288315, 5.289358697221541838 ) ) ;
#21377=FACE_OUTER_BOUND ( 'NONE', #11975, .T. ) ;
#21381=EDGE_CURVE ( 'NONE', #13894, #1995, #24881, .T. ) ;
#21392=CARTESIAN_POINT ( 'NONE',  ( -54.49608498031047787, 1.530604779201329535, -4.051096982736679841 ) ) ;
#21393=ORIENTED_EDGE ( 'NONE', *, *, #16178, .F. ) ;
#21396=CARTESIAN_POINT ( 'NONE',  ( 48.40000000000001990, 0.6304760106459518232, 3.950000000000022826 ) ) ;
#21397=DIRECTION ( 'NONE',  ( 1.000000000000000000, 5.172273892338149033E-16, 0.000000000000000000 ) ) ;
#21398=LINE ( 'NONE', #31025, #7853 ) ;
#21401=DIRECTION ( 'NONE',  ( -0.000000000000000000, 1.000000000000000000, 0.000000000000000000 ) ) ;
#21404=CARTESIAN_POINT ( 'NONE',  ( 50.34665981758796960, -1.329038565861417220, -3.861394075523871816 ) ) ;
#21408=CARTESIAN_POINT ( 'NONE',  ( 16.07279755198655025, -2.910597594660164322, -4.559461819278072703 ) ) ;
#21413=CARTESIAN_POINT ( 'NONE',  ( 50.34130827207516745, -1.344780351710843425, 3.858600739747801711 ) ) ;
#21416=CARTESIAN_POINT ( 'NONE',  ( 56.97354279652698494, 0.7803351525568237301, -2.480154250529269522 ) ) ;
#21418=ORIENTED_EDGE ( 'NONE', *, *, #25276, .T. ) ;
#21420=VERTEX_POINT ( 'NONE', #10946 ) ;
#21426=CARTESIAN_POINT ( 'NONE',  ( 48.30000000000001847, -0.6462379109120514054, 4.048750000000023164 ) ) ;
#21429=CIRCLE ( 'NONE', #18385, 1.000000000000000000 ) ;
#21431=EDGE_CURVE ( 'NONE', #5143, #12299, #27269, .T. ) ;
#21435=EDGE_CURVE ( 'NONE', #17963, #26911, #11739, .T. ) ;
#21436=CARTESIAN_POINT ( 'NONE',  ( 46.90000000000002700, -4.227689052994015206, 1.125730994152047471 ) ) ;
#21438=CARTESIAN_POINT ( 'NONE',  ( 15.41217651307625225, 5.027944117024030213, -1.353132643598505380 ) ) ;
#21440=DIRECTION ( 'NONE',  ( 0.000000000000000000, 0.000000000000000000, 1.000000000000000000 ) ) ;
#21443=CARTESIAN_POINT ( 'NONE',  ( 48.30268563551750560, -0.9333771270347004378, 3.994943142064449670 ) ) ;
#21444=CARTESIAN_POINT ( 'NONE',  ( 50.30000000000001847, -1.391941090707491835, 3.850000000000022293 ) ) ;
#21454=DIRECTION ( 'NONE',  ( -1.000000000000000000, -2.586136946169074517E-16, 0.000000000000000000 ) ) ;
#21456=LINE ( 'NONE', #21930, #6074 ) ;
#21460=DIRECTION ( 'NONE',  ( 2.459562394685749702E-16, -0.9510565162951545304, 0.3090169943749447312 ) ) ;
#21461=EDGE_CURVE ( 'NONE', #4123, #19150, #13931, .T. ) ;
#21462=DIRECTION ( 'NONE',  ( 0.000000000000000000, -1.000000000000000000, -0.000000000000000000 ) ) ;
#21464=EDGE_LOOP ( 'NONE', ( #8259, #12702, #26877, #12769, #18020 ) ) ;
#21472=CARTESIAN_POINT ( 'NONE',  ( 48.30000000000001847, 2.428612866367529932E-14, 0.000000000000000000 ) ) ;
#21475=B_SPLINE_CURVE_WITH_KNOTS ( 'NONE', 3,
 ( #28842, #25713, #18288, #4020, #26307, #2076, #12063, #21416, #23934, #11741, #18441, #7154, #4755, #2227, #16818, #11891 ),
 .UNSPECIFIED., .F., .F.,
 ( 4, 3, 3, 3, 3, 4 ),
 ( 0.000000000000000000, 2.806063833126217928E-05, 6.345755872418550124E-05, 9.706205683209630718E-05, 0.0001297115041001252684, 0.0001622821609780518274 ),
 .UNSPECIFIED. ) ;
#21477=CARTESIAN_POINT ( 'NONE',  ( 51.80021594609809199, -4.243814194680251894, 1.064485530476970032 ) ) ;
#21489=CARTESIAN_POINT ( 'NONE',  ( -36.50489844130379424, 3.461789369942879002, 4.158232265984318055 ) ) ;
#21494=VERTEX_POINT ( 'NONE', #21267 ) ;
#21495=CARTESIAN_POINT ( 'NONE',  ( 50.46980263351819929, 1.141995257496368987, 3.938405479918978713 ) ) ;
#21496=FACE_OUTER_BOUND ( 'NONE', #23678, .T. ) ;
#21498=DIRECTION ( 'NONE',  ( 0.000000000000000000, 0.000000000000000000, -1.000000000000000000 ) ) ;
#21499=EDGE_CURVE ( 'NONE', #22540, #27746, #19847, .T. ) ;
#21500=CARTESIAN_POINT ( 'NONE',  ( 57.00630022123013418, 0.7249518695496515175, 1.800067615291236711 ) ) ;
#21501=ADVANCED_FACE ( 'NONE', ( #1591 ), #18875, .T. ) ;
#21502=CARTESIAN_POINT ( 'NONE',  ( 15.03925126672133139, -5.086913985776138958, -1.171642053949127460 ) ) ;
#21503=CARTESIAN_POINT ( 'NONE',  ( 57.05000000000001137, 0.7500000000000002220, -1.746008434843742796 ) ) ;
#21504=CIRCLE ( 'NONE', #20504, 4.700000000000000178 ) ;
#21505=ADVANCED_FACE ( 'NONE', ( #26145 ), #5766, .F. ) ;
#21508=LINE ( 'NONE', #19293, #30674 ) ;
#21509=DIRECTION ( 'NONE',  ( 1.000000000000000000, 0.000000000000000000, -0.000000000000000000 ) ) ;
#21516=CARTESIAN_POINT ( 'NONE',  ( 57.05000000000001137, -0.8156862745098039102, -2.468735688885371982 ) ) ;
#21517=CARTESIAN_POINT ( 'NONE',  ( -35.85663232820601820, -1.123735532908291423, 5.289358697221548944 ) ) ;
#21526=EDGE_LOOP ( 'NONE', ( #20477, #23311, #21929, #28642 ) ) ;
#21528=LINE ( 'NONE', #2668, #7786 ) ;
#21531=CARTESIAN_POINT ( 'NONE',  ( 34.50000000000001421, 3.245314017740485962E-16, 2.649999999999999911 ) ) ;
#21535=CARTESIAN_POINT ( 'NONE',  ( 46.99306361170634716, -4.271975761602691435, -0.9446694106403947799 ) ) ;
#21536=AXIS2_PLACEMENT_3D ( 'NONE', #18896, #2094, #6847 ) ;
#21537=CARTESIAN_POINT ( 'NONE',  ( -36.89831264271879263, 3.408535483610504180, 4.200031884472282151 ) ) ;
#21538=EDGE_CURVE ( 'NONE', #28113, #23361, #28504, .T. ) ;
#21541=FACE_OUTER_BOUND ( 'NONE', #9737, .T. ) ;
#21545=ORIENTED_EDGE ( 'NONE', *, *, #476, .F. ) ;
#21548=CIRCLE ( 'NONE', #3818, 0.09999999999999997780 ) ;
#21549=CARTESIAN_POINT ( 'NONE',  ( 15.29384114148387397, -3.378548217643446705, 3.972894518062632940 ) ) ;
#21550=CARTESIAN_POINT ( 'NONE',  ( 48.50000000000002132, 1.426739617975221641, -3.843750000000023093 ) ) ;
#21559=LINE ( 'NONE', #23299, #12460 ) ;
#21564=FACE_OUTER_BOUND ( 'NONE', #4376, .T. ) ;
#21565=FACE_OUTER_BOUND ( 'NONE', #2946, .T. ) ;
#21566=CARTESIAN_POINT ( 'NONE',  ( 15.81621483022863472, -5.330414537250523388, 0.9106291984478885881 ) ) ;
#21576=CARTESIAN_POINT ( 'NONE',  ( 58.50000000000001421, -0.8000000000000000444, 2.421260002560650104 ) ) ;
#21580=SURFACE_STYLE_USAGE ( .BOTH. , #24399 ) ;
#21590=DIRECTION ( 'NONE',  ( -2.459562394685737870E-16, 0.9510565162951500895, 0.3090169943749582204 ) ) ;
#21593=LINE ( 'NONE', #14127, #23068 ) ;
#21601=CYLINDRICAL_SURFACE ( 'NONE', #25579, 0.05000000000000012768 ) ;
#21602=DIRECTION ( 'NONE',  ( 0.000000000000000000, 0.000000000000000000, -1.000000000000000000 ) ) ;
#21606=AXIS2_PLACEMENT_3D ( 'NONE', #18143, #22570, #12734 ) ;
#21608=CARTESIAN_POINT ( 'NONE',  ( 50.35335635708054269, -1.310522848978943555, 3.864668279552718300 ) ) ;
#21615=ORIENTED_EDGE ( 'NONE', *, *, #1110, .T. ) ;
#21620=ORIENTED_EDGE ( 'NONE', *, *, #15827, .F. ) ;
#21621=CARTESIAN_POINT ( 'NONE',  ( 15.41217651307625225, 4.863043649742707863, 1.860644097022760013 ) ) ;
#21629=AXIS2_PLACEMENT_3D ( 'NONE', #20914, #9030, #4267 ) ;
#21648=FACE_OUTER_BOUND ( 'NONE', #19084, .T. ) ;
#21651=CIRCLE ( 'NONE', #15031, 0.05000000000000015543 ) ;
#21652=AXIS2_PLACEMENT_3D ( 'NONE', #3838, #13489, #23181 ) ;
#21658=DIRECTION ( 'NONE',  ( -1.000000000000000000, -2.586136946169074517E-16, 0.000000000000000000 ) ) ;
#21661=CARTESIAN_POINT ( 'NONE',  ( -36.11187263677869907, 2.734387802833793124, 4.440904455451962995 ) ) ;
#21672=EDGE_CURVE ( 'NONE', #14710, #4862, #29524, .T. ) ;
#21675=EDGE_CURVE ( 'NONE', #2569, #16545, #12327, .T. ) ;
#21677=DIRECTION ( 'NONE',  ( 0.000000000000000000, -1.000000000000000000, 0.000000000000000000 ) ) ;
#21680=FACE_OUTER_BOUND ( 'NONE', #28077, .T. ) ;
#21682=AXIS2_PLACEMENT_3D ( 'NONE', #9626, #1842, #16412 ) ;
#21691=ORIENTED_EDGE ( 'NONE', *, *, #9122, .T. ) ;
#21692=CARTESIAN_POINT ( 'NONE',  ( -54.44999999999997442, 1.499999999999999556, 4.029888335921975262 ) ) ;
#21695=CARTESIAN_POINT ( 'NONE',  ( 16.07279755198631932, 0.3252614978953071168, -5.399488438498867282 ) ) ;
#21700=CARTESIAN_POINT ( 'NONE',  ( -35.85663232820584057, 2.199885893005988358, -4.939696249117657700 ) ) ;
#21709=CARTESIAN_POINT ( 'NONE',  ( 15.03925126672133139, -3.817150320980655209, -2.203324261490558822 ) ) ;
#21714=CARTESIAN_POINT ( 'NONE',  ( 15.49676243306307022, -3.102491976071180879, 4.173461118157664629 ) ) ;
#21720=EDGE_CURVE ( 'NONE', #1101, #13576, #2702, .T. ) ;
#21724=CYLINDRICAL_SURFACE ( 'NONE', #17545, 1.000000000000000000 ) ;
#21731=CARTESIAN_POINT ( 'NONE',  ( -36.21152527658242093, 5.035245099686857628, 1.330662535294883098 ) ) ;
#21737=CARTESIAN_POINT ( 'NONE',  ( 54.40000000000001990, 0.000000000000000000, 0.000000000000000000 ) ) ;
#21738=DIRECTION ( 'NONE',  ( 2.085103575917242148E-15, -0.9615843008030771077, 0.2745098039215673746 ) ) ;
#21748=EDGE_LOOP ( 'NONE', ( #2654, #25784, #11518, #9163 ) ) ;
#21753=DIRECTION ( 'NONE',  ( -1.000000000000000000, -0.000000000000000000, -0.000000000000000000 ) ) ;
#21757=DIRECTION ( 'NONE',  ( -1.000000000000000000, -0.000000000000000000, -0.000000000000000000 ) ) ;
#21758=CARTESIAN_POINT ( 'NONE',  ( -36.77443515226921278, 0.6016956010319299830, -5.375730734456574567 ) ) ;
#21760=CARTESIAN_POINT ( 'NONE',  ( 47.00000000000002842, -4.144693941441892626, 1.074391609828098559 ) ) ;
#21762=CARTESIAN_POINT ( 'NONE',  ( 54.44364453144186911, -0.0003028757502672923879, -4.365665911209477557 ) ) ;
#21769=CARTESIAN_POINT ( 'NONE',  ( 48.29999997184167881, -0.7900353715960748424, 4.025797886239748991 ) ) ;
#21770=CARTESIAN_POINT ( 'NONE',  ( 48.50000000000002132, -1.391941090707485396, -3.850000000000022737 ) ) ;
#21779=ORIENTED_EDGE ( 'NONE', *, *, #9587, .F. ) ;
#21783=AXIS2_PLACEMENT_3D ( 'NONE', #18297, #10840, #1497 ) ;
#21784=FACE_OUTER_BOUND ( 'NONE', #5534, .T. ) ;
#21787=EDGE_LOOP ( 'NONE', ( #24633, #24840, #2694, #3081 ) ) ;
#21788=DIRECTION ( 'NONE',  ( -1.000000000000000000, 0.000000000000000000, -0.000000000000000000 ) ) ;
#21791=VERTEX_POINT ( 'NONE', #956 ) ;
#21794=CARTESIAN_POINT ( 'NONE',  ( -54.49999999999997868, -1.549598385535858380, 4.064203588144675194 ) ) ;
#21796=CARTESIAN_POINT ( 'NONE',  ( 56.98297952491088836, 0.7550874052942159187, 1.743526814789472912 ) ) ;
#21797=CARTESIAN_POINT ( 'NONE',  ( -36.68866260399460799, -3.738196885377723877, 3.908481927057712024 ) ) ;
#21810=CARTESIAN_POINT ( 'NONE',  ( 15.18459684427940104, 5.377732432866634049, 0.5657657256216265251 ) ) ;
#21814=CARTESIAN_POINT ( 'NONE',  ( -54.49999999999997868, 0.000000000000000000, 0.000000000000000000 ) ) ;
#21815=VERTEX_POINT ( 'NONE', #3162 ) ;
#21817=ADVANCED_FACE ( 'NONE', ( #17892 ), #8078, .F. ) ;
#21818=VERTEX_POINT ( 'NONE', #3632 ) ;
#21820=EDGE_LOOP ( 'NONE', ( #29953, #22148, #1658, #11067 ) ) ;
#21821=CIRCLE ( 'NONE', #30902, 1.000000000000000000 ) ;
#21822=CARTESIAN_POINT ( 'NONE',  ( 57.01079215475500206, -0.7500001437588036390, 1.746008375800299772 ) ) ;
#21829=DIRECTION ( 'NONE',  ( 0.000000000000000000, 0.000000000000000000, 1.000000000000000000 ) ) ;
#21830=CARTESIAN_POINT ( 'NONE',  ( 50.35335635708054980, 1.310522848978987298, -3.864668279552719632 ) ) ;
#21831=AXIS2_PLACEMENT_3D ( 'NONE', #7537, #26525, #29062 ) ;
#21833=B_SPLINE_CURVE_WITH_KNOTS ( 'NONE', 3,
 ( #28635, #12163, #26094, #4408, #21845, #9784, #29096, #7410, #23738, #2029, #17086, #31000, #18984, #26258, #16767, #6951 ),
 .UNSPECIFIED., .F., .F.,
 ( 4, 2, 2, 2, 2, 2, 2, 4 ),
 ( 0.000000000000000000, 0.0004351083927046443789, 0.0008702167854092887579, 0.001740433570818577516, 0.002175541963523222166, 0.002610650356227867466, 0.003045758748932512333, 0.003480867141637158067 ),
 .UNSPECIFIED. ) ;
#21836=EDGE_CURVE ( 'NONE', #7967, #3082, #24980, .T. ) ;
#21840=CARTESIAN_POINT ( 'NONE',  ( 57.00000000000000711, -0.7137254901960808917, -2.500119182088006209 ) ) ;
#21841=CARTESIAN_POINT ( 'NONE',  ( -36.58413561666738900, -3.095036031508881180, -4.435288302043747244 ) ) ;
#21845=CARTESIAN_POINT ( 'NONE',  ( -36.52679053911622731, -5.349174094756211417, 0.7986533162260726071 ) ) ;
#21847=CARTESIAN_POINT ( 'NONE',  ( -36.76447480099743359, -4.924630501335189869, 2.234249019593649077 ) ) ;
#21851=DIRECTION ( 'NONE',  ( 1.000000000000000000, 4.678365685400771632E-16, 1.520093157366894206E-16 ) ) ;
#21852=DIRECTION ( 'NONE',  ( -0.000000000000000000, -1.000000000000000000, 0.000000000000000000 ) ) ;
#21854=DIRECTION ( 'NONE',  ( -1.000000000000000000, -2.586136946169074517E-16, 0.000000000000000000 ) ) ;
#21858=FACE_OUTER_BOUND ( 'NONE', #27787, .T. ) ;
#21859=CARTESIAN_POINT ( 'NONE',  ( 58.45000000000001705, 0.000000000000000000, 0.000000000000000000 ) ) ;
#21860=CYLINDRICAL_SURFACE ( 'NONE', #24977, 4.300000000000019362 ) ;
#21864=DIRECTION ( 'NONE',  ( 0.000000000000000000, 1.000000000000000000, 0.000000000000000000 ) ) ;
#21876=CARTESIAN_POINT ( 'NONE',  ( -35.85663232820583346, -3.817150320980672529, -2.203324261490544611 ) ) ;
#21877=ORIENTED_EDGE ( 'NONE', *, *, #12678, .T. ) ;
#21881=PLANE ( 'NONE',  #28804 ) ;
#21882=DIRECTION ( 'NONE',  ( 1.000000000000000000, -0.000000000000000000, -0.000000000000000000 ) ) ;
#21884=ORIENTED_EDGE ( 'NONE', *, *, #7036, .T. ) ;
#21886=ORIENTED_EDGE ( 'NONE', *, *, #5340, .F. ) ;
#21887=CARTESIAN_POINT ( 'NONE',  ( 51.71308018800799289, -4.178911716362186723, 1.000646358242007983 ) ) ;
#21891=CARTESIAN_POINT ( 'NONE',  ( -35.85663232820581214, -5.086913985776156721, -1.171642053949115914 ) ) ;
#21893=FILL_AREA_STYLE ('',( #31049 ) ) ;
#21900=EDGE_CURVE ( 'NONE', #11230, #23664, #28161, .T. ) ;
#21907=FACE_OUTER_BOUND ( 'NONE', #18985, .T. ) ;
#21912=CARTESIAN_POINT ( 'NONE',  ( 48.46953526341861362, 1.366509374015061784, -3.854674997130605352 ) ) ;
#21913=CARTESIAN_POINT ( 'NONE',  ( 15.22842924604222503, 4.861582136949903266, -2.394243986685391512 ) ) ;
#21914=CARTESIAN_POINT ( 'NONE',  ( 57.03820272507597622, -0.7500000014582769436, 2.490438835250821992 ) ) ;
#21916=ORIENTED_EDGE ( 'NONE', *, *, #20855, .T. ) ;
#21917=CARTESIAN_POINT ( 'NONE',  ( 36.55000000000001847, 0.000000000000000000, 0.000000000000000000 ) ) ;
#21918=CARTESIAN_POINT ( 'NONE',  ( -36.00201293083839005, -5.377732432866788592, -0.5657657256210414376 ) ) ;
#21919=CARTESIAN_POINT ( 'NONE',  ( 48.45103168306561514, -1.383117500626934282, 3.859810431918025309 ) ) ;
#21922=ORIENTED_EDGE ( 'NONE', *, *, #25669, .F. ) ;
#21928=CARTESIAN_POINT ( 'NONE',  ( 15.87128154250932610, 5.321612844166258682, 0.9647713018063041046 ) ) ;
#21929=ORIENTED_EDGE ( 'NONE', *, *, #1489, .F. ) ;
#21930=CARTESIAN_POINT ( 'NONE',  ( 47.10000000000002274, -3.726179070414207928, -1.000000000000000000 ) ) ;
#21935=CARTESIAN_POINT ( 'NONE',  ( 51.80000000000001847, 1.734723475976807094E-15, -4.275000000000000355 ) ) ;
#21943=CARTESIAN_POINT ( 'NONE',  ( 57.03405126743467690, -0.7473881623357462312, 2.422979693216943176 ) ) ;
#21944=( BOUNDED_SURFACE ( )  B_SPLINE_SURFACE ( 3, 2, ( 
 ( #14852, #19788, #7732 ),
 ( #23910, #26436, #29121 ),
 ( #28965, #7593, #21549 ),
 ( #17394, #5058, #4729 ),
 ( #14239, #27041, #14390 ),
 ( #2684, #16942, #9970 ),
 ( #12040, #19328, #2538 ),
 ( #19642, #24513, #2827 ),
 ( #9521, #24062, #21714 ),
 ( #19180, #3, #7273 ),
 ( #26587, #12185, #5834 ),
 ( #29898, #17726, #22322 ),
 ( #2994, #12637, #22797 ),
 ( #10589, #17565, #27214 ),
 ( #15494, #22938, #8521 ),
 ( #30040, #8059, #3301 ) ),
 .UNSPECIFIED., .F., .F., .F. ) 
 B_SPLINE_SURFACE_WITH_KNOTS ( ( 4, 2, 2, 2, 2, 2, 2, 4 ),
 ( 3, 3 ),
 ( 0.001780502285214207499, 0.002558945925323793252, 0.002753556835351190016, 0.002948167745378586346, 0.003337389565433379439, 0.003726611385488172532, 0.004115833205542965625, 0.004894276845652550945 ),
 ( 0.000000000000000000, 1.000000000000000000 ),
 .UNSPECIFIED. ) 
 GEOMETRIC_REPRESENTATION_ITEM ( )  RATIONAL_B_SPLINE_SURFACE ( (
 ( 1.000000000000000000, 0.9418517008537220514, 1.000000000000000000),
 ( 1.000000000000000000, 0.9417987965885382673, 1.000000000000000000),
 ( 1.000000000000000000, 0.9418198861733636518, 1.000000000000000000),
 ( 1.000000000000000000, 0.9434060303845666073, 1.000000000000000000),
 ( 1.000000000000000000, 0.9437939819948258924, 1.000000000000000000),
 ( 1.000000000000000000, 0.9445989566712681418, 1.000000000000000000),
 ( 1.000000000000000000, 0.9450169930049783229, 1.000000000000000000),
 ( 1.000000000000000000, 0.9461610507673675619, 1.000000000000000000),
 ( 1.000000000000000000, 0.9467217966427196041, 1.000000000000000000),
 ( 1.000000000000000000, 0.9467345476124345849, 1.000000000000000000),
 ( 1.000000000000000000, 0.9461964028052562981, 1.000000000000000000),
 ( 1.000000000000000000, 0.9446801822474193422, 1.000000000000000000),
 ( 1.000000000000000000, 0.9437582546536890105, 1.000000000000000000),
 ( 1.000000000000000000, 0.9418129560294938862, 1.000000000000000000),
 ( 1.000000000000000000, 0.9418016889778016987, 1.000000000000000000),
 ( 1.000000000000000000, 0.9418517008537222734, 1.000000000000000000) ) ) 
 REPRESENTATION_ITEM ( '' )  SURFACE ( )  );
#21945=CARTESIAN_POINT ( 'NONE',  ( -36.43290890416756156, -3.561547362098786973, 4.076645242318810425 ) ) ;
#21951=ORIENTED_EDGE ( 'NONE', *, *, #7870, .F. ) ;
#21952=ORIENTED_EDGE ( 'NONE', *, *, #14724, .F. ) ;
#21953=CARTESIAN_POINT ( 'NONE',  ( 58.45000000000001705, 0.000000000000000000, 0.000000000000000000 ) ) ;
#21956=CARTESIAN_POINT ( 'NONE',  ( 51.80000000000001847, 2.428612866367529932E-14, 0.000000000000000000 ) ) ;
#21957=EDGE_LOOP ( 'NONE', ( #1867, #19090 ) ) ;
#21959=LINE ( 'NONE', #246, #27540 ) ;
#21964=VERTEX_POINT ( 'NONE', #30859 ) ;
#21965=CARTESIAN_POINT ( 'NONE',  ( -54.49999999999997868, 0.000000000000000000, -0.7500000000000001110 ) ) ;
#21967=EDGE_CURVE ( 'NONE', #5072, #22540, #6786, .T. ) ;
#21973=CARTESIAN_POINT ( 'NONE',  ( -36.11122220296834939, -3.378548217643453366, -3.972894518062632052 ) ) ;
#21974=CIRCLE ( 'NONE', #16349, 4.375000000000000000 ) ;
#21975=CARTESIAN_POINT ( 'NONE',  ( -54.49999999999997868, 0.000000000000000000, 4.349999999999997868 ) ) ;
#21976=VERTEX_POINT ( 'NONE', #30378 ) ;
#21977=CARTESIAN_POINT ( 'NONE',  ( 57.02185466405004632, -0.7499999999999981126, -2.421260014775926006 ) ) ;
#21979=CARTESIAN_POINT ( 'NONE',  ( 47.10000000000002274, 2.428612866367529932E-14, -1.100000000000000089 ) ) ;
#21984=CARTESIAN_POINT ( 'NONE',  ( 15.48609859788818355, 0.1138661108243574638, -5.199999999057642874 ) ) ;
#21986=CARTESIAN_POINT ( 'NONE',  ( -36.58413561666647951, -5.174628573245042773, 1.572974725650844174 ) ) ;
#21987=CARTESIAN_POINT ( 'NONE',  ( 48.46289871413547701, -1.426739617975173013, -3.843750000000023981 ) ) ;
#21989=ADVANCED_FACE ( 'NONE', ( #18679, #30229, #23744, #8830, #23273, #20597 ), #3943, .T. ) ;
#21991=CYLINDRICAL_SURFACE ( 'NONE', #12842, 0.05000000000000012768 ) ;
#21992=CARTESIAN_POINT ( 'NONE',  ( -45.15971931043468146, 0.000000000000000000, 0.000000000000000000 ) ) ;
#22000=ADVANCED_FACE ( 'NONE', ( #11218 ), #5789, .T. ) ;
#22002=LINE ( 'NONE', #14382, #2058 ) ;
#22003=CARTESIAN_POINT ( 'NONE',  ( -35.85663232820584057, -1.793057972834811054, 4.026191436120395650 ) ) ;
#22004=ADVANCED_FACE ( 'NONE', ( #15964 ), #6635, .F. ) ;
#22005=AXIS2_PLACEMENT_3D ( 'NONE', #26013, #18604, #27778 ) ;
#22008=AXIS2_PLACEMENT_3D ( 'NONE', #10500, #8119, #17787 ) ;
#22022=CARTESIAN_POINT ( 'NONE',  ( 57.02405634237670284, 0.7430569499193692140, -2.425812863566016997 ) ) ;
#22033=CARTESIAN_POINT ( 'NONE',  ( 50.30000000000001847, -1.426739617975173013, 3.843750000000023093 ) ) ;
#22035=CARTESIAN_POINT ( 'NONE',  ( -36.92362342067168868, -5.192953935288583622, -1.516181439821844279 ) ) ;
#22041=ORIENTED_EDGE ( 'NONE', *, *, #23398, .T. ) ;
#22043=CARTESIAN_POINT ( 'NONE',  ( 50.31874172786520916, 1.426739617975217866, 3.843750000000022649 ) ) ;
#22045=DIRECTION ( 'NONE',  ( 1.000000000000000000, 0.000000000000000000, 0.000000000000000000 ) ) ;
#22046=AXIS2_PLACEMENT_3D ( 'NONE', #15479, #10258, #14840 ) ;
#22048=CARTESIAN_POINT ( 'NONE',  ( 51.70000000000000995, -4.179189514726507682, -1.000000000000000000 ) ) ;
#22050=DIRECTION ( 'NONE',  ( 0.000000000000000000, 0.000000000000000000, 1.000000000000000000 ) ) ;
#22052=CARTESIAN_POINT ( 'NONE',  ( -36.30424252565905618, 0.1108756495952690768, -5.200000001675009642 ) ) ;
#22055=LINE ( 'NONE', #809, #8406 ) ;
#22057=CARTESIAN_POINT ( 'NONE',  ( 15.76623786017541562, 5.175840503946205651, -1.569056257078622618 ) ) ;
#22058=CARTESIAN_POINT ( 'NONE',  ( 57.02184386277451722, -0.7500000000000000000, 2.421260326253384942 ) ) ;
#22062=CARTESIAN_POINT ( 'NONE',  ( -36.92405921417685022, -5.187083072802368022, -1.534568794951191251 ) ) ;
#22066=EDGE_CURVE ( 'NONE', #19552, #28113, #21528, .T. ) ;
#22067=ORIENTED_EDGE ( 'NONE', *, *, #26088, .T. ) ;
#22069=EDGE_CURVE ( 'NONE', #12204, #8913, #26513, .T. ) ;
#22070=AXIS2_PLACEMENT_3D ( 'NONE', #25512, #17788, #29959 ) ;
#22077=CARTESIAN_POINT ( 'NONE',  ( 15.03925126672132784, 5.377732432866644707, -0.5657657256215208319 ) ) ;
#22078=ORIENTED_EDGE ( 'NONE', *, *, #5718, .T. ) ;
#22081=ORIENTED_EDGE ( 'NONE', *, *, #24035, .F. ) ;
#22087=ORIENTED_EDGE ( 'NONE', *, *, #11830, .T. ) ;
#22089=FACE_BOUND ( 'NONE', #22652, .T. ) ;
#22094=DIRECTION ( 'NONE',  ( 1.000000000000000000, 2.586136946169074517E-16, -0.000000000000000000 ) ) ;
#22095=CARTESIAN_POINT ( 'NONE',  ( 57.00000000000001421, 0.7058179832143345322, 2.448718171069995009 ) ) ;
#22098=CARTESIAN_POINT ( 'NONE',  ( 51.80000000000001847, -3.726179070414207928, 1.000000000000002220 ) ) ;
#22099=VECTOR ( 'NONE', #25659, 1000.000000000000000 ) ;
#22106=CIRCLE ( 'NONE', #12470, 4.375000000000000000 ) ;
#22108=ADVANCED_FACE ( 'NONE', ( #4879 ), #21991, .T. ) ;
#22110=ORIENTED_EDGE ( 'NONE', *, *, #25338, .T. ) ;
#22121=ORIENTED_EDGE ( 'NONE', *, *, #4707, .T. ) ;
#22125=DIRECTION ( 'NONE',  ( 0.000000000000000000, -1.000000000000000000, 0.000000000000000000 ) ) ;
#22126=AXIS2_PLACEMENT_3D ( 'NONE', #10403, #20245, #29262 ) ;
#22128=CIRCLE ( 'NONE', #20612, 0.05000000000000012768 ) ;
#22135=CARTESIAN_POINT ( 'NONE',  ( 15.59140265158956140, -4.755985070912263524, -2.573747172434730945 ) ) ;
#22136=B_SPLINE_CURVE_WITH_KNOTS ( 'NONE', 3,
 ( #24574, #12843, #20169, #3365, #5735, #26809, #22525, #29800, #27107, #17783, #12382, #29335, #27424, #5428, #2897, #3052 ),
 .UNSPECIFIED., .F., .F.,
 ( 4, 2, 2, 2, 2, 2, 2, 4 ),
 ( 1.734723475976807094E-18, 0.0004351083927046432947, 0.0008702167854092848548, 0.001740433570818574914, 0.002175541963523219997, 0.002610650356227864864, 0.003045758748932510165, 0.003480867141637155032 ),
 .UNSPECIFIED. ) ;
#22139=AXIS2_PLACEMENT_3D ( 'NONE', #446, #7582, #10109 ) ;
#22141=AXIS2_PLACEMENT_3D ( 'NONE', #18996, #18841, #14066 ) ;
#22144=ORIENTED_EDGE ( 'NONE', *, *, #20656, .F. ) ;
#22146=CARTESIAN_POINT ( 'NONE',  ( 50.50000000000002132, 0.6462379109121000331, -4.048750000000023164 ) ) ;
#22148=ORIENTED_EDGE ( 'NONE', *, *, #24908, .F. ) ;
#22150=CARTESIAN_POINT ( 'NONE',  ( -35.85663232820581214, -4.804073783693462829, 2.042134687550346772 ) ) ;
#22152=DIRECTION ( 'NONE',  ( 1.000000000000000000, 0.000000000000000000, 0.000000000000000000 ) ) ;
#22156=DIRECTION ( 'NONE',  ( 1.000000000000000000, 2.586136946169074517E-16, -0.000000000000000000 ) ) ;
#22159=DIRECTION ( 'NONE',  ( 0.000000000000000000, 0.000000000000000000, 1.000000000000000000 ) ) ;
#22165=DIRECTION ( 'NONE',  ( 0.000000000000000000, 0.000000000000000000, -1.000000000000000000 ) ) ;
#22172=DIRECTION ( 'NONE',  ( 0.000000000000000000, 0.000000000000000000, -1.000000000000000000 ) ) ;
#22173=CARTESIAN_POINT ( 'NONE',  ( 15.03925126672132961, 1.123735532908280765, -5.289358697221546279 ) ) ;
#22183=DIRECTION ( 'NONE',  ( 1.000000000000000000, 0.000000000000000000, 0.000000000000000000 ) ) ;
#22184=CARTESIAN_POINT ( 'NONE',  ( 15.17256654081423051, -3.426725948577732606, -3.937891352654259602 ) ) ;
#22187=EDGE_CURVE ( 'NONE', #4123, #23938, #26999, .T. ) ;
#22188=ORIENTED_EDGE ( 'NONE', *, *, #6628, .T. ) ;
#22190=ORIENTED_EDGE ( 'NONE', *, *, #19685, .T. ) ;
#22195=CARTESIAN_POINT ( 'NONE',  ( 56.95000000000001705, -0.6820512820512817376, -1.773360101234997988 ) ) ;
#22196=CARTESIAN_POINT ( 'NONE',  ( 50.34665981758797670, 1.329038565861465848, 3.861394075523872260 ) ) ;
#22197=CARTESIAN_POINT ( 'NONE',  ( -36.89017861347080185, -5.235729994560249345, -1.359191621353769142 ) ) ;
#22202=ORIENTED_EDGE ( 'NONE', *, *, #7933, .T. ) ;
#22204=CARTESIAN_POINT ( 'NONE',  ( 50.46999119548826940, 1.140870969100562293, 3.938727831757874664 ) ) ;
#22205=CARTESIAN_POINT ( 'NONE',  ( 48.39328721529930277, -1.343285922954026379, -3.873819829599202791 ) ) ;
#22206=CARTESIAN_POINT ( 'NONE',  ( -54.46462222424374033, -1.502185874895794138, 3.301501926143236343 ) ) ;
#22207=EDGE_CURVE ( 'NONE', #28800, #21494, #28017, .T. ) ;
#22214=DIRECTION ( 'NONE',  ( 0.000000000000000000, -0.2573099415204678775, 0.9663289263986324373 ) ) ;
#22216=CARTESIAN_POINT ( 'NONE',  ( 15.74652664997094575, 5.076023720898220404, -1.868859051106881664 ) ) ;
#22223=CARTESIAN_POINT ( 'NONE',  ( 15.41170998834797246, 2.595074437874858031, -4.757608386865152639 ) ) ;
#22224=FACE_OUTER_BOUND ( 'NONE', #12103, .T. ) ;
#22226=EDGE_CURVE ( 'NONE', #3125, #17229, #14997, .T. ) ;
#22244=FACE_OUTER_BOUND ( 'NONE', #27165, .T. ) ;
#22258=CARTESIAN_POINT ( 'NONE',  ( -54.49998431799114940, 1.548747819918198987, -3.331336553795240185 ) ) ;
#22262=AXIS2_PLACEMENT_3D ( 'NONE', #10180, #1001, #27431 ) ;
#22263=EDGE_LOOP ( 'NONE', ( #17393, #18299, #26679 ) ) ;
#22286=EDGE_CURVE ( 'NONE', #20389, #18736, #28036, .T. ) ;
#22289=CARTESIAN_POINT ( 'NONE',  ( 48.30000000000001847, 0.6304760106459513791, -3.950000000000021938 ) ) ;
#22290=DIRECTION ( 'NONE',  ( 0.000000000000000000, 0.000000000000000000, -1.000000000000000000 ) ) ;
#22298=EDGE_CURVE ( 'NONE', #20361, #23664, #18459, .T. ) ;
#22299=CARTESIAN_POINT ( 'NONE',  ( 50.46977479615469520, 1.142230555601122965, -3.938343097974785767 ) ) ;
#22303=CARTESIAN_POINT ( 'NONE',  ( 48.50000000000002132, -1.426739617975173013, -3.843750000000023093 ) ) ;
#22304=EDGE_LOOP ( 'NONE', ( #16011, #12016, #29094, #14011 ) ) ;
#22306=CIRCLE ( 'NONE', #2572, 1.949999999999999956 ) ;
#22308=ORIENTED_EDGE ( 'NONE', *, *, #9624, .T. ) ;
#22311=DIRECTION ( 'NONE',  ( 0.000000000000000000, -1.000000000000000000, 0.000000000000000000 ) ) ;
#22318=CARTESIAN_POINT ( 'NONE',  ( 15.18463186935387554, -1.123735532908824997, 5.289358697221508976 ) ) ;
#22319=EDGE_LOOP ( 'NONE', ( #4877, #12740, #8432, #1203, #21374, #10950, #12699, #6566, #8223, #29635, #25718, #16664, #29637, #12448, #8921, #18992, #4053 ) ) ;
#22322=CARTESIAN_POINT ( 'NONE',  ( 15.44631504820161005, -2.881190829692224398, 4.334245811858097319 ) ) ;
#22325=CARTESIAN_POINT ( 'NONE',  ( -36.11692583559843683, 4.683225668088560667, -2.703237747137714919 ) ) ;
#22330=DIRECTION ( 'NONE',  ( 1.000000000000000000, 2.586136946169074517E-16, -0.000000000000000000 ) ) ;
#22331=EDGE_LOOP ( 'NONE', ( #15197, #10369, #22087, #20689 ) ) ;
#22338=VECTOR ( 'NONE', #3576, 1000.000000000000000 ) ;
#22348=CIRCLE ( 'NONE', #30932, 4.275000000000000355 ) ;
#22352=CARTESIAN_POINT ( 'NONE',  ( 15.41080140630216988, -0.6967302926296836674, 5.374298406429148578 ) ) ;
#22354=VECTOR ( 'NONE', #13424, 1000.000000000000000 ) ;
#22359=CARTESIAN_POINT ( 'NONE',  ( 58.50000000000001421, 0.8000000000000000444, -2.489477856900920383 ) ) ;
#22361=CARTESIAN_POINT ( 'NONE',  ( 54.45370770736469268, -0.0004837498569171640238, -4.360091688067994298 ) ) ;
#22362=CARTESIAN_POINT ( 'NONE',  ( 57.00000000000001421, -0.7137254901960804476, 2.500119182088006209 ) ) ;
#22365=CARTESIAN_POINT ( 'NONE',  ( 50.32838854698020725, -1.409900272549264644, -3.850000494969507248 ) ) ;
#22369=DIRECTION ( 'NONE',  ( 0.000000000000000000, 0.000000000000000000, -1.000000000000000000 ) ) ;
#22370=VERTEX_POINT ( 'NONE', #28446 ) ;
#22377=ORIENTED_EDGE ( 'NONE', *, *, #13610, .F. ) ;
#22378=CARTESIAN_POINT ( 'NONE',  ( 15.97944027357901042, 5.289443499204828925, -1.131445731060737980 ) ) ;
#22384=VERTEX_POINT ( 'NONE', #13706 ) ;
#22389=CARTESIAN_POINT ( 'NONE',  ( 51.79694101351947211, -4.143816080048276618, -1.075455348895917984 ) ) ;
#22390=ADVANCED_FACE ( 'NONE', ( #4211 ), #1672, .T. ) ;
#22391=CARTESIAN_POINT ( 'NONE',  ( -54.46439202372638277, -1.502116081466616793, 4.031358338852112588 ) ) ;
#22395=EDGE_CURVE ( 'NONE', #22708, #14986, #1838, .T. ) ;
#22396=CARTESIAN_POINT ( 'NONE',  ( 57.00174889577907322, -0.7131084301676396953, 2.444403622924161912 ) ) ;
#22397=CARTESIAN_POINT ( 'NONE',  ( -36.92443669619772351, -3.305069970238164956, 4.282766538619550367 ) ) ;
#22399=CARTESIAN_POINT ( 'NONE',  ( 50.50000000000002132, -0.7900853852131047850, -4.025789903357282817 ) ) ;
#22401=B_SPLINE_CURVE_WITH_KNOTS ( 'NONE', 3,
 ( #1851, #9151, #18812, #23871, #25238, #3557, #6090, #15741, #27922, #16055, #28071, #13194, #13506, #20964, #11137, #6390 ),
 .UNSPECIFIED., .F., .F.,
 ( 4, 2, 2, 2, 2, 2, 2, 4 ),
 ( 0.000000000000000000, 0.0004351083927046427526, 0.0008702167854092855053, 0.001740433570818570794, 0.002175541963523213926, 0.002610650356227856624, 0.003045758748932499323, 0.003480867141637142021 ),
 .UNSPECIFIED. ) ;
#22404=CARTESIAN_POINT ( 'NONE',  ( -54.46462222424374033, 1.502185874895793694, 3.301501926143237675 ) ) ;
#22406=ORIENTED_EDGE ( 'NONE', *, *, #2137, .F. ) ;
#22410=DIRECTION ( 'NONE',  ( 0.000000000000000000, 0.000000000000000000, 1.000000000000000000 ) ) ;
#22412=ADVANCED_FACE ( 'NONE', ( #30653 ), #22921, .T. ) ;
#22423=CARTESIAN_POINT ( 'NONE',  ( 15.03925126672126034, -4.861582140531611529, -2.394243978978356502 ) ) ;
#22430=DIRECTION ( 'NONE',  ( 0.000000000000000000, -1.000000000000000000, 0.000000000000000000 ) ) ;
#22431=CARTESIAN_POINT ( 'NONE',  ( 50.30000000000001847, 1.426739617975228525, -3.843750000000022649 ) ) ;
#22432=AXIS2_PLACEMENT_3D ( 'NONE', #17735, #22330, #15337 ) ;
#22438=CARTESIAN_POINT ( 'NONE',  ( -36.89017861347172555, -3.436881753486550561, -4.177093996075186055 ) ) ;
#22451=ADVANCED_FACE ( 'NONE', ( #14021 ), #7377, .T. ) ;
#22452=CARTESIAN_POINT ( 'NONE',  ( 57.00074754615238248, -0.7099475343046129927, -1.812279303590036639 ) ) ;
#22455=CARTESIAN_POINT ( 'NONE',  ( -54.47710365256552478, -1.507983431629474014, -4.035431478432994545 ) ) ;
#22456=ORIENTED_EDGE ( 'NONE', *, *, #27340, .F. ) ;
#22466=CARTESIAN_POINT ( 'NONE',  ( 15.03925126672127810, 2.686240680702102868, 4.475885388010754085 ) ) ;
#22469=CARTESIAN_POINT ( 'NONE',  ( 51.90000000000001990, -4.241638912518127746, 1.073342218585537466 ) ) ;
#22472=CARTESIAN_POINT ( 'NONE',  ( -35.85663232820581214, 0.7747498368337695229, 5.363501452440937456 ) ) ;
#22474=EDGE_LOOP ( 'NONE', ( #24325, #548, #30791, #28839, #24253, #9985, #8154, #1630, #23624, #19126 ) ) ;
#22480=CARTESIAN_POINT ( 'NONE',  ( 57.02888566337306031, 0.7456496514153734267, -2.424120212325347357 ) ) ;
#22481=CARTESIAN_POINT ( 'NONE',  ( -54.44999999999997442, 0.000000000000000000, 0.000000000000000000 ) ) ;
#22486=DIRECTION ( 'NONE',  ( 0.000000000000000000, 0.000000000000000000, 1.000000000000000000 ) ) ;
#22492=CIRCLE ( 'NONE', #13370, 0.4576450603546982632 ) ;
#22500=CIRCLE ( 'NONE', #25010, 1.000000000000000000 ) ;
#22516=CARTESIAN_POINT ( 'NONE',  ( 15.41217651307625580, 3.272340825137240117, -4.050058705652119784 ) ) ;
#22518=CARTESIAN_POINT ( 'NONE',  ( 15.56274145962647104, -5.369990034204302098, 0.6654225812208781621 ) ) ;
#22521=CARTESIAN_POINT ( 'NONE',  ( 47.00101556927586444, -4.139722501993201575, 1.083525984490929961 ) ) ;
#22525=CARTESIAN_POINT ( 'NONE',  ( 16.10660252424456829, -5.053896291911978977, 1.944420249220634833 ) ) ;
#22526=ORIENTED_EDGE ( 'NONE', *, *, #23161, .T. ) ;
#22530=ORIENTED_EDGE ( 'NONE', *, *, #5323, .T. ) ;
#22536=DIRECTION ( 'NONE',  ( -0.000000000000000000, 0.000000000000000000, 1.000000000000000000 ) ) ;
#22540=VERTEX_POINT ( 'NONE', #18957 ) ;
#22541=AXIS2_PLACEMENT_3D ( 'NONE', #31245, #28870, #7181 ) ;
#22542=EDGE_CURVE ( 'NONE', #30886, #15970, #21959, .T. ) ;
#22543=CARTESIAN_POINT ( 'NONE',  ( 51.77770663993858591, -4.163003037071927537, -1.036150823695777934 ) ) ;
#22546=CARTESIAN_POINT ( 'NONE',  ( 57.00914817631336717, -0.7715555436188452632, -1.736293111776144205 ) ) ;
#22557=CARTESIAN_POINT ( 'NONE',  ( 48.30000000000001847, -0.7900853852131047850, 4.025789903357282817 ) ) ;
#22563=EDGE_CURVE ( 'NONE', #3627, #2662, #13872, .T. ) ;
#22564=AXIS2_PLACEMENT_3D ( 'NONE', #10056, #2925, #2617 ) ;
#22565=ORIENTED_EDGE ( 'NONE', *, *, #10739, .T. ) ;
#22570=DIRECTION ( 'NONE',  ( 1.000000000000000000, 0.000000000000000000, 0.000000000000000000 ) ) ;
#22572=ORIENTED_EDGE ( 'NONE', *, *, #14704, .T. ) ;
#22574=ORIENTED_EDGE ( 'NONE', *, *, #27628, .T. ) ;
#22578=CIRCLE ( 'NONE', #2852, 4.100000000000022737 ) ;
#22579=( BOUNDED_SURFACE ( )  B_SPLINE_SURFACE ( 3, 2, ( 
 ( #8414, #13457, #6200 ),
 ( #25499, #18395, #28030 ),
 ( #22518, #9210, #13926 ),
 ( #21566, #4129, #11249 ),
 ( #4450, #11736, #28684 ),
 ( #18871, #1739, #8866 ),
 ( #16173, #6998, #20927 ),
 ( #14259, #1588, #7148 ),
 ( #9044, #13766, #21263 ),
 ( #31210, #23779, #11409 ),
 ( #2221, #11582, #6817 ),
 ( #28205, #30894, #30558 ),
 ( #16811, #23623, #19198 ),
 ( #6666, #16660, #28837 ),
 ( #26452, #23929, #26301 ),
 ( #11885, #4602, #9538 ) ),
 .UNSPECIFIED., .F., .F., .F. ) 
 B_SPLINE_SURFACE_WITH_KNOTS ( ( 4, 2, 2, 2, 2, 2, 2, 4 ),
 ( 3, 3 ),
 ( 0.001780502285214212487, 0.002558945925323800191, 0.002753556835351196955, 0.002948167745378593718, 0.003337389565433387679, 0.003726611385488181639, 0.004115833205542975166, 0.004894276845652563088 ),
 ( 0.000000000000000000, 1.000000000000000000 ),
 .UNSPECIFIED. ) 
 GEOMETRIC_REPRESENTATION_ITEM ( )  RATIONAL_B_SPLINE_SURFACE ( (
 ( 1.000000000000000000, 0.9418517008537223845, 1.000000000000000000),
 ( 1.000000000000000000, 0.9417987965885161739, 1.000000000000000000),
 ( 1.000000000000000000, 0.9418198861733920735, 1.000000000000000000),
 ( 1.000000000000000000, 0.9434060303845589468, 1.000000000000000000),
 ( 1.000000000000000000, 0.9437939819948110154, 1.000000000000000000),
 ( 1.000000000000000000, 0.9445989566712821306, 1.000000000000000000),
 ( 1.000000000000000000, 0.9450169930049815425, 1.000000000000000000),
 ( 1.000000000000000000, 0.9461610507673599013, 1.000000000000000000),
 ( 1.000000000000000000, 0.9467217966427268205, 1.000000000000000000),
 ( 1.000000000000000000, 0.9467345476124273684, 1.000000000000000000),
 ( 1.000000000000000000, 0.9461964028052485265, 1.000000000000000000),
 ( 1.000000000000000000, 0.9446801822474260035, 1.000000000000000000),
 ( 1.000000000000000000, 0.9437582546536592565, 1.000000000000000000),
 ( 1.000000000000000000, 0.9418129560295517289, 1.000000000000000000),
 ( 1.000000000000000000, 0.9418016889777567346, 1.000000000000000000),
 ( 1.000000000000000000, 0.9418517008537217183, 1.000000000000000000) ) ) 
 REPRESENTATION_ITEM ( '' )  SURFACE ( )  );
#22584=DIRECTION ( 'NONE',  ( 1.000000000000000000, 0.000000000000000000, 0.000000000000000000 ) ) ;
#22585=ADVANCED_FACE ( 'NONE', ( #9457 ), #19124, .F. ) ;
#22594=LINE ( 'NONE', #573, #31180 ) ;
#22602=DIRECTION ( 'NONE',  ( 0.000000000000000000, 1.000000000000000000, 0.000000000000000000 ) ) ;
#22603=VECTOR ( 'NONE', #28343, 1000.000000000000000 ) ;
#22613=DIRECTION ( 'NONE',  ( -1.000000000000000000, 0.000000000000000000, 0.000000000000000000 ) ) ;
#22619=ORIENTED_EDGE ( 'NONE', *, *, #30372, .T. ) ;
#22624=ORIENTED_EDGE ( 'NONE', *, *, #4116, .F. ) ;
#22636=AXIS2_PLACEMENT_3D ( 'NONE', #3437, #30329, #13075 ) ;
#22637=CIRCLE ( 'NONE', #1861, 3.625000000000000444 ) ;
#22640=CARTESIAN_POINT ( 'NONE',  ( 15.98305126557428224, 2.728070298465770982, 4.669343935538297963 ) ) ;
#22641=AXIS2_PLACEMENT_3D ( 'NONE', #13095, #23084, #3460 ) ;
#22643=CIRCLE ( 'NONE', #8967, 1.000000000000000000 ) ;
#22646=AXIS2_PLACEMENT_3D ( 'NONE', #27989, #28151, #6774 ) ;
#22651=CARTESIAN_POINT ( 'NONE',  ( 48.43920370478603843, 1.278211010209494347, -3.870212229389975889 ) ) ;
#22652=EDGE_LOOP ( 'NONE', ( #20724, #28 ) ) ;
#22653=CIRCLE ( 'NONE', #30201, 1.000000000000000000 ) ;
#22656=EDGE_LOOP ( 'NONE', ( #16485, #11864, #12794, #11674, #14313, #5523, #250 ) ) ;
#22660=ORIENTED_EDGE ( 'NONE', *, *, #12285, .T. ) ;
#22663=EDGE_LOOP ( 'NONE', ( #17140, #16015, #17502, #23408 ) ) ;
#22668=CARTESIAN_POINT ( 'NONE',  ( 51.90000000000001279, 1.029992063861229212E-15, -4.375000000000002665 ) ) ;
#22672=CIRCLE ( 'NONE', #27688, 1.000000000000000000 ) ;
#22676=CARTESIAN_POINT ( 'NONE',  ( 48.46709009337374141, -1.365599538210734876, -3.854893000251051749 ) ) ;
#22677=CARTESIAN_POINT ( 'NONE',  ( 15.03925126672132961, 1.123735532908287427, 5.289358697221544503 ) ) ;
#22678=EDGE_CURVE ( 'NONE', #10038, #12845, #17426, .T. ) ;
#22692=CARTESIAN_POINT ( 'NONE',  ( 15.41586008885047576, 2.840672495176553625, -4.363684107482565189 ) ) ;
#22702=EDGE_LOOP ( 'NONE', ( #26064, #774, #25618, #18113 ) ) ;
#22706=DIRECTION ( 'NONE',  ( 1.000000000000000000, 0.000000000000000000, 0.000000000000000000 ) ) ;
#22708=VERTEX_POINT ( 'NONE', #16222 ) ;
#22709=CARTESIAN_POINT ( 'NONE',  ( 56.97512559646294505, 0.7466375667864569854, -1.747149777169433094 ) ) ;
#22716=CARTESIAN_POINT ( 'NONE',  ( 48.40000000000001990, -4.899999999999999467, -4.100000000000022737 ) ) ;
#22717=CARTESIAN_POINT ( 'NONE',  ( 46.90000000000001279, 1.734723475976807094E-15, -4.375000000000000000 ) ) ;
#22721=DIRECTION ( 'NONE',  ( 1.000000000000000000, -1.165806029810671835E-15, -1.108125256279701864E-14 ) ) ;
#22723=DIRECTION ( 'NONE',  ( 0.000000000000000000, 0.000000000000000000, 1.000000000000000000 ) ) ;
#22726=CARTESIAN_POINT ( 'NONE',  ( -54.45495050826418293, 1.499999999999999556, -3.300094695611021312 ) ) ;
#22742=DIRECTION ( 'NONE',  ( 1.000000000000000000, -0.000000000000000000, -0.000000000000000000 ) ) ;
#22748=CARTESIAN_POINT ( 'NONE',  ( 33.47623932017462778, -4.018128179617539431, 3.618665901676652918 ) ) ;
#22753=VECTOR ( 'NONE', #10572, 1000.000000000000000 ) ;
#22757=DIRECTION ( 'NONE',  ( 0.000000000000000000, 1.224646799147358384E-16, 1.000000000000000000 ) ) ;
#22763=CARTESIAN_POINT ( 'NONE',  ( -36.00201293083839005, 1.123735532908824331, 5.289358697221505423 ) ) ;
#22765=B_SPLINE_CURVE_WITH_KNOTS ( 'NONE', 3,
 ( #1302, #30115, #22867, #24902, #5921, #7984, #17804, #3222, #6078, #11124, #13181, #22546, #1155, #850, #17947, #1464 ),
 .UNSPECIFIED., .F., .F.,
 ( 4, 3, 3, 3, 3, 4 ),
 ( 0.000000000000000000, 3.111139534546023401E-05, 6.583698738123831937E-05, 9.811465807641186142E-05, 0.0001294159172546408877, 0.0001609582457662007114 ),
 .UNSPECIFIED. ) ;
#22772=ORIENTED_EDGE ( 'NONE', *, *, #11720, .F. ) ;
#22773=DIRECTION ( 'NONE',  ( 0.000000000000000000, 0.000000000000000000, 1.000000000000000000 ) ) ;
#22776=LINE ( 'NONE', #23075, #15668 ) ;
#22777=VERTEX_POINT ( 'NONE', #18444 ) ;
#22783=CARTESIAN_POINT ( 'NONE',  ( 58.45000000000001705, 0.8000000000000000444, -1.778341924377873751 ) ) ;
#22784=CARTESIAN_POINT ( 'NONE',  ( 47.10000000000002274, 2.260045634542508431E-14, 1.100000000000006084 ) ) ;
#22785=ORIENTED_EDGE ( 'NONE', *, *, #15081, .F. ) ;
#22787=CIRCLE ( 'NONE', #13143, 0.09999999999999982514 ) ;
#22788=CARTESIAN_POINT ( 'NONE',  ( -36.92443669619682112, 5.191204783933211608, -1.522159526382838246 ) ) ;
#22792=CARTESIAN_POINT ( 'NONE',  ( -54.49999999999997868, -1.549999999999999600, -3.332135201338624952 ) ) ;
#22793=DIRECTION ( 'NONE',  ( 1.857384214413941805E-31, -5.942513678379226626E-16, -1.000000000000000000 ) ) ;
#22794=DIRECTION ( 'NONE',  ( -0.000000000000000000, 0.000000000000000000, 1.000000000000000000 ) ) ;
#22797=CARTESIAN_POINT ( 'NONE',  ( 15.41586008885047221, -2.840672495176578938, 4.363684107482475483 ) ) ;
#22800=DIRECTION ( 'NONE',  ( 0.000000000000000000, -1.000000000000000000, 5.942513678379226626E-16 ) ) ;
#22802=DIRECTION ( 'NONE',  ( 1.000000000000000000, 0.000000000000000000, 0.000000000000000000 ) ) ;
#22805=AXIS2_PLACEMENT_3D ( 'NONE', #12316, #31183, #17249 ) ;
#22807=VERTEX_POINT ( 'NONE', #1331 ) ;
#22811=CARTESIAN_POINT ( 'NONE',  ( 48.30261087823118515, 0.9335627837658418970, 3.994936164801341061 ) ) ;
#22814=EDGE_LOOP ( 'NONE', ( #22886, #20510, #24176, #101 ) ) ;
#22830=CARTESIAN_POINT ( 'NONE',  ( 48.40000000000002700, -0.6462379109120522935, -4.048750000000028493 ) ) ;
#22831=CARTESIAN_POINT ( 'NONE',  ( 15.17256654081409373, 0.4576450652446744649, 5.200000002521306008 ) ) ;
#22834=CARTESIAN_POINT ( 'NONE',  ( -35.85663232820601820, 1.123735532908269441, -5.289358697221545391 ) ) ;
#22837=DIRECTION ( 'NONE',  ( -1.000000000000000000, -2.586136946169074517E-16, 0.000000000000000000 ) ) ;
#22842=CARTESIAN_POINT ( 'NONE',  ( 15.86395258069111769, 3.736273719777285507, -3.909490113446701720 ) ) ;
#22844=CARTESIAN_POINT ( 'NONE',  ( 57.05000000000001137, 0.8156862745098039102, 2.468735688885371982 ) ) ;
#22852=CARTESIAN_POINT ( 'NONE',  ( 16.10660252424456829, 2.945786441214607532, -4.543674732827721385 ) ) ;
#22860=CARTESIAN_POINT ( 'NONE',  ( 57.02478278053006022, 0.7769964508979760875, -1.733862565638740305 ) ) ;
#22861=ADVANCED_FACE ( 'NONE', ( #7043 ), #26347, .T. ) ;
#22867=CARTESIAN_POINT ( 'NONE',  ( 56.95150694030147775, -0.7014737422875408912, -1.765795469766037185 ) ) ;
#22869=ADVANCED_FACE ( 'NONE', ( #16705 ), #13670, .T. ) ;
#22873=CARTESIAN_POINT ( 'NONE',  ( -54.44999999999997442, 1.499999999999999556, -3.300094695611021312 ) ) ;
#22875=CIRCLE ( 'NONE', #9724, 2.600000000000000089 ) ;
#22886=ORIENTED_EDGE ( 'NONE', *, *, #10032, .T. ) ;
#22889=EDGE_CURVE ( 'NONE', #1787, #9517, #22913, .T. ) ;
#22891=ORIENTED_EDGE ( 'NONE', *, *, #25338, .F. ) ;
#22896=CARTESIAN_POINT ( 'NONE',  ( 47.00000000000002842, -4.144729964592912097, -1.074323956810995240 ) ) ;
#22899=CARTESIAN_POINT ( 'NONE',  ( 16.10667815269232506, 3.062358472872010129, 4.459001320275609359 ) ) ;
#22901=DIRECTION ( 'NONE',  ( 0.000000000000000000, 0.000000000000000000, -1.000000000000000000 ) ) ;
#22906=CARTESIAN_POINT ( 'NONE',  ( 58.50000000000001421, -0.8000000000000000444, 2.489477856900920383 ) ) ;
#22907=CARTESIAN_POINT ( 'NONE',  ( -36.40878371307407235, 0.9780988077348086174, 5.318542208600379517 ) ) ;
#22909=VECTOR ( 'NONE', #30778, 1000.000000000000000 ) ;
#22910=ORIENTED_EDGE ( 'NONE', *, *, #23601, .F. ) ;
#22913=B_SPLINE_CURVE_WITH_KNOTS ( 'NONE', 3,
 ( #2900, #7790, #12698, #9873, #7966, #3055, #831, #29192, #19845, #22378, #27427, #20172, #3203, #17630, #12386, #22077 ),
 .UNSPECIFIED., .F., .F.,
 ( 4, 2, 2, 2, 2, 2, 2, 4 ),
 ( 1.734723475976807094E-18, 0.0004351083927046410721, 0.0008702167854092804095, 0.001740433570818558434, 0.002175541963523197446, 0.002610650356227836241, 0.003045758748932475037, 0.003480867141637114266 ),
 .UNSPECIFIED. ) ;
#22919=ORIENTED_EDGE ( 'NONE', *, *, #7620, .T. ) ;
#22921=CYLINDRICAL_SURFACE ( 'NONE', #25006, 4.384222560975607585 ) ;
#22923=CARTESIAN_POINT ( 'NONE',  ( 47.00000000000002132, 2.428612866367529932E-14, 0.000000000000000000 ) ) ;
#22925=CARTESIAN_POINT ( 'NONE',  ( 57.05000000000001847, -0.6999999999999999556, 0.000000000000000000 ) ) ;
#22929=CARTESIAN_POINT ( 'NONE',  ( -36.30347965937239962, 4.910307320510253426, -1.715181477143334021 ) ) ;
#22932=CARTESIAN_POINT ( 'NONE',  ( 15.03925126672132961, 3.056483311920805690, 4.206888370749768846 ) ) ;
#22933=CIRCLE ( 'NONE', #24436, 4.100000000000022737 ) ;
#22935=TOROIDAL_SURFACE ( 'NONE', #25451, 3.675000000000029132, 0.05000000000000000278 ) ;
#22936=ORIENTED_EDGE ( 'NONE', *, *, #18830, .T. ) ;
#22938=CARTESIAN_POINT ( 'NONE',  ( 15.22842924604237069, -2.525801262579322248, 4.794550356815982184 ) ) ;
#22945=CARTESIAN_POINT ( 'NONE',  ( 48.47161145301956253, 1.409900272549317268, -3.850000494969540554 ) ) ;
#22946=ORIENTED_EDGE ( 'NONE', *, *, #2261, .F. ) ;
#22951=CARTESIAN_POINT ( 'NONE',  ( 48.34352038844360777, 1.212999249975939886, 3.917061424767716016 ) ) ;
#22955=AXIS2_PLACEMENT_3D ( 'NONE', #16397, #28587, #23522 ) ;
#22962=CARTESIAN_POINT ( 'NONE',  ( -35.85663232820592583, -4.804073783693453059, -2.042134687550363648 ) ) ;
#22965=ORIENTED_EDGE ( 'NONE', *, *, #30680, .T. ) ;
#22966=EDGE_CURVE ( 'NONE', #22370, #26302, #1255, .T. ) ;
#22967=CARTESIAN_POINT ( 'NONE',  ( 47.00000000000002132, -4.131056160354152240, -1.100000000000000089 ) ) ;
#22969=DIRECTION ( 'NONE',  ( 1.000000000000000000, 0.000000000000000000, 0.000000000000000000 ) ) ;
#22971=CARTESIAN_POINT ( 'NONE',  ( 15.66436536804551238, -0.4008586329626869782, 5.396496690166844523 ) ) ;
#22974=DIRECTION ( 'NONE',  ( 0.000000000000000000, 0.000000000000000000, 1.000000000000000000 ) ) ;
#22977=EDGE_CURVE ( 'NONE', #1571, #6093, #15389, .T. ) ;
#22988=CARTESIAN_POINT ( 'NONE',  ( 47.00000000000002132, -3.976179070414207928, 1.000000000000000000 ) ) ;
#22996=CARTESIAN_POINT ( 'NONE',  ( -54.44999999999997442, 0.000000000000000000, 0.000000000000000000 ) ) ;
#23005=VECTOR ( 'NONE', #12660, 1000.000000000000000 ) ;
#23013=CARTESIAN_POINT ( 'NONE',  ( 15.03925126672132784, 5.377732432866644707, -0.5657657256215208319 ) ) ;
#23016=VECTOR ( 'NONE', #6357, 1000.000000000000000 ) ;
#23017=EDGE_CURVE ( 'NONE', #24464, #15593, #3669, .T. ) ;
#23020=CARTESIAN_POINT ( 'NONE',  ( 48.30000000000001847, 0.6304760106459519342, 3.950000000000022826 ) ) ;
#23021=CARTESIAN_POINT ( 'NONE',  ( 56.96603746669009638, 0.7703957983921196906, 2.483260519405945388 ) ) ;
#23028=CARTESIAN_POINT ( 'NONE',  ( 50.38476904405314372, -1.115727354199205879, 3.895947837398489266 ) ) ;
#23030=( NAMED_UNIT ( * ) PLANE_ANGLE_UNIT ( ) SI_UNIT ( $, .RADIAN. ) );
#23036=AXIS2_PLACEMENT_3D ( 'NONE', #4626, #11912, #14284 ) ;
#23043=CARTESIAN_POINT ( 'NONE',  ( 58.45000000000001705, 0.8000000000000000444, -2.421260002560649660 ) ) ;
#23047=CARTESIAN_POINT ( 'NONE',  ( 47.10000000000002274, -4.179189514726513011, -1.000000000000000000 ) ) ;
#23052=DIRECTION ( 'NONE',  ( 0.000000000000000000, 0.000000000000000000, -1.000000000000000000 ) ) ;
#23066=AXIS2_PLACEMENT_3D ( 'NONE', #20949, #2242, #20800 ) ;
#23068=VECTOR ( 'NONE', #9384, 1000.000000000000000 ) ;
#23075=CARTESIAN_POINT ( 'NONE',  ( 57.00000000000001421, -0.7500000000000000000, -2.421260002560649216 ) ) ;
#23080=CARTESIAN_POINT ( 'NONE',  ( 47.00000000000002132, 2.478823385132571406E-14, 4.100000000000022737 ) ) ;
#23083=CYLINDRICAL_SURFACE ( 'NONE', #28209, 0.05000000000000143219 ) ;
#23084=DIRECTION ( 'NONE',  ( -1.000000000000000000, 0.000000000000000000, 0.000000000000000000 ) ) ;
#23087=CARTESIAN_POINT ( 'NONE',  ( -35.85663232820600399, 5.377732432866631385, -0.5657657256215193886 ) ) ;
#23088=CIRCLE ( 'NONE', #28135, 0.09999999999999982514 ) ;
#23090=CARTESIAN_POINT ( 'NONE',  ( -36.40878371307407235, -2.334862116275012944, 4.877703086529554533 ) ) ;
#23096=AXIS2_PLACEMENT_3D ( 'NONE', #6766, #8810, #26080 ) ;
#23097=AXIS2_PLACEMENT_3D ( 'NONE', #7177, #30764, #25853 ) ;
#23099=CARTESIAN_POINT ( 'NONE',  ( 15.03925126672132961, 3.779372838781728916, 3.883777296072592922 ) ) ;
#23100=( BOUNDED_SURFACE ( )  B_SPLINE_SURFACE ( 3, 2, ( 
 ( #13663, #23345, #31044 ),
 ( #9367, #19034, #7005 ),
 ( #17274, #10292, #26778 ),
 ( #24850, #19665, #22195 ) ),
 .UNSPECIFIED., .F., .F., .F. ) 
 B_SPLINE_SURFACE_WITH_KNOTS ( ( 4, 4 ),
 ( 3, 3 ),
 ( 6.291704175186453303E-05, 0.0002258017310250082428 ),
 ( 0.000000000000000000, 1.000000000000000000 ),
 .UNSPECIFIED. ) 
 GEOMETRIC_REPRESENTATION_ITEM ( )  RATIONAL_B_SPLINE_SURFACE ( (
 ( 1.000000000000000000, 0.8397191227596314533, 1.000000000000000000),
 ( 1.000000000000000000, 0.8408372669632975249, 1.000000000000000000),
 ( 1.000000000000000000, 0.7715695853058209819, 1.000000000000000000),
 ( 1.000000000000000000, 0.7071067811864981678, 1.000000000000000000) ) ) 
 REPRESENTATION_ITEM ( '' )  SURFACE ( )  );
#23103=DIRECTION ( 'NONE',  ( -1.000000000000000000, -1.786976680021873984E-16, -2.459562394685737870E-16 ) ) ;
#23109=CARTESIAN_POINT ( 'NONE',  ( 48.40000000000002700, 0.7707709757764751313, -3.938803467580343831 ) ) ;
#23115=CARTESIAN_POINT ( 'NONE',  ( 57.00059118976931671, 0.7088470050679284151, -2.446935707828179485 ) ) ;
#23125=CARTESIAN_POINT ( 'NONE',  ( 57.00000000000001421, 0.000000000000000000, 0.000000000000000000 ) ) ;
#23128=CARTESIAN_POINT ( 'NONE',  ( -36.22909104983323658, -4.895911367891200960, -2.323639554370684035 ) ) ;
#23133=AXIS2_PLACEMENT_3D ( 'NONE', #4059, #11036, #25283 ) ;
#23134=CARTESIAN_POINT ( 'NONE',  ( 47.06945706549019093, -4.177413309949347564, -1.004109922956873069 ) ) ;
#23136=CARTESIAN_POINT ( 'NONE',  ( -36.25997906085253675, 2.880023619481788533, -4.335093843541867109 ) ) ;
#23137=DIRECTION ( 'NONE',  ( -1.000000000000000000, -0.000000000000000000, -0.000000000000000000 ) ) ;
#23138=FACE_OUTER_BOUND ( 'NONE', #26332, .T. ) ;
#23142=CIRCLE ( 'NONE', #21629, 5.407411300779133789 ) ;
#23144=CARTESIAN_POINT ( 'NONE',  ( -35.98994760229917489, 0.4576450652446111267, -5.200000002521294462 ) ) ;
#23145=VECTOR ( 'NONE', #28709, 1000.000000000000000 ) ;
#23146=EDGE_CURVE ( 'NONE', #9190, #26864, #17650, .T. ) ;
#23152=CYLINDRICAL_SURFACE ( 'NONE', #14329, 0.05000000000000143219 ) ;
#23159=CARTESIAN_POINT ( 'NONE',  ( 15.03925126672132961, 3.056483311920904278, -4.206888370749696904 ) ) ;
#23161=EDGE_CURVE ( 'NONE', #29689, #18491, #13165, .T. ) ;
#23162=VECTOR ( 'NONE', #17365, 1000.000000000000000 ) ;
#23166=CARTESIAN_POINT ( 'NONE',  ( 15.32752150720753370, 2.228039998204479843, -4.927410888447814052 ) ) ;
#23175=EDGE_CURVE ( 'NONE', #17048, #26590, #18105, .T. ) ;
#23176=ORIENTED_EDGE ( 'NONE', *, *, #20952, .F. ) ;
#23178=FACE_OUTER_BOUND ( 'NONE', #31041, .T. ) ;
#23180=DIRECTION ( 'NONE',  ( 0.000000000000000000, 0.000000000000000000, -1.000000000000000000 ) ) ;
#23181=DIRECTION ( 'NONE',  ( 0.000000000000000000, 0.000000000000000000, 1.000000000000000000 ) ) ;
#23185=ADVANCED_FACE ( 'NONE', ( #8423 ), #6064, .T. ) ;
#23187=LINE ( 'NONE', #1949, #26606 ) ;
#23190=CARTESIAN_POINT ( 'NONE',  ( 57.01033040358699111, 0.8080171122822069618, 2.471263581425196421 ) ) ;
#23191=CARTESIAN_POINT ( 'NONE',  ( 51.80000000000002558, -4.179189514726507682, 0.9999999999999997780 ) ) ;
#23201=ORIENTED_EDGE ( 'NONE', *, *, #20324, .F. ) ;
#23205=CARTESIAN_POINT ( 'NONE',  ( 48.50000000000002132, -1.391941090707485396, 3.850000000000022737 ) ) ;
#23206=ORIENTED_EDGE ( 'NONE', *, *, #12313, .F. ) ;
#23210=LINE ( 'NONE', #18770, #14673 ) ;
#23224=AXIS2_PLACEMENT_3D ( 'NONE', #26555, #5026, #24032 ) ;
#23226=ORIENTED_EDGE ( 'NONE', *, *, #4707, .F. ) ;
#23236=CARTESIAN_POINT ( 'NONE',  ( -36.39645873810206211, 3.590618801409514838, 4.051716037497281597 ) ) ;
#23238=ORIENTED_EDGE ( 'NONE', *, *, #27242, .T. ) ;
#23242=DIRECTION ( 'NONE',  ( 0.000000000000000000, 0.000000000000000000, -1.000000000000000000 ) ) ;
#23244=CARTESIAN_POINT ( 'NONE',  ( 47.00000000000002132, -1.391941090707485396, 3.750000000000022649 ) ) ;
#23246=CARTESIAN_POINT ( 'NONE',  ( -36.48174642953002689, 5.008501212420958026, -2.048848402342137387 ) ) ;
#23247=ADVANCED_FACE ( 'NONE', ( #21858 ), #2193, .T. ) ;
#23255=AXIS2_PLACEMENT_3D ( 'NONE', #26955, #24582, #8268 ) ;
#23259=CARTESIAN_POINT ( 'NONE',  ( -35.85663232820584057, 0.4576450603546987628, 5.200000000000000178 ) ) ;
#23260=CARTESIAN_POINT ( 'NONE',  ( 44.98443556292537693, -3.726179070414207928, 1.100000000000000311 ) ) ;
#23265=CIRCLE ( 'NONE', #5041, 2.600000000000000089 ) ;
#23272=VERTEX_POINT ( 'NONE', #19633 ) ;
#23273=FACE_BOUND ( 'NONE', #10355, .T. ) ;
#23280=CARTESIAN_POINT ( 'NONE',  ( -36.92405921417685022, 3.294441450831133711, 4.290383166762168798 ) ) ;
#23285=DIRECTION ( 'NONE',  ( 1.000000000000000000, 0.000000000000000000, 0.000000000000000000 ) ) ;
#23292=AXIS2_PLACEMENT_3D ( 'NONE', #4806, #21460, #9418 ) ;
#23293=CARTESIAN_POINT ( 'NONE',  ( 15.03925126672132961, -1.123735532908297863, -5.289358697221544503 ) ) ;
#23299=CARTESIAN_POINT ( 'NONE',  ( -35.85663232820584057, -5.086913985776155833, -1.171642053949114803 ) ) ;
#23300=ORIENTED_EDGE ( 'NONE', *, *, #8623, .F. ) ;
#23306=VERTEX_POINT ( 'NONE', #9958 ) ;
#23311=ORIENTED_EDGE ( 'NONE', *, *, #12019, .F. ) ;
#23315=CARTESIAN_POINT ( 'NONE',  ( 15.03925126672132961, 0.4576450603546987628, 5.200000000000000178 ) ) ;
#23319=VERTEX_POINT ( 'NONE', #16930 ) ;
#23337=ORIENTED_EDGE ( 'NONE', *, *, #14704, .F. ) ;
#23339=LINE ( 'NONE', #17962, #8026 ) ;
#23345=CARTESIAN_POINT ( 'NONE',  ( 57.05000000000001137, -0.7500000000000000000, -1.746008434843730583 ) ) ;
#23361=VERTEX_POINT ( 'NONE', #11498 ) ;
#23367=EDGE_CURVE ( 'NONE', #29967, #30656, #24901, .T. ) ;
#23368=CARTESIAN_POINT ( 'NONE',  ( 15.03925126672132961, -0.9159215771349724644, -4.311190327366005270 ) ) ;
#23370=CARTESIAN_POINT ( 'NONE',  ( -36.50489844130401451, -2.884962146574324926, 4.577321775072974219 ) ) ;
#23374=DIRECTION ( 'NONE',  ( -1.000000000000000000, -0.000000000000000000, -0.000000000000000000 ) ) ;
#23377=EDGE_CURVE ( 'NONE', #15671, #2569, #6589, .T. ) ;
#23379=CARTESIAN_POINT ( 'NONE',  ( -43.84599839145305111, -8.171597657156649598E-15, 0.000000000000000000 ) ) ;
#23385=CARTESIAN_POINT ( 'NONE',  ( -36.89017861347080185, 3.436881753486414670, 4.177093996075273097 ) ) ;
#23392=DIRECTION ( 'NONE',  ( 0.000000000000000000, 0.000000000000000000, 1.000000000000000000 ) ) ;
#23395=ADVANCED_FACE ( 'NONE', ( #1823 ), #21177, .T. ) ;
#23397=CARTESIAN_POINT ( 'NONE',  ( -36.80043232705879319, 4.951626736499065373, -2.174059107776711297 ) ) ;
#23398=EDGE_CURVE ( 'NONE', #16762, #24288, #7702, .T. ) ;
#23401=CARTESIAN_POINT ( 'NONE',  ( 57.00000000000001421, 0.6820512820512794061, 1.773360101234991326 ) ) ;
#23404=DIRECTION ( 'NONE',  ( 0.000000000000000000, 2.818925648462304271E-14, 1.000000000000000000 ) ) ;
#23408=ORIENTED_EDGE ( 'NONE', *, *, #3991, .F. ) ;
#23409=DIRECTION ( 'NONE',  ( -1.000000000000000000, 0.000000000000000000, 0.000000000000000000 ) ) ;
#23415=ORIENTED_EDGE ( 'NONE', *, *, #5495, .F. ) ;
#23418=ADVANCED_FACE ( 'NONE', ( #31112 ), #11246, .T. ) ;
#23425=FACE_OUTER_BOUND ( 'NONE', #7791, .T. ) ;
#23430=DIRECTION ( 'NONE',  ( 1.000000000000000000, -7.137062321648221502E-17, -7.924918191827128155E-17 ) ) ;
#23432=DIRECTION ( 'NONE',  ( 0.000000000000000000, -1.224646799147362821E-16, 1.000000000000000000 ) ) ;
#23437=CARTESIAN_POINT ( 'NONE',  ( -36.48821680285229974, 3.495540671458303716, -4.131527132740814956 ) ) ;
#23440=CARTESIAN_POINT ( 'NONE',  ( 16.10667815269232506, 0.1434351685890397909, -5.407416993630365987 ) ) ;
#23441=SPHERICAL_SURFACE ( 'NONE', #16963, 0.05000000000000000278 ) ;
#23451=DIRECTION ( 'NONE',  ( -1.000000000000000000, 0.000000000000000000, 0.000000000000000000 ) ) ;
#23453=EDGE_LOOP ( 'NONE', ( #6966, #19248, #18134, #7007 ) ) ;
#23454=CARTESIAN_POINT ( 'NONE',  ( 48.33022520384532328, 1.142230555601122965, 3.938343097974785767 ) ) ;
#23459=DIRECTION ( 'NONE',  ( -1.000000000000000000, 0.000000000000000000, 0.000000000000000000 ) ) ;
#23462=ADVANCED_FACE ( 'NONE', ( #20421 ), #30045, .T. ) ;
#23469=DIRECTION ( 'NONE',  ( 0.000000000000000000, 0.000000000000000000, 1.000000000000000000 ) ) ;
#23470=DIRECTION ( 'NONE',  ( 1.000000000000000000, -0.000000000000000000, 0.000000000000000000 ) ) ;
#23476=CIRCLE ( 'NONE', #4259, 2.549999999999999822 ) ;
#23478=CARTESIAN_POINT ( 'NONE',  ( 15.98305126557416500, 5.283830060792412020, -1.151642405604206720 ) ) ;
#23482=CARTESIAN_POINT ( 'NONE',  ( 50.30000000000001847, 1.391941090707534023, -3.850000000000022737 ) ) ;
#23490=DIRECTION ( 'NONE',  ( 0.000000000000000000, 0.000000000000000000, -1.000000000000000000 ) ) ;
#23499=EDGE_LOOP ( 'NONE', ( #12803, #23525, #14758, #21779 ) ) ;
#23503=LINE ( 'NONE', #11476, #9117 ) ;
#23504=EDGE_LOOP ( 'NONE', ( #21344, #30461 ) ) ;
#23507=CARTESIAN_POINT ( 'NONE',  ( 50.30000000000001847, -1.426739617975173013, -3.843750000000023093 ) ) ;
#23513=DIRECTION ( 'NONE',  ( 0.000000000000000000, 0.000000000000000000, -1.000000000000000000 ) ) ;
#23522=DIRECTION ( 'NONE',  ( 0.000000000000000000, 0.000000000000000000, -1.000000000000000000 ) ) ;
#23525=ORIENTED_EDGE ( 'NONE', *, *, #3407, .F. ) ;
#23536=CARTESIAN_POINT ( 'NONE',  ( -36.27260443516980359, 3.212533369474494638, 4.093511368021819585 ) ) ;
#23538=DIRECTION ( 'NONE',  ( 1.000000000000000000, -0.000000000000000000, -0.000000000000000000 ) ) ;
#23539=ORIENTED_EDGE ( 'NONE', *, *, #11641, .T. ) ;
#23540=CIRCLE ( 'NONE', #26584, 4.100000000000022737 ) ;
#23545=DIRECTION ( 'NONE',  ( 1.000000000000000000, 3.385297212316258532E-16, -2.459562394685744279E-16 ) ) ;
#23552=CARTESIAN_POINT ( 'NONE',  ( 57.05000000000001847, 0.7500000000000000000, 1.778341924377873751 ) ) ;
#23554=AXIS2_PLACEMENT_3D ( 'NONE', #22784, #1073, #7721 ) ;
#23556=CARTESIAN_POINT ( 'NONE',  ( 51.86040321072245263, 0.1224230307917539146, 4.365444804395989919 ) ) ;
#23557=CIRCLE ( 'NONE', #291, 4.275000000000000355 ) ;
#23559=CARTESIAN_POINT ( 'NONE',  ( 33.47623932017462778, 4.375000000000001776, 5.948056943527305374E-16 ) ) ;
#23570=DIRECTION ( 'NONE',  ( 0.000000000000000000, 5.942513678379226626E-16, 1.000000000000000000 ) ) ;
#23571=CARTESIAN_POINT ( 'NONE',  ( -36.92362342067168868, 0.1627367787822124878, 5.407318510437578496 ) ) ;
#23575=CARTESIAN_POINT ( 'NONE',  ( 47.00000000000002132, 2.428612866367529932E-14, -4.100000000000022737 ) ) ;
#23583=DIRECTION ( 'NONE',  ( 0.000000000000000000, 0.000000000000000000, -1.000000000000000000 ) ) ;
#23584=AXIS2_PLACEMENT_3D ( 'NONE', #11916, #9074, #11275 ) ;
#23587=ORIENTED_EDGE ( 'NONE', *, *, #19270, .T. ) ;
#23591=AXIS2_PLACEMENT_3D ( 'NONE', #2167, #28782, #7239 ) ;
#23592=TOROIDAL_SURFACE ( 'NONE', #30148, -24.59258869922086888, 30.00000000000000000 ) ;
#23595=DIRECTION ( 'NONE',  ( -1.000000000000000000, 0.000000000000000000, -0.000000000000000000 ) ) ;
#23596=AXIS2_PLACEMENT_3D ( 'NONE', #364, #19698, #7957 ) ;
#23599=ORIENTED_EDGE ( 'NONE', *, *, #6615, .F. ) ;
#23601=EDGE_CURVE ( 'NONE', #10142, #618, #26981, .T. ) ;
#23602=AXIS2_PLACEMENT_3D ( 'NONE', #27758, #10970, #1462 ) ;
#23603=CARTESIAN_POINT ( 'NONE',  ( -36.11692583559977976, 2.199885872770852124, -4.939696258129341544 ) ) ;
#23607=AXIS2_PLACEMENT_3D ( 'NONE', #17888, #5847, #622 ) ;
#23608=CARTESIAN_POINT ( 'NONE',  ( 57.00000000000001421, -0.6999999999999999556, -2.452039967047845437 ) ) ;
#23610=LINE ( 'NONE', #16468, #17470 ) ;
#23616=CARTESIAN_POINT ( 'NONE',  ( 50.30000000000001847, -1.391941090707485396, -3.850000000000022737 ) ) ;
#23622=FACE_OUTER_BOUND ( 'NONE', #24081, .T. ) ;
#23623=CARTESIAN_POINT ( 'NONE',  ( 15.61552784268231520, -4.977698683490599407, 2.127480166903654268 ) ) ;
#23624=ORIENTED_EDGE ( 'NONE', *, *, #19892, .T. ) ;
#23625=VERTEX_POINT ( 'NONE', #11586 ) ;
#23626=CARTESIAN_POINT ( 'NONE',  ( -36.30347965937279753, -4.910307320510546525, 1.715181477143133071 ) ) ;
#23629=CARTESIAN_POINT ( 'NONE',  ( 36.50000000000002132, -0.8000000000000000444, -1.778341924377873751 ) ) ;
#23633=ORIENTED_EDGE ( 'NONE', *, *, #26592, .T. ) ;
#23639=ADVANCED_FACE ( 'NONE', ( #21266 ), #9641, .T. ) ;
#23640=VERTEX_POINT ( 'NONE', #17372 ) ;
#23647=CARTESIAN_POINT ( 'NONE',  ( 57.00791613703923844, -0.8068646677135199452, 2.471635681327667644 ) ) ;
#23649=CARTESIAN_POINT ( 'NONE',  ( -35.85663232820584767, 4.683225679163358635, -2.703237727951174563 ) ) ;
#23652=CARTESIAN_POINT ( 'NONE',  ( -35.85663232820584057, 2.686240680702182804, -4.475885388010699018 ) ) ;
#23653=CARTESIAN_POINT ( 'NONE',  ( 57.05000000000001847, -0.8000000000000001554, -1.778341924377873973 ) ) ;
#23654=AXIS2_PLACEMENT_3D ( 'NONE', #20405, #11043, #926 ) ;
#23655=CIRCLE ( 'NONE', #5960, 4.275000000000000355 ) ;
#23658=CARTESIAN_POINT ( 'NONE',  ( 15.29384114148388818, 5.068511731019603062, -1.228278365481837220 ) ) ;
#23662=CARTESIAN_POINT ( 'NONE',  ( 57.02184386277451722, 0.7500000000000000000, -2.421260326253384942 ) ) ;
#23664=VERTEX_POINT ( 'NONE', #12615 ) ;
#23667=CARTESIAN_POINT ( 'NONE',  ( 15.03925126672132961, -4.018128179617538542, -3.618665901676658248 ) ) ;
#23674=CARTESIAN_POINT ( 'NONE',  ( 15.76675455518196678, 5.174628573245020569, 1.572974725650792438 ) ) ;
#23677=DIRECTION ( 'NONE',  ( -1.000000000000000000, 0.000000000000000000, 0.000000000000000000 ) ) ;
#23678=EDGE_LOOP ( 'NONE', ( #14460, #9266, #1878, #22190 ) ) ;
#23685=CIRCLE ( 'NONE', #10019, 0.05000000000000143219 ) ;
#23686=EDGE_CURVE ( 'NONE', #20639, #24678, #649, .T. ) ;
#23688=DIRECTION ( 'NONE',  ( 0.000000000000000000, -1.000000000000000000, 0.000000000000000000 ) ) ;
#23691=EDGE_LOOP ( 'NONE', ( #9721, #14723, #2066 ) ) ;
#23692=DIRECTION ( 'NONE',  ( 0.000000000000000000, 1.000000000000000000, 0.000000000000000000 ) ) ;
#23693=CARTESIAN_POINT ( 'NONE',  ( 56.96274124341056222, 0.7308628367038140228, 1.753832840855930719 ) ) ;
#23697=PLANE ( 'NONE',  #30614 ) ;
#23698=CARTESIAN_POINT ( 'NONE',  ( 46.99309270008836847, -4.271967808728817317, 0.9446991603439680585 ) ) ;
#23703=AXIS2_PLACEMENT_3D ( 'NONE', #6213, #3538, #839 ) ;
#23709=CARTESIAN_POINT ( 'NONE',  ( -36.42771574642738130, 3.560621078037010001, 4.077054076718899189 ) ) ;
#23714=DIRECTION ( 'NONE',  ( 1.000000000000000000, 2.586136946169074517E-16, -0.000000000000000000 ) ) ;
#23716=CARTESIAN_POINT ( 'NONE',  ( 50.40918227724429812, 1.198378070452317257, 3.921585382224057614 ) ) ;
#23717=DIRECTION ( 'NONE',  ( 0.000000000000000000, 1.000000000000000000, 0.000000000000000000 ) ) ;
#23719=CARTESIAN_POINT ( 'NONE',  ( 56.99137905793185155, -0.7079296279778910517, 1.763407125847052725 ) ) ;
#23721=EDGE_CURVE ( 'NONE', #8161, #19150, #8732, .T. ) ;
#23723=PLANE ( 'NONE',  #16277 ) ;
#23728=CARTESIAN_POINT ( 'NONE',  ( 50.50000000000001421, 0.6462379109120998111, -4.048750000000022276 ) ) ;
#23735=CARTESIAN_POINT ( 'NONE',  ( -36.23324115033522475, -0.2667568399897324860, 5.200000000294890512 ) ) ;
#23738=CARTESIAN_POINT ( 'NONE',  ( -36.89831264271880684, -5.047763082740456930, 1.943828653492516212 ) ) ;
#23744=FACE_BOUND ( 'NONE', #14850, .T. ) ;
#23745=( GEOMETRIC_REPRESENTATION_CONTEXT ( 3 ) GLOBAL_UNCERTAINTY_ASSIGNED_CONTEXT ( ( #5371 ) ) GLOBAL_UNIT_ASSIGNED_CONTEXT ( ( #4761, #19505, #7305 ) ) REPRESENTATION_CONTEXT ( 'NONE', 'WORKASPACE' ) );
#23755=EDGE_CURVE ( 'NONE', #2624, #3490, #19371, .T. ) ;
#23756=DIRECTION ( 'NONE',  ( 0.000000000000000000, 0.000000000000000000, 1.000000000000000000 ) ) ;
#23759=CARTESIAN_POINT ( 'NONE',  ( -54.45487361440510909, 1.499999999999999556, -4.029888335921975262 ) ) ;
#23761=ORIENTED_EDGE ( 'NONE', *, *, #22889, .T. ) ;
#23763=AXIS2_PLACEMENT_3D ( 'NONE', #26103, #23583, #18682 ) ;
#23770=CARTESIAN_POINT ( 'NONE',  ( 58.45000000000001705, -0.8000000000000000444, 1.778341924377873751 ) ) ;
#23771=CARTESIAN_POINT ( 'NONE',  ( 50.50000000000002132, 2.428612866367529932E-14, 0.000000000000000000 ) ) ;
#23773=CARTESIAN_POINT ( 'NONE',  ( -35.85663232820584057, 3.275050215668543263, 2.949461045527633996 ) ) ;
#23778=CARTESIAN_POINT ( 'NONE',  ( 15.41080140630260686, -2.595266697484886365, -4.757426534476337565 ) ) ;
#23779=CARTESIAN_POINT ( 'NONE',  ( 15.76675455518197388, -5.110933801299744950, 1.769007076671009093 ) ) ;
#23783=CARTESIAN_POINT ( 'NONE',  ( -35.85663232820578372, -4.683225679163362187, 2.703237727951222968 ) ) ;
#23789=ORIENTED_EDGE ( 'NONE', *, *, #27536, .F. ) ;
#23798=CARTESIAN_POINT ( 'NONE',  ( 56.95640338720422591, -0.7513613876702617267, 2.489093304807997509 ) ) ;
#23802=CARTESIAN_POINT ( 'NONE',  ( -35.85663232820584767, 4.683225679163358635, -2.703237727951174563 ) ) ;
#23805=DIRECTION ( 'NONE',  ( -1.000000000000000000, -0.000000000000000000, -0.000000000000000000 ) ) ;
#23807=CARTESIAN_POINT ( 'NONE',  ( 15.57907767661756182, 5.286410563980352251, -1.167394352644079314 ) ) ;
#23811=ORIENTED_EDGE ( 'NONE', *, *, #10338, .F. ) ;
#23813=CARTESIAN_POINT ( 'NONE',  ( 50.42118334212123898, -1.311095223031168766, 3.884869838566831657 ) ) ;
#23820=EDGE_CURVE ( 'NONE', #31094, #7978, #16218, .T. ) ;
#23821=FACE_OUTER_BOUND ( 'NONE', #28479, .T. ) ;
#23825=ORIENTED_EDGE ( 'NONE', *, *, #22966, .T. ) ;
#23826=CARTESIAN_POINT ( 'NONE',  ( 15.76623786017564122, 5.109611055794853307, 1.772889539330601449 ) ) ;
#23836=EDGE_CURVE ( 'NONE', #9397, #8955, #13763, .T. ) ;
#23837=LINE ( 'NONE', #23984, #24863 ) ;
#23846=CARTESIAN_POINT ( 'NONE',  ( 51.72668767004672929, -4.179189507150981697, 0.9999999999999995559 ) ) ;
#23847=CARTESIAN_POINT ( 'NONE',  ( 15.03925126672132784, 5.086913985776138070, 1.171642053949162987 ) ) ;
#23852=AXIS2_PLACEMENT_3D ( 'NONE', #18159, #1185, #3876 ) ;
#23855=DIRECTION ( 'NONE',  ( 1.520093157366863638E-16, -0.5877852522924685852, -0.8090169943749507819 ) ) ;
#23858=CARTESIAN_POINT ( 'NONE',  ( -36.31440869660544024, 3.012234853004066348, 4.239036759381678898 ) ) ;
#23862=EDGE_LOOP ( 'NONE', ( #7159, #27866, #19202, #3173 ) ) ;
#23865=CARTESIAN_POINT ( 'NONE',  ( -35.85663232820584767, 5.377732432866621615, 0.5657657256216177544 ) ) ;
#23866=DIRECTION ( 'NONE',  ( 1.000000000000000000, 3.385297212316223527E-16, 2.459562394685754633E-16 ) ) ;
#23869=CARTESIAN_POINT ( 'NONE',  ( 57.01262970566578758, 0.7335977677777304473, 1.792760110902297921 ) ) ;
#23871=CARTESIAN_POINT ( 'NONE',  ( -36.40793637698146057, 0.9785522574021833231, -5.318456145981288685 ) ) ;
#23873=DIRECTION ( 'NONE',  ( 0.000000000000000000, -0.000000000000000000, -1.000000000000000000 ) ) ;
#23875=CARTESIAN_POINT ( 'NONE',  ( -44.49999999999999289, 1.499999999999999556, 3.300094695611021756 ) ) ;
#23876=CIRCLE ( 'NONE', #601, 0.09999999999999982514 ) ;
#23877=AXIS2_PLACEMENT_3D ( 'NONE', #19092, #9105, #26504 ) ;
#23879=DIRECTION ( 'NONE',  ( 0.000000000000000000, 0.000000000000000000, -1.000000000000000000 ) ) ;
#23882=EDGE_LOOP ( 'NONE', ( #22110, #4830, #18408, #21418 ) ) ;
#23884=CARTESIAN_POINT ( 'NONE',  ( -36.31414349454749413, 0.05686983728433445129, 5.199999998842928406 ) ) ;
#23888=CARTESIAN_POINT ( 'NONE',  ( -54.49853245345825314, 1.536420219664552445, 4.055116445457032981 ) ) ;
#23892=DIRECTION ( 'NONE',  ( 0.000000000000000000, 0.000000000000000000, -1.000000000000000000 ) ) ;
#23894=CARTESIAN_POINT ( 'NONE',  ( -43.84599839145305111, -8.171597657156649598E-15, 0.000000000000000000 ) ) ;
#23910=CARTESIAN_POINT ( 'NONE',  ( 15.29954477411492242, -4.018128194441231926, 3.618665885216586720 ) ) ;
#23914=CARTESIAN_POINT ( 'NONE',  ( 57.00000000000001421, 0.000000000000000000, 0.000000000000000000 ) ) ;
#23925=CARTESIAN_POINT ( 'NONE',  ( 50.40000000000001990, 2.428612866367529932E-14, 0.000000000000000000 ) ) ;
#23927=CARTESIAN_POINT ( 'NONE',  ( 15.76623786017565187, -3.091683853621961298, -4.437651790014649045 ) ) ;
#23928=CARTESIAN_POINT ( 'NONE',  ( -36.23324115033478421, 4.863061488092484730, 1.860589201779825341 ) ) ;
#23929=CARTESIAN_POINT ( 'NONE',  ( 15.22842924604202786, -4.861582136950232780, 2.394243986684292391 ) ) ;
#23934=CARTESIAN_POINT ( 'NONE',  ( 56.98113911906671092, 0.7884861235339004626, -2.477567088838556586 ) ) ;
#23936=EDGE_LOOP ( 'NONE', ( #5446, #17453, #29289, #31186 ) ) ;
#23938=VERTEX_POINT ( 'NONE', #2265 ) ;
#23939=SHAPE_REPRESENTATION_RELATIONSHIP ( 'NONE' , 'NONE' ,  #18201, #12719 ) ;
#23957=CARTESIAN_POINT ( 'NONE',  ( -36.00197790576392975, -2.199885893005944837, -4.939696249117692339 ) ) ;
#23958=ORIENTED_EDGE ( 'NONE', *, *, #10719, .F. ) ;
#23961=EDGE_CURVE ( 'NONE', #2253, #19424, #26935, .T. ) ;
#23962=CARTESIAN_POINT ( 'NONE',  ( 50.30837315852409830, 1.391941090707552897, -3.850000000000020517 ) ) ;
#23963=CARTESIAN_POINT ( 'NONE',  ( 48.38952526309123670, -0.7808213810455604253, 4.027268569370238360 ) ) ;
#23969=DIRECTION ( 'NONE',  ( 1.000000000000000000, -0.000000000000000000, -0.000000000000000000 ) ) ;
#23975=CARTESIAN_POINT ( 'NONE',  ( 15.57907767661755649, 4.962973169597125533, 2.162832296644338737 ) ) ;
#23976=ORIENTED_EDGE ( 'NONE', *, *, #533, .F. ) ;
#23984=CARTESIAN_POINT ( 'NONE',  ( -35.85663232820584057, -0.4576450603546987628, 5.200000000000000178 ) ) ;
#23988=DIRECTION ( 'NONE',  ( 1.000000000000000000, 0.000000000000000000, -0.000000000000000000 ) ) ;
#23990=CARTESIAN_POINT ( 'NONE',  ( 56.99150396717417522, 0.7610778266783598811, 1.740907964752457904 ) ) ;
#23991=ADVANCED_FACE ( 'NONE', ( #10646 ), #30572, .T. ) ;
#23993=CARTESIAN_POINT ( 'NONE',  ( -36.11692583559974423, -2.199885872771085271, 4.939696258129251838 ) ) ;
#23994=CARTESIAN_POINT ( 'NONE',  ( 57.05000000000001847, 0.7500000000000000000, 2.421260002560649660 ) ) ;
#24008=VERTEX_POINT ( 'NONE', #12543 ) ;
#24015=CARTESIAN_POINT ( 'NONE',  ( 34.50000000000001421, 0.000000000000000000, -3.200000000000000178 ) ) ;
#24016=CARTESIAN_POINT ( 'NONE',  ( 57.04540039768303217, 0.7500000000000000000, 1.778341924377873751 ) ) ;
#24017=DIRECTION ( 'NONE',  ( 0.000000000000000000, -0.2573099415204678775, -0.9663289263986324373 ) ) ;
#24018=CARTESIAN_POINT ( 'NONE',  ( 58.45000000000001705, -0.8000000000000000444, -2.421260002560649660 ) ) ;
#24019=AXIS2_PLACEMENT_3D ( 'NONE', #13304, #8572, #8263 ) ;
#24023=EDGE_CURVE ( 'NONE', #1800, #1101, #21504, .T. ) ;
#24024=DIRECTION ( 'NONE',  ( 3.167104333282667910E-32, -1.224646799147353207E-16, 1.000000000000000000 ) ) ;
#24025=DIRECTION ( 'NONE',  ( 0.000000000000000000, 0.000000000000000000, -1.000000000000000000 ) ) ;
#24027=ORIENTED_EDGE ( 'NONE', *, *, #943, .F. ) ;
#24032=DIRECTION ( 'NONE',  ( 0.000000000000000000, 0.000000000000000000, -1.000000000000000000 ) ) ;
#24035=EDGE_CURVE ( 'NONE', #12135, #25275, #22136, .T. ) ;
#24037=AXIS2_PLACEMENT_3D ( 'NONE', #7760, #17425, #27071 ) ;
#24038=CARTESIAN_POINT ( 'NONE',  ( 15.29384114148384199, 0.3980941177579093715, -5.199999998461561468 ) ) ;
#24042=DIRECTION ( 'NONE',  ( 1.000000000000000000, 2.586136946169074517E-16, -0.000000000000000000 ) ) ;
#24044=FACE_OUTER_BOUND ( 'NONE', #20252, .T. ) ;
#24045=CARTESIAN_POINT ( 'NONE',  ( 34.55000000000001847, 0.000000000000000000, 0.000000000000000000 ) ) ;
#24046=ORIENTED_EDGE ( 'NONE', *, *, #29244, .F. ) ;
#24050=VECTOR ( 'NONE', #10158, 1000.000000000000000 ) ;
#24052=VECTOR ( 'NONE', #16843, 1000.000000000000000 ) ;
#24053=CARTESIAN_POINT ( 'NONE',  ( 57.00000000000001421, 0.000000000000000000, 0.000000000000000000 ) ) ;
#24055=DIRECTION ( 'NONE',  ( 1.000000000000000000, -0.000000000000000000, -0.000000000000000000 ) ) ;
#24057=ORIENTED_EDGE ( 'NONE', *, *, #13, .T. ) ;
#24062=CARTESIAN_POINT ( 'NONE',  ( 15.76623786017565187, -3.265074799938555206, 4.311675893544620664 ) ) ;
#24066=CARTESIAN_POINT ( 'NONE',  ( 33.47623932017462778, 5.377732432866640266, 0.5657657256216092057 ) ) ;
#24067=CARTESIAN_POINT ( 'NONE',  ( 33.47623932017462778, 4.018128179617571405, -3.618665901676623164 ) ) ;
#24070=CARTESIAN_POINT ( 'NONE',  ( 50.40000000000001990, -0.6304760106459033064, -3.950000000000022826 ) ) ;
#24074=LINE ( 'NONE', #14722, #15340 ) ;
#24077=CARTESIAN_POINT ( 'NONE',  ( 15.39414421509785491, -2.821511581828335391, -4.377605326016334786 ) ) ;
#24078=CARTESIAN_POINT ( 'NONE',  ( -36.11187263677958725, 4.822464347459026968, 1.985534350301239481 ) ) ;
#24079=CYLINDRICAL_SURFACE ( 'NONE', #13526, 0.05000000000000012768 ) ;
#24080=CIRCLE ( 'NONE', #3327, 4.100000000000022737 ) ;
#24081=EDGE_LOOP ( 'NONE', ( #13742, #17858, #12175, #8957 ) ) ;
#24091=CARTESIAN_POINT ( 'NONE',  ( -36.48821680285229263, -5.009497273852872468, -2.047744636826959397 ) ) ;
#24094=VECTOR ( 'NONE', #28148, 1000.000000000000000 ) ;
#24097=AXIS2_PLACEMENT_3D ( 'NONE', #16249, #21001, #15774 ) ;
#24103=CARTESIAN_POINT ( 'NONE',  ( 47.10000000000002274, -4.179189514726507682, 0.9999999999999997780 ) ) ;
#24104=CYLINDRICAL_SURFACE ( 'NONE', #28107, 0.05000000000000143219 ) ;
#24110=CARTESIAN_POINT ( 'NONE',  ( -35.85663232820584057, 4.804073783693455724, -2.042134687550314354 ) ) ;
#24111=CARTESIAN_POINT ( 'NONE',  ( -36.31414349454749413, -0.05686983728438164964, -5.199999998842928406 ) ) ;
#24112=( BOUNDED_SURFACE ( )  B_SPLINE_SURFACE ( 3, 2, ( 
 ( #4550, #22423, #13065 ),
 ( #5305, #567, #17835 ),
 ( #15286, #20224, #24933 ),
 ( #14811, #10078, #19602 ),
 ( #15133, #26998, #420 ),
 ( #7837, #19753, #715 ),
 ( #12747, #3254, #29383 ),
 ( #5635, #3097, #17680 ),
 ( #5787, #20058, #7553 ),
 ( #29852, #8166, #29523 ),
 ( #257, #15442, #27469 ),
 ( #17514, #10375, #2950 ),
 ( #24472, #27169, #12595 ),
 ( #25094, #5481, #29695 ),
 ( #7695, #17353, #8015 ),
 ( #12897, #10225, #890 ) ),
 .UNSPECIFIED., .F., .F., .F. ) 
 B_SPLINE_SURFACE_WITH_KNOTS ( ( 4, 2, 2, 2, 2, 2, 2, 4 ),
 ( 3, 3 ),
 ( 0.001780502285214213788, 0.002558945925323803227, 0.002753556835351200424, 0.002948167745378598055, 0.003337389565433392449, 0.003726611385488186844, 0.004115833205542981238, 0.004894276845652570894 ),
 ( 0.000000000000000000, 1.000000000000000000 ),
 .UNSPECIFIED. ) 
 GEOMETRIC_REPRESENTATION_ITEM ( )  RATIONAL_B_SPLINE_SURFACE ( (
 ( 1.000000000000000000, 0.9418517008537217183, 1.000000000000000000),
 ( 1.000000000000000000, 0.9417987965884941914, 1.000000000000000000),
 ( 1.000000000000000000, 0.9418198861734206062, 1.000000000000000000),
 ( 1.000000000000000000, 0.9434060303845515083, 1.000000000000000000),
 ( 1.000000000000000000, 0.9437939819948067965, 1.000000000000000000),
 ( 1.000000000000000000, 0.9445989566712852392, 1.000000000000000000),
 ( 1.000000000000000000, 0.9450169930049960865, 1.000000000000000000),
 ( 1.000000000000000000, 0.9461610507673310355, 1.000000000000000000),
 ( 1.000000000000000000, 0.9467217966427192710, 1.000000000000000000),
 ( 1.000000000000000000, 0.9467345476124342518, 1.000000000000000000),
 ( 1.000000000000000000, 0.9461964028052916031, 1.000000000000000000),
 ( 1.000000000000000000, 0.9446801822473820387, 1.000000000000000000),
 ( 1.000000000000000000, 0.9437582546536950057, 1.000000000000000000),
 ( 1.000000000000000000, 0.9418129560294778990, 1.000000000000000000),
 ( 1.000000000000000000, 0.9418016889778114686, 1.000000000000000000),
 ( 1.000000000000000000, 0.9418517008537208302, 1.000000000000000000) ) ) 
 REPRESENTATION_ITEM ( '' )  SURFACE ( )  );
#24114=CARTESIAN_POINT ( 'NONE',  ( 15.87128154250932255, 4.872353571451126797, -2.347449169364848487 ) ) ;
#24117=ORIENTED_EDGE ( 'NONE', *, *, #29245, .F. ) ;
#24118=EDGE_CURVE ( 'NONE', #13582, #30927, #7817, .T. ) ;
#24121=VECTOR ( 'NONE', #11376, 1000.000000000000000 ) ;
#24144=ORIENTED_EDGE ( 'NONE', *, *, #19031, .F. ) ;
#24147=ADVANCED_FACE ( 'NONE', ( #20476 ), #15908, .T. ) ;
#24149=CARTESIAN_POINT ( 'NONE',  ( 57.00000000000001421, 0.000000000000000000, 0.000000000000000000 ) ) ;
#24152=EDGE_CURVE ( 'NONE', #15593, #6507, #14047, .T. ) ;
#24158=CARTESIAN_POINT ( 'NONE',  ( 51.75337531998826535, -4.276948325786879224, 0.9210526687159865666 ) ) ;
#24166=CARTESIAN_POINT ( 'NONE',  ( 51.88778388204188730, 0.01071552754804109761, -4.374297461196706927 ) ) ;
#24171=CIRCLE ( 'NONE', #1844, 1.899999999999999911 ) ;
#24176=ORIENTED_EDGE ( 'NONE', *, *, #8441, .T. ) ;
#24180=CARTESIAN_POINT ( 'NONE',  ( 50.42106458229518751, 0.9199776782966334610, 3.998258245321812510 ) ) ;
#24190=DIRECTION ( 'NONE',  ( -1.000000000000000000, -0.000000000000000000, -0.000000000000000000 ) ) ;
#24191=CARTESIAN_POINT ( 'NONE',  ( 51.90000000000001279, -4.227689052994015206, -1.125730994152046804 ) ) ;
#24193=CARTESIAN_POINT ( 'NONE',  ( 15.18459684427940104, -5.377732432866643819, -0.5657657256215741226 ) ) ;
#24194=ORIENTED_EDGE ( 'NONE', *, *, #27077, .T. ) ;
#24195=CARTESIAN_POINT ( 'NONE',  ( -36.79682133506354091, 0.5584590966806799450, 5.380195666604549842 ) ) ;
#24204=CARTESIAN_POINT ( 'NONE',  ( 15.67083574136730384, -0.3995010896671927214, -5.397102918580121589 ) ) ;
#24212=CARTESIAN_POINT ( 'NONE',  ( -54.49983703358571319, -1.542636180423123449, -4.059406436927352146 ) ) ;
#24213=EDGE_CURVE ( 'NONE', #29437, #30188, #22500, .T. ) ;
#24223=DIRECTION ( 'NONE',  ( 0.000000000000000000, 0.000000000000000000, -1.000000000000000000 ) ) ;
#24241=FACE_OUTER_BOUND ( 'NONE', #25941, .T. ) ;
#24253=ORIENTED_EDGE ( 'NONE', *, *, #25455, .F. ) ;
#24254=CIRCLE ( 'NONE', #13110, 2.600000000000000089 ) ;
#24257=EDGE_LOOP ( 'NONE', ( #4370, #19065, #19340, #18552, #9661 ) ) ;
#24259=CIRCLE ( 'NONE', #9, 1.899999999999999911 ) ;
#24260=EDGE_CURVE ( 'NONE', #15422, #13616, #28049, .T. ) ;
#24270=CARTESIAN_POINT ( 'NONE',  ( 15.71019289815287934, -3.857619034241787759, 3.790808625284011857 ) ) ;
#24275=CARTESIAN_POINT ( 'NONE',  ( -36.72207054450174724, -5.313409993919712804, -1.009519134730212819 ) ) ;
#24280=DIRECTION ( 'NONE',  ( 0.000000000000000000, 0.000000000000000000, -1.000000000000000000 ) ) ;
#24288=VERTEX_POINT ( 'NONE', #19035 ) ;
#24290=VECTOR ( 'NONE', #11475, 1000.000000000000000 ) ;
#24294=CARTESIAN_POINT ( 'NONE',  ( 54.41118797001386298, -1.084202172485505913E-16, 4.375000000000000000 ) ) ;
#24297=VERTEX_POINT ( 'NONE', #21576 ) ;
#24298=ADVANCED_FACE ( 'NONE', ( #12210 ), #31218, .T. ) ;
#24299=CARTESIAN_POINT ( 'NONE',  ( 51.79427239975815667, -4.149162114478044394, -1.064915450748001646 ) ) ;
#24300=DIRECTION ( 'NONE',  ( 1.000000000000000000, -1.805490781531623600E-17, 1.716160222047040134E-16 ) ) ;
#24305=PLANE ( 'NONE',  #15979 ) ;
#24306=LINE ( 'NONE', #22098, #25524 ) ;
#24307=EDGE_CURVE ( 'NONE', #16732, #2659, #10352, .T. ) ;
#24316=EDGE_CURVE ( 'NONE', #1935, #7270, #9369, .T. ) ;
#24322=ORIENTED_EDGE ( 'NONE', *, *, #2200, .T. ) ;
#24325=ORIENTED_EDGE ( 'NONE', *, *, #15982, .F. ) ;
#24330=B_SPLINE_CURVE_WITH_KNOTS ( 'NONE', 3,
 ( #17032, #4986, #14639, #21943, #5452, #20018, #17480, #12562, #24759, #7665, #5133, #27132, #22396, #3389, #13035, #29208 ),
 .UNSPECIFIED., .F., .F.,
 ( 4, 3, 3, 3, 3, 4 ),
 ( 0.000000000000000000, 1.625241835515689952E-05, 3.292491922809579385E-05, 5.060195339673861708E-05, 6.961003767230190245E-05, 8.476187580399473969E-05 ),
 .UNSPECIFIED. ) ;
#24337=DIRECTION ( 'NONE',  ( 1.000000000000000000, 0.000000000000000000, 0.000000000000000000 ) ) ;
#24343=CARTESIAN_POINT ( 'NONE',  ( 57.00873807961998097, -0.7491996424029042645, -2.489992076190610248 ) ) ;
#24344=CARTESIAN_POINT ( 'NONE',  ( -36.56390771145616725, -3.008101665203226638, -4.495550615867749400 ) ) ;
#24350=CARTESIAN_POINT ( 'NONE',  ( 15.98305126557428579, 0.5375162698823215957, -5.381098085087392846 ) ) ;
#24356=DIRECTION ( 'NONE',  ( -1.000000000000000000, 0.000000000000000000, 0.000000000000000000 ) ) ;
#24357=CARTESIAN_POINT ( 'NONE',  ( 58.45000000000001705, -0.8000000000000000444, 2.421260002560649660 ) ) ;
#24358=AXIS2_PLACEMENT_3D ( 'NONE', #10664, #19861, #17803 ) ;
#24365=CARTESIAN_POINT ( 'NONE',  ( 15.03925126672132961, -2.199885893005931070, -4.939696249117691451 ) ) ;
#24368=PLANE ( 'NONE',  #22805 ) ;
#24374=EDGE_CURVE ( 'NONE', #24537, #5072, #5070, .T. ) ;
#24375=CARTESIAN_POINT ( 'NONE',  ( 48.50000000000002132, 1.409787217987196861, -3.850000000000022737 ) ) ;
#24377=EDGE_CURVE ( 'NONE', #3532, #28342, #7755, .T. ) ;
#24378=AXIS2_PLACEMENT_3D ( 'NONE', #13064, #3095, #25093 ) ;
#24379=DIRECTION ( 'NONE',  ( 0.000000000000000000, 0.9495137264943719346, -0.3137254901960807585 ) ) ;
#24384=ORIENTED_EDGE ( 'NONE', *, *, #8144, .T. ) ;
#24387=CARTESIAN_POINT ( 'NONE',  ( 15.68751737981894934, -2.884962146574149511, -4.577321775072947574 ) ) ;
#24390=EDGE_LOOP ( 'NONE', ( #10789, #13808, #4147, #11217 ) ) ;
#24391=VERTEX_POINT ( 'NONE', #10145 ) ;
#24397=CARTESIAN_POINT ( 'NONE',  ( -36.30347965937280463, -4.980680447166691671, -1.498595263773966790 ) ) ;
#24399=SURFACE_SIDE_STYLE ('',( #2232 ) ) ;
#24404=CARTESIAN_POINT ( 'NONE',  ( 50.33625478868709990, 1.419210040599422795, 3.846553521706499446 ) ) ;
#24406=CARTESIAN_POINT ( 'NONE',  ( -54.45495050826418293, -1.500000000000000000, 3.300094695611020867 ) ) ;
#24407=CARTESIAN_POINT ( 'NONE',  ( 51.87921884176515164, -4.254539148539595139, -1.020319270753726526 ) ) ;
#24411=CARTESIAN_POINT ( 'NONE',  ( -36.89250464418362441, 0.3169205264057852189, -5.400007398663901448 ) ) ;
#24412=EDGE_CURVE ( 'NONE', #3198, #15422, #12346, .T. ) ;
#24415=CARTESIAN_POINT ( 'NONE',  ( 15.41586008885035319, 4.863061488092564666, -1.860589201779632607 ) ) ;
#24416=CARTESIAN_POINT ( 'NONE',  ( 57.05000000000001847, -0.8156862745098039102, 2.468735688885368873 ) ) ;
#24420=CARTESIAN_POINT ( 'NONE',  ( 48.40000000000002700, -0.6462379109120522935, 4.048750000000028493 ) ) ;
#24421=DIRECTION ( 'NONE',  ( 1.000000000000000000, 4.678365685400793326E-16, -1.520093157366863638E-16 ) ) ;
#24423=VERTEX_POINT ( 'NONE', #176 ) ;
#24429=ORIENTED_EDGE ( 'NONE', *, *, #21348, .T. ) ;
#24430=DIRECTION ( 'NONE',  ( -0.000000000000000000, -0.000000000000000000, 1.000000000000000000 ) ) ;
#24435=CARTESIAN_POINT ( 'NONE',  ( 54.46244440770933437, -0.0007103938889471558219, 4.353106894003209604 ) ) ;
#24436=AXIS2_PLACEMENT_3D ( 'NONE', #8185, #10567, #15462 ) ;
#24442=CARTESIAN_POINT ( 'NONE',  ( -54.49409853110120139, -1.525884777627347644, 4.047834655405393889 ) ) ;
#24447=CARTESIAN_POINT ( 'NONE',  ( 57.00000000000001421, 0.7500000000000000000, 3.499999999999999556 ) ) ;
#24464=VERTEX_POINT ( 'NONE', #30455 ) ;
#24469=ORIENTED_EDGE ( 'NONE', *, *, #12019, .T. ) ;
#24471=DIRECTION ( 'NONE',  ( 0.000000000000000000, 0.000000000000000000, -1.000000000000000000 ) ) ;
#24472=CARTESIAN_POINT ( 'NONE',  ( 15.87128154250934031, -5.321612844166236478, -0.9647713018064705270 ) ) ;
#24477=CARTESIAN_POINT ( 'NONE',  ( 50.31877865969198638, 1.391940262981064214, -3.850000000000022293 ) ) ;
#24480=CARTESIAN_POINT ( 'NONE',  ( 16.10667815269233216, -5.098435263432253173, -1.807398698456192276 ) ) ;
#24493=CARTESIAN_POINT ( 'NONE',  ( 48.43326094847141405, 1.398826622412688403, 3.854114288381606190 ) ) ;
#24495=SPHERICAL_SURFACE ( 'NONE', #16159, 0.05000000000000000278 ) ;
#24496=ORIENTED_EDGE ( 'NONE', *, *, #4763, .F. ) ;
#24500=CARTESIAN_POINT ( 'NONE',  ( -54.49998548284560940, -1.548795215916124013, -4.063650232134933482 ) ) ;
#24503=CARTESIAN_POINT ( 'NONE',  ( -35.85663232820584057, 0.000000000000000000, 5.200000000000000178 ) ) ;
#24507=FACE_OUTER_BOUND ( 'NONE', #24390, .T. ) ;
#24513=CARTESIAN_POINT ( 'NONE',  ( 15.74504787372189263, -3.350344226587724794, 4.246692235171886765 ) ) ;
#24528=CARTESIAN_POINT ( 'NONE',  ( 15.49702763512083870, -3.100731772197800495, -4.174739983989899095 ) ) ;
#24535=AXIS2_PLACEMENT_3D ( 'NONE', #816, #15072, #13154 ) ;
#24537=VERTEX_POINT ( 'NONE', #15481 ) ;
#24540=ADVANCED_FACE ( 'NONE', ( #12935 ), #17457, .T. ) ;
#24545=CARTESIAN_POINT ( 'NONE',  ( 48.50000000000002132, -1.391941090707485396, -3.850000000000022737 ) ) ;
#24551=CARTESIAN_POINT ( 'NONE',  ( 48.34352038844360777, -1.212999249975891258, -3.917061424767716016 ) ) ;
#24559=CARTESIAN_POINT ( 'NONE',  ( 15.03925126672132961, -2.199885893005945725, 4.939696249117685234 ) ) ;
#24560=AXIS2_PLACEMENT_3D ( 'NONE', #12862, #25523, #23180 ) ;
#24562=CARTESIAN_POINT ( 'NONE',  ( 56.95000043478394502, -0.7674401070440159955, 2.484784916619714679 ) ) ;
#24567=CARTESIAN_POINT ( 'NONE',  ( 15.57907767661750498, 3.590618801409606320, -4.051716037497242517 ) ) ;
#24570=ORIENTED_EDGE ( 'NONE', *, *, #5168, .F. ) ;
#24574=CARTESIAN_POINT ( 'NONE',  ( 15.03925126672133139, -4.683225679163343536, 2.703237727951232294 ) ) ;
#24579=CARTESIAN_POINT ( 'NONE',  ( 15.67083574136752055, 5.256402525809845905, 1.287848407636934089 ) ) ;
#24582=DIRECTION ( 'NONE',  ( 1.000000000000000000, -0.000000000000000000, -0.000000000000000000 ) ) ;
#24584=VERTEX_POINT ( 'NONE', #28411 ) ;
#24586=CARTESIAN_POINT ( 'NONE',  ( 54.44364453144186911, -0.0003028757503198298978, 4.365665911209477557 ) ) ;
#24592=CIRCLE ( 'NONE', #20070, 0.04999999999999991257 ) ;
#24598=CARTESIAN_POINT ( 'NONE',  ( -54.49999999999997868, -1.549999999999999600, -4.064480286580312907 ) ) ;
#24605=VECTOR ( 'NONE', #4277, 1000.000000000000000 ) ;
#24609=VECTOR ( 'NONE', #8248, 1000.000000000000000 ) ;
#24615=VERTEX_POINT ( 'NONE', #28697 ) ;
#24631=AXIS2_PLACEMENT_3D ( 'NONE', #27617, #15747, #5945 ) ;
#24632=CARTESIAN_POINT ( 'NONE',  ( 57.00000000000001421, -0.6999999999999999556, -2.489477856900920383 ) ) ;
#24633=ORIENTED_EDGE ( 'NONE', *, *, #22286, .F. ) ;
#24639=AXIS2_PLACEMENT_3D ( 'NONE', #444, #14999, #10106 ) ;
#24642=AXIS2_PLACEMENT_3D ( 'NONE', #3108, #14397, #17528 ) ;
#24645=CARTESIAN_POINT ( 'NONE',  ( 50.37749466183669256, 1.328329461116619425, -3.879000873601229138 ) ) ;
#24646=LINE ( 'NONE', #2959, #8867 ) ;
#24654=CARTESIAN_POINT ( 'NONE',  ( 50.30000000000001847, 1.426739617975221641, -3.843750000000023093 ) ) ;
#24663=DIRECTION ( 'NONE',  ( -1.000000000000000000, -0.000000000000000000, -0.000000000000000000 ) ) ;
#24666=SPHERICAL_SURFACE ( 'NONE', #16056, 0.05000000000000000278 ) ;
#24672=CARTESIAN_POINT ( 'NONE',  ( 56.99280487254718253, -0.7628505807388673565, 1.740142286037820618 ) ) ;
#24674=CARTESIAN_POINT ( 'NONE',  ( 34.50000000000001421, 0.000000000000000000, -3.200000000000000178 ) ) ;
#24675=DIRECTION ( 'NONE',  ( -1.000000000000000000, -0.000000000000000000, -0.000000000000000000 ) ) ;
#24676=DIRECTION ( 'NONE',  ( 0.000000000000000000, 0.000000000000000000, -1.000000000000000000 ) ) ;
#24678=VERTEX_POINT ( 'NONE', #14591 ) ;
#24681=CARTESIAN_POINT ( 'NONE',  ( 15.48609859788820131, 2.964363692626647673, 4.273817190665822885 ) ) ;
#24694=CARTESIAN_POINT ( 'NONE',  ( 15.03925126672133139, -3.779372838781759558, -3.883777296072569385 ) ) ;
#24697=EDGE_LOOP ( 'NONE', ( #5215, #28808, #10068 ) ) ;
#24701=LINE ( 'NONE', #30934, #17187 ) ;
#24702=ORIENTED_EDGE ( 'NONE', *, *, #13274, .T. ) ;
#24711=EDGE_CURVE ( 'NONE', #14148, #3532, #1284, .T. ) ;
#24714=CARTESIAN_POINT ( 'NONE',  ( 48.50000000000002132, -1.426739617975179897, -3.843750000000022649 ) ) ;
#24715=CARTESIAN_POINT ( 'NONE',  ( -54.49998431799114940, -1.548747819918199209, 3.331336553795240185 ) ) ;
#24724=CARTESIAN_POINT ( 'NONE',  ( 54.49070678691090563, -0.001831363507897020146, -4.318560329337371329 ) ) ;
#24725=CARTESIAN_POINT ( 'NONE',  ( 57.00000000000001421, -0.7263196003080392149, 2.437012689524181486 ) ) ;
#24726=EDGE_LOOP ( 'NONE', ( #7216, #21240, #20035, #20861 ) ) ;
#24731=CARTESIAN_POINT ( 'NONE',  ( 15.49702763512083514, 3.012234853004126300, -4.239036759381555441 ) ) ;
#24733=CARTESIAN_POINT ( 'NONE',  ( 57.00000000000001421, 0.7000000000000006217, 2.452039967047844993 ) ) ;
#24736=CARTESIAN_POINT ( 'NONE',  ( 47.08898448364825384, -4.179189514726507682, 0.9999999999999997780 ) ) ;
#24740=ORIENTED_EDGE ( 'NONE', *, *, #27012, .F. ) ;
#24741=VERTEX_POINT ( 'NONE', #24545 ) ;
#24742=ADVANCED_FACE ( 'NONE', ( #2862 ), #12515, .F. ) ;
#24743=CARTESIAN_POINT ( 'NONE',  ( 15.17256654081411327, 5.086913989685035276, 1.171642050077737585 ) ) ;
#24750=EDGE_LOOP ( 'NONE', ( #10579, #2435, #11944, #11339 ) ) ;
#24751=CARTESIAN_POINT ( 'NONE',  ( 54.42253022455169997, -6.265509904175804647E-05, 4.373069084971676013 ) ) ;
#24754=ORIENTED_EDGE ( 'NONE', *, *, #11976, .T. ) ;
#24755=CARTESIAN_POINT ( 'NONE',  ( 51.70000000000001705, -4.179189514726506793, -1.000000000000000000 ) ) ;
#24757=DIRECTION ( 'NONE',  ( 1.000000000000000000, 0.000000000000000000, 0.000000000000000000 ) ) ;
#24758=DIRECTION ( 'NONE',  ( -1.000000000000000000, -0.000000000000000000, -0.000000000000000000 ) ) ;
#24759=CARTESIAN_POINT ( 'NONE',  ( 57.01173390802158991, -0.7326096616897963543, 2.432492958759772783 ) ) ;
#24760=DIRECTION ( 'NONE',  ( 0.000000000000000000, -0.000000000000000000, 1.000000000000000000 ) ) ;
#24761=CARTESIAN_POINT ( 'NONE',  ( 54.50000000000002132, 1.734723475976807094E-15, 0.000000000000000000 ) ) ;
#24763=CARTESIAN_POINT ( 'NONE',  ( 50.37722501620131510, -1.384253668070385856, -3.859284659399054185 ) ) ;
#24766=DIRECTION ( 'NONE',  ( 1.000000000000000000, 0.000000000000000000, 0.000000000000000000 ) ) ;
#24767=CARTESIAN_POINT ( 'NONE',  ( 48.42277498379876022, -1.384253668070385856, 3.859284659399054185 ) ) ;
#24769=ORIENTED_EDGE ( 'NONE', *, *, #26592, .F. ) ;
#24770=CARTESIAN_POINT ( 'NONE',  ( -54.48833221701376317, 1.517896399908648108, 3.311598511235000153 ) ) ;
#24773=ORIENTED_EDGE ( 'NONE', *, *, #27077, .F. ) ;
#24784=AXIS2_PLACEMENT_3D ( 'NONE', #5785, #22584, #24931 ) ;
#24789=CARTESIAN_POINT ( 'NONE',  ( -45.15971931043468146, 5.755839955992559655E-16, -4.700000000000000178 ) ) ;
#24799=EDGE_CURVE ( 'NONE', #21818, #1995, #16976, .T. ) ;
#24801=CARTESIAN_POINT ( 'NONE',  ( -41.12388279035661753, -5.147405183146891439, 6.303753281455314391E-16 ) ) ;
#24804=CARTESIAN_POINT ( 'NONE',  ( -36.80043232705833844, -3.597789892641473752, -4.037455662930106826 ) ) ;
#24812=VERTEX_POINT ( 'NONE', #18230 ) ;
#24813=DIRECTION ( 'NONE',  ( -1.000000000000000000, -0.000000000000000000, -0.000000000000000000 ) ) ;
#24817=VERTEX_POINT ( 'NONE', #18371 ) ;
#24828=CARTESIAN_POINT ( 'NONE',  ( 15.18459684427940104, 1.123735532908289425, 5.289358697221545391 ) ) ;
#24831=CARTESIAN_POINT ( 'NONE',  ( 15.87128154250955170, 3.738196885377689238, 3.908481927057728456 ) ) ;
#24834=CYLINDRICAL_SURFACE ( 'NONE', #21033, 0.1000000000000000472 ) ;
#24835=FACE_OUTER_BOUND ( 'NONE', #16674, .T. ) ;
#24836=CARTESIAN_POINT ( 'NONE',  ( 36.50000000000002132, 0.000000000000000000, -0.7500000000000001110 ) ) ;
#24837=CARTESIAN_POINT ( 'NONE',  ( 48.48092587705050960, 1.391939743175939048, -3.849999999996903899 ) ) ;
#24840=ORIENTED_EDGE ( 'NONE', *, *, #19292, .T. ) ;
#24842=CARTESIAN_POINT ( 'NONE',  ( 15.30042582489635272, -4.018128186975086891, -3.618665893506916031 ) ) ;
#24844=EDGE_LOOP ( 'NONE', ( #11063, #3246, #6124, #31254 ) ) ;
#24850=CARTESIAN_POINT ( 'NONE',  ( 57.00000000000001421, -0.6999999999999997335, -1.820027472320129514 ) ) ;
#24856=ORIENTED_EDGE ( 'NONE', *, *, #5706, .T. ) ;
#24860=CARTESIAN_POINT ( 'NONE',  ( 15.22842924604220016, 0.7747498452697078042, 5.363501451416292198 ) ) ;
#24861=FACE_OUTER_BOUND ( 'NONE', #16133, .T. ) ;
#24863=VECTOR ( 'NONE', #16867, 1000.000000000000000 ) ;
#24868=EDGE_CURVE ( 'NONE', #20184, #9901, #14933, .T. ) ;
#24870=CARTESIAN_POINT ( 'NONE',  ( 48.40000000000001990, 0.6304760106459513791, -3.950000000000022826 ) ) ;
#24872=CARTESIAN_POINT ( 'NONE',  ( 57.00872446408695993, -0.7491456045391122753, 2.490007504536590588 ) ) ;
#24874=CARTESIAN_POINT ( 'NONE',  ( 50.50000002815836098, -0.7900353715960748424, -4.025797886239748991 ) ) ;
#24876=CARTESIAN_POINT ( 'NONE',  ( 15.61033468494287213, 3.560621078037196519, -4.077054076718805042 ) ) ;
#24881=LINE ( 'NONE', #5731, #25464 ) ;
#24882=EDGE_CURVE ( 'NONE', #13995, #27463, #14423, .T. ) ;
#24885=EDGE_LOOP ( 'NONE', ( #4782, #17007, #17508, #9650 ) ) ;
#24886=EDGE_LOOP ( 'NONE', ( #18487, #9956, #11538, #7224, #881 ) ) ;
#24901=CIRCLE ( 'NONE', #22955, 4.100000000000022737 ) ;
#24902=CARTESIAN_POINT ( 'NONE',  ( 56.95442145253466038, -0.7107037530308675244, -1.762072693003282398 ) ) ;
#24908=EDGE_CURVE ( 'NONE', #10216, #15120, #27044, .T. ) ;
#24925=ORIENTED_EDGE ( 'NONE', *, *, #10250, .T. ) ;
#24926=CARTESIAN_POINT ( 'NONE',  ( 57.05000000000001847, -0.8000000000000002665, 2.421260002560650104 ) ) ;
#24927=ORIENTED_EDGE ( 'NONE', *, *, #3473, .T. ) ;
#24931=DIRECTION ( 'NONE',  ( 0.000000000000000000, 0.000000000000000000, 1.000000000000000000 ) ) ;
#24933=CARTESIAN_POINT ( 'NONE',  ( 15.29384114148407825, -4.822476035523829196, -1.985498375066542476 ) ) ;
#24937=CARTESIAN_POINT ( 'NONE',  ( -54.44999999999997442, 2.818925648462311528E-15, 9.856100559121352825E-17 ) ) ;
#24940=AXIS2_PLACEMENT_3D ( 'NONE', #14862, #3004, #2838 ) ;
#24953=ORIENTED_EDGE ( 'NONE', *, *, #25138, .F. ) ;
#24955=CARTESIAN_POINT ( 'NONE',  ( -36.38139716712352367, -5.370189181195086370, 0.6649548426257814171 ) ) ;
#24960=ORIENTED_EDGE ( 'NONE', *, *, #8715, .T. ) ;
#24965=DIRECTION ( 'NONE',  ( 0.000000000000000000, 0.000000000000000000, 1.000000000000000000 ) ) ;
#24966=CIRCLE ( 'NONE', #9797, 0.05000000000000008604 ) ;
#24976=CARTESIAN_POINT ( 'NONE',  ( 15.45522337368514521, 2.900433254920969706, 4.320265374240213951 ) ) ;
#24977=AXIS2_PLACEMENT_3D ( 'NONE', #19173, #292, #9800 ) ;
#24979=CARTESIAN_POINT ( 'NONE',  ( 54.50000000000002132, 0.000000000000000000, 0.000000000000000000 ) ) ;
#24980=CIRCLE ( 'NONE', #1214, 0.04999999999999991257 ) ;
#24983=CARTESIAN_POINT ( 'NONE',  ( 48.39081772275598325, 1.198378070452247091, -3.921585382223974570 ) ) ;
#24992=ORIENTED_EDGE ( 'NONE', *, *, #27322, .F. ) ;
#24998=CARTESIAN_POINT ( 'NONE',  ( 50.36640492253749102, 1.250162886418204389, 3.874884102585954171 ) ) ;
#24999=AXIS2_PLACEMENT_3D ( 'NONE', #31119, #23855, #9452 ) ;
#25002=SHAPE_DEFINITION_REPRESENTATION ( #26044, #18201 ) ;
#25006=AXIS2_PLACEMENT_3D ( 'NONE', #8966, #6749, #8792 ) ;
#25010=AXIS2_PLACEMENT_3D ( 'NONE', #1749, #11419, #30099 ) ;
#25011=CARTESIAN_POINT ( 'NONE',  ( 48.44664364291948999, -1.310522848978938670, -3.864668279552719632 ) ) ;
#25012=CARTESIAN_POINT ( 'NONE',  ( 15.17214319754858387, -0.4576450703117617702, 5.200000005133924574 ) ) ;
#25017=CIRCLE ( 'NONE', #23036, 5.147405183146873675 ) ;
#25022=ORIENTED_EDGE ( 'NONE', *, *, #12321, .F. ) ;
#25025=CARTESIAN_POINT ( 'NONE',  ( -36.92405921417682890, 3.062358472872086956, -4.459001320275544522 ) ) ;
#25026=CARTESIAN_POINT ( 'NONE',  ( 15.22780280894146543, 3.779372851356984864, -3.883777284340693026 ) ) ;
#25031=CARTESIAN_POINT ( 'NONE',  ( 51.79999999999820659, 1.279603193924745863, -4.104441627167203066 ) ) ;
#25032=VECTOR ( 'NONE', #13681, 1000.000000000000000 ) ;
#25039=DIRECTION ( 'NONE',  ( -1.000000000000000000, 0.000000000000000000, 0.000000000000000000 ) ) ;
#25049=CIRCLE ( 'NONE', #3315, 0.09999999999999997780 ) ;
#25053=VECTOR ( 'NONE', #27560, 1000.000000000000000 ) ;
#25058=CIRCLE ( 'NONE', #28093, 1.000000000000000000 ) ;
#25062=CARTESIAN_POINT ( 'NONE',  ( 50.45717930666027229, -1.210123066480733200, -3.917958458743180827 ) ) ;
#25065=CARTESIAN_POINT ( 'NONE',  ( 36.50000000000002132, 2.296212748401286986E-16, 1.850000000000000089 ) ) ;
#25072=VERTEX_POINT ( 'NONE', #24674 ) ;
#25073=AXIS2_PLACEMENT_3D ( 'NONE', #23020, #25530, #20350 ) ;
#25081=ORIENTED_EDGE ( 'NONE', *, *, #6765, .T. ) ;
#25087=ORIENTED_EDGE ( 'NONE', *, *, #6897, .T. ) ;
#25093=DIRECTION ( 'NONE',  ( 0.000000000000000000, -1.224646799147353947E-16, 1.000000000000000000 ) ) ;
#25094=CARTESIAN_POINT ( 'NONE',  ( 15.56401610563846383, -5.370189181195031303, -0.6649548426260208922 ) ) ;
#25117=VERTEX_POINT ( 'NONE', #1539 ) ;
#25119=ORIENTED_EDGE ( 'NONE', *, *, #1905, .F. ) ;
#25122=DIRECTION ( 'NONE',  ( 0.000000000000000000, -1.000000000000000000, 0.000000000000000000 ) ) ;
#25125=CIRCLE ( 'NONE', #9971, 4.284222560975607053 ) ;
#25133=DIRECTION ( 'NONE',  ( 1.000000000000000000, 2.586136946169074517E-16, -0.000000000000000000 ) ) ;
#25134=FACE_OUTER_BOUND ( 'NONE', #26824, .T. ) ;
#25137=DIRECTION ( 'NONE',  ( 0.000000000000000000, 0.000000000000000000, 1.000000000000000000 ) ) ;
#25138=EDGE_CURVE ( 'NONE', #11503, #18794, #11920, .T. ) ;
#25147=VERTEX_POINT ( 'NONE', #27678 ) ;
#25149=AXIS2_PLACEMENT_3D ( 'NONE', #11822, #4068, #23866 ) ;
#25151=PLANE ( 'NONE',  #29616 ) ;
#25167=CARTESIAN_POINT ( 'NONE',  ( 57.05000000000001847, 0.7500000000000000000, -2.421260002560649660 ) ) ;
#25168=LINE ( 'NONE', #1098, #28824 ) ;
#25170=EDGE_LOOP ( 'NONE', ( #12704, #26499, #5261, #30903 ) ) ;
#25179=EDGE_CURVE ( 'NONE', #13619, #13291, #1235, .T. ) ;
#25187=CARTESIAN_POINT ( 'NONE',  ( 48.30261087823118515, -0.9335627837657933803, -3.994936164801341061 ) ) ;
#25190=CARTESIAN_POINT ( 'NONE',  ( -35.85663232820584767, 4.683225679163309785, 2.703237727951257607 ) ) ;
#25191=AXIS2_PLACEMENT_3D ( 'NONE', #30555, #13612, #6344 ) ;
#25192=AXIS2_PLACEMENT_3D ( 'NONE', #16026, #27580, #15570 ) ;
#25197=EDGE_CURVE ( 'NONE', #18572, #28342, #20501, .T. ) ;
#25199=CARTESIAN_POINT ( 'NONE',  ( 50.37798322691364916, -1.327156576403582644, -3.879406274192440218 ) ) ;
#25200=CARTESIAN_POINT ( 'NONE',  ( -36.40878371307407946, 2.334862116275031596, -4.877703086529530552 ) ) ;
#25206=CARTESIAN_POINT ( 'NONE',  ( 46.99999999999168665, -4.135416958146860722, 1.091811499727122658 ) ) ;
#25209=ORIENTED_EDGE ( 'NONE', *, *, #27628, .F. ) ;
#25210=CARTESIAN_POINT ( 'NONE',  ( 15.32766723174653478, 3.997758138077601942, -3.641634024966042826 ) ) ;
#25213=CARTESIAN_POINT ( 'NONE',  ( 48.40000000000001990, -0.6304760106459033064, 3.950000000000022826 ) ) ;
#25216=ORIENTED_EDGE ( 'NONE', *, *, #22226, .F. ) ;
#25226=FACE_BOUND ( 'NONE', #30261, .T. ) ;
#25227=CYLINDRICAL_SURFACE ( 'NONE', #19608, 4.100000000000022737 ) ;
#25228=CARTESIAN_POINT ( 'NONE',  ( 50.30000000000001847, -1.391941090707485396, -3.750000000000022649 ) ) ;
#25232=CARTESIAN_POINT ( 'NONE',  ( -35.85663232820584057, -3.056483311920867862, 4.206888370749728878 ) ) ;
#25234=CARTESIAN_POINT ( 'NONE',  ( -54.45996984137642727, 1.500763111530253990, -3.300586169551324556 ) ) ;
#25237=CARTESIAN_POINT ( 'NONE',  ( 50.41422517315185559, -1.132063507975291650, 3.941224428058361706 ) ) ;
#25238=CARTESIAN_POINT ( 'NONE',  ( -36.52679053911622020, 0.8934212604923185141, -5.334164326942875789 ) ) ;
#25240=TOROIDAL_SURFACE ( 'NONE', #14623, 4.650000000000000355, 0.05000000000000000278 ) ;
#25241=EDGE_LOOP ( 'NONE', ( #3010, #17932, #30057, #27569 ) ) ;
#25245=CARTESIAN_POINT ( 'NONE',  ( 51.70000000000001705, -3.826179070414207573, -1.000000000000000000 ) ) ;
#25246=VERTEX_POINT ( 'NONE', #21502 ) ;
#25252=ORIENTED_EDGE ( 'NONE', *, *, #7127, .F. ) ;
#25256=AXIS2_PLACEMENT_3D ( 'NONE', #5855, #20599, #3776 ) ;
#25259=EDGE_CURVE ( 'NONE', #11630, #6668, #21548, .T. ) ;
#25261=CARTESIAN_POINT ( 'NONE',  ( 54.40000000000001990, 0.000000000000000000, 0.000000000000000000 ) ) ;
#25264=CARTESIAN_POINT ( 'NONE',  ( 48.43364830228694018, 1.250438735127648027, 3.874838289045730910 ) ) ;
#25269=AXIS2_PLACEMENT_3D ( 'NONE', #10654, #524, #12848 ) ;
#25275=VERTEX_POINT ( 'NONE', #4548 ) ;
#25276=EDGE_CURVE ( 'NONE', #3572, #20361, #22401, .T. ) ;
#25281=CARTESIAN_POINT ( 'NONE',  ( 15.87128154250933321, -0.7269167730139459715, -5.359285300587695033 ) ) ;
#25282=CARTESIAN_POINT ( 'NONE',  ( -36.68866260399369850, -5.321612844166216938, 0.9647713018066813584 ) ) ;
#25283=DIRECTION ( 'NONE',  ( 1.000000000000000000, 0.000000000000000000, 4.738179285253040686E-16 ) ) ;
#25284=CARTESIAN_POINT ( 'NONE',  ( -35.85663232820584057, -1.854603232583471356E-14, -5.200000000000000178 ) ) ;
#25288=CARTESIAN_POINT ( 'NONE',  ( 57.02942257420237837, -0.7458803891215903814, -1.782029179052657009 ) ) ;
#25294=ORIENTED_EDGE ( 'NONE', *, *, #25782, .F. ) ;
#25295=DIRECTION ( 'NONE',  ( 1.000000000000000000, -0.000000000000000000, 0.000000000000000000 ) ) ;
#25298=CARTESIAN_POINT ( 'NONE',  ( -54.49999999999997868, 0.000000000000000000, 0.000000000000000000 ) ) ;
#25303=B_SPLINE_CURVE_WITH_KNOTS ( 'NONE', 3,
 ( #14007, #21176, #9439, #23698, #26369, #11655 ),
 .UNSPECIFIED., .F., .F.,
 ( 4, 2, 4 ),
 ( 0.000000000000000000, 0.0001614717865051788824, 0.0003229435730103577648 ),
 .UNSPECIFIED. ) ;
#25306=CARTESIAN_POINT ( 'NONE',  ( -44.49999999999997868, -1.499999999999999556, 4.029888335921975262 ) ) ;
#25313=AXIS2_PLACEMENT_3D ( 'NONE', #380, #12705, #3212 ) ;
#25316=FACE_OUTER_BOUND ( 'NONE', #11780, .T. ) ;
#25320=CARTESIAN_POINT ( 'NONE',  ( 48.45124641917420405, 1.383300983803913198, 3.859740869727656953 ) ) ;
#25324=DIRECTION ( 'NONE',  ( 0.000000000000000000, 0.000000000000000000, -1.000000000000000000 ) ) ;
#25327=DIRECTION ( 'NONE',  ( 0.000000000000000000, 8.881784197001252323E-16, -1.000000000000000000 ) ) ;
#25337=DIRECTION ( 'NONE',  ( -1.000000000000000000, -1.293068473084537258E-16, -0.000000000000000000 ) ) ;
#25338=EDGE_CURVE ( 'NONE', #20361, #28557, #12095, .T. ) ;
#25341=CARTESIAN_POINT ( 'NONE',  ( 15.39414421509789932, -0.2904410314644361724, 5.200000000384604526 ) ) ;
#25343=CARTESIAN_POINT ( 'NONE',  ( -44.49999999999999289, 1.499999999999999556, -3.300094695611021312 ) ) ;
#25344=FACE_OUTER_BOUND ( 'NONE', #21464, .T. ) ;
#25352=CARTESIAN_POINT ( 'NONE',  ( -36.72207054450174013, 2.602043737612699470, -4.741394629686777051 ) ) ;
#25356=ORIENTED_EDGE ( 'NONE', *, *, #9268, .F. ) ;
#25363=DIRECTION ( 'NONE',  ( 0.000000000000000000, 0.000000000000000000, -1.000000000000000000 ) ) ;
#25367=CIRCLE ( 'NONE', #10699, 4.299999999999998046 ) ;
#25379=DIRECTION ( 'NONE',  ( 1.000000000000000000, -0.000000000000000000, -0.000000000000000000 ) ) ;
#25388=CARTESIAN_POINT ( 'NONE',  ( 56.96003682719288008, 0.7597908294545935304, 2.486534234876009553 ) ) ;
#25389=CARTESIAN_POINT ( 'NONE',  ( 48.50000000000002132, -1.426739617975173013, 3.843750000000023093 ) ) ;
#25390=ORIENTED_EDGE ( 'NONE', *, *, #10338, .T. ) ;
#25391=DIRECTION ( 'NONE',  ( 0.000000000000000000, 0.000000000000000000, -1.000000000000000000 ) ) ;
#25397=FACE_OUTER_BOUND ( 'NONE', #30953, .T. ) ;
#25411=CARTESIAN_POINT ( 'NONE',  ( 15.70940947763170925, 0.8934212604923389422, 5.334164326942875789 ) ) ;
#25420=DIRECTION ( 'NONE',  ( -1.000000000000000000, -0.000000000000000000, -0.000000000000000000 ) ) ;
#25424=AXIS2_PLACEMENT_3D ( 'NONE', #1626, #8749, #23490 ) ;
#25443=CARTESIAN_POINT ( 'NONE',  ( -35.85663232820583346, 3.817150320979498357, 2.203324261493436520 ) ) ;
#25450=ADVANCED_FACE ( 'NONE', ( #4961 ), #4793, .T. ) ;
#25451=AXIS2_PLACEMENT_3D ( 'NONE', #1916, #18554, #26138 ) ;
#25453=LINE ( 'NONE', #4080, #5883 ) ;
#25455=EDGE_CURVE ( 'NONE', #26012, #29967, #11456, .T. ) ;
#25456=CARTESIAN_POINT ( 'NONE',  ( 51.80693638829369974, -4.271975761602690547, 0.9446694106403946689 ) ) ;
#25463=CARTESIAN_POINT ( 'NONE',  ( 50.33710128586455568, -1.426739617975172569, 3.843750000000022649 ) ) ;
#25464=VECTOR ( 'NONE', #27740, 1000.000000000000000 ) ;
#25467=EDGE_CURVE ( 'NONE', #24423, #11687, #30774, .T. ) ;
#25469=VERTEX_POINT ( 'NONE', #23667 ) ;
#25472=DIRECTION ( 'NONE',  ( 1.000000000000000000, 0.000000000000000000, 0.000000000000000000 ) ) ;
#25474=CARTESIAN_POINT ( 'NONE',  ( 50.30000000000001847, -1.391941090707485396, 3.750000000000022649 ) ) ;
#25478=ADVANCED_FACE ( 'NONE', ( #27268 ), #7888, .T. ) ;
#25484=DIRECTION ( 'NONE',  ( 1.000000000000000000, 2.586136946169074517E-16, -0.000000000000000000 ) ) ;
#25488=FACE_OUTER_BOUND ( 'NONE', #29873, .T. ) ;
#25489=CARTESIAN_POINT ( 'NONE',  ( -36.11187263677868486, 0.3981319440505239893, -5.199999999410233720 ) ) ;
#25490=AXIS2_PLACEMENT_3D ( 'NONE', #19324, #21864, #28961 ) ;
#25492=CARTESIAN_POINT ( 'NONE',  ( 15.03925126672132961, 0.9159215771349694668, -4.311190327366004382 ) ) ;
#25496=CARTESIAN_POINT ( 'NONE',  ( -36.00201293083839715, 2.199885893005534054, -4.939696249117942806 ) ) ;
#25499=CARTESIAN_POINT ( 'NONE',  ( 15.29954477411491887, -5.377732435184348070, 0.5657657035912492249 ) ) ;
#25500=AXIS2_PLACEMENT_3D ( 'NONE', #28909, #21658, #14654 ) ;
#25505=B_SPLINE_CURVE_WITH_KNOTS ( 'NONE', 3,
 ( #26275, #11708, #11380, #6321, #9184, #21066, #30708, #23280, #21537, #6487, #16305, #25950, #18687, #19003, #4580, #14229 ),
 .UNSPECIFIED., .F., .F.,
 ( 4, 2, 2, 2, 2, 2, 2, 4 ),
 ( 0.000000000000000000, 0.0004351083927046410721, 0.0008702167854092821443, 0.001740433570818564289, 0.002175541963523204819, 0.002610650356227845349, 0.003045758748932484578, 0.003480867141637123807 ),
 .UNSPECIFIED. ) ;
#25508=AXIS2_PLACEMENT_3D ( 'NONE', #5948, #13517, #30607 ) ;
#25510=VERTEX_POINT ( 'NONE', #12379 ) ;
#25512=CARTESIAN_POINT ( 'NONE',  ( -54.44999999999997442, -1.549999999999999600, 4.029888335921975262 ) ) ;
#25519=EDGE_LOOP ( 'NONE', ( #14982, #13928, #14408, #24925 ) ) ;
#25523=DIRECTION ( 'NONE',  ( 1.000000000000000000, 0.000000000000000000, 0.000000000000000000 ) ) ;
#25524=VECTOR ( 'NONE', #7526, 1000.000000000000000 ) ;
#25527=B_SPLINE_CURVE_WITH_KNOTS ( 'NONE', 3,
 ( #6841, #30580, #31232, #18417, #23798, #6370, #16034, #18739, #13641, #16506, #11603, #23647, #1941, #8889, #26164, #26322 ),
 .UNSPECIFIED., .F., .F.,
 ( 4, 3, 3, 3, 3, 4 ),
 ( 0.000000000000000000, 2.806063833126217928E-05, 6.345755872418550124E-05, 9.706205683209630718E-05, 0.0001297115041001252684, 0.0001622821609780518274 ),
 .UNSPECIFIED. ) ;
#25528=CARTESIAN_POINT ( 'NONE',  ( 15.03925126672133139, -5.086913985776151392, 1.171642053949083495 ) ) ;
#25530=DIRECTION ( 'NONE',  ( -2.964772755551650383E-16, 0.9875000000000001554, -0.1576190026614809614 ) ) ;
#25531=CARTESIAN_POINT ( 'NONE',  ( 57.05000000000001847, 0.8156862745098041323, 2.468735688885368873 ) ) ;
#25532=CARTESIAN_POINT ( 'NONE',  ( 48.50000000000002132, 1.391941090707534023, -3.750000000000022649 ) ) ;
#25533=AXIS2_PLACEMENT_3D ( 'NONE', #21709, #14076, #11561 ) ;
#25534=CARTESIAN_POINT ( 'NONE',  ( 50.40000000000001990, 0.6304760106459518232, -3.950000000000022826 ) ) ;
#25550=CIRCLE ( 'NONE', #13899, 1.899999999999999911 ) ;
#25551=CARTESIAN_POINT ( 'NONE',  ( 47.10000000000002274, -3.826179070414207573, -1.000000000000000000 ) ) ;
#25557=ORIENTED_EDGE ( 'NONE', *, *, #2806, .T. ) ;
#25565=DIRECTION ( 'NONE',  ( 0.000000000000000000, 0.000000000000000000, 1.000000000000000000 ) ) ;
#25570=CARTESIAN_POINT ( 'NONE',  ( 51.80641384975955788, -4.235076411889995285, 1.097987773005780321 ) ) ;
#25576=AXIS2_PLACEMENT_3D ( 'NONE', #20015, #22094, #4816 ) ;
#25577=ORIENTED_EDGE ( 'NONE', *, *, #30999, .F. ) ;
#25579=AXIS2_PLACEMENT_3D ( 'NONE', #16355, #21133, #31241 ) ;
#25586=CARTESIAN_POINT ( 'NONE',  ( -36.21152527658241382, 3.291455042465393444, 4.036171416105503340 ) ) ;
#25588=VERTEX_POINT ( 'NONE', #29186 ) ;
#25592=EDGE_LOOP ( 'NONE', ( #14619, #28246 ) ) ;
#25597=DIRECTION ( 'NONE',  ( 1.000000000000000000, 5.570239943078649173E-15, -9.650165233620068940E-15 ) ) ;
#25599=CARTESIAN_POINT ( 'NONE',  ( 33.47623932017462778, 1.734723475976807094E-15, 0.000000000000000000 ) ) ;
#25601=CARTESIAN_POINT ( 'NONE',  ( 57.01079425239058196, 0.7499991164627679563, 1.746008812021272227 ) ) ;
#25612=CIRCLE ( 'NONE', #8445, 4.375000000000000000 ) ;
#25613=AXIS2_PLACEMENT_3D ( 'NONE', #13327, #27769, #10986 ) ;
#25614=CARTESIAN_POINT ( 'NONE',  ( 48.40000000000001990, -0.6304760106459033064, -3.950000000000022826 ) ) ;
#25615=CIRCLE ( 'NONE', #23607, 0.05000000000000017625 ) ;
#25616=CARTESIAN_POINT ( 'NONE',  ( -36.38139716712170468, -1.027070083876041373, 5.312835761376664578 ) ) ;
#25618=ORIENTED_EDGE ( 'NONE', *, *, #11976, .F. ) ;
#25622=ORIENTED_EDGE ( 'NONE', *, *, #12285, .F. ) ;
#25624=CARTESIAN_POINT ( 'NONE',  ( 48.42176022524417789, 1.183413901109590105, 3.885761703493072261 ) ) ;
#25628=CARTESIAN_POINT ( 'NONE',  ( -44.49999999999997868, 2.818925648462311528E-15, 9.856100559121352825E-17 ) ) ;
#25633=DIRECTION ( 'NONE',  ( -1.293068473084537258E-16, 1.000000000000000000, 0.000000000000000000 ) ) ;
#25635=ORIENTED_EDGE ( 'NONE', *, *, #8835, .T. ) ;
#25642=AXIS2_PLACEMENT_3D ( 'NONE', #18189, #10723, #27355 ) ;
#25647=CARTESIAN_POINT ( 'NONE',  ( -36.38139716712352367, 3.953723660658955641, -3.694477770903653369 ) ) ;
#25650=B_SPLINE_CURVE_WITH_KNOTS ( 'NONE', 3,
 ( #13536, #18465, #11308, #20840, #20698, #25888, #9114, #18165, #28102, #4045, #16392, #18784, #1814, #6583, #30324, #8630, #30469, #4191, #11490 ),
 .UNSPECIFIED., .F., .F.,
 ( 4, 3, 3, 3, 3, 3, 4 ),
 ( 0.000000000000000000, 2.270809125664990461E-05, 4.499850898804030560E-05, 6.557565265601914873E-05, 7.920624315363274039E-05, 8.325821076725717102E-05, 9.013793637923205450E-05 ),
 .UNSPECIFIED. ) ;
#25653=AXIS2_PLACEMENT_3D ( 'NONE', #29267, #22156, #4715 ) ;
#25659=DIRECTION ( 'NONE',  ( 0.000000000000000000, 1.000000000000000000, -0.000000000000000000 ) ) ;
#25664=LINE ( 'NONE', #9535, #14072 ) ;
#25669=EDGE_CURVE ( 'NONE', #9539, #10988, #20371, .T. ) ;
#25672=CARTESIAN_POINT ( 'NONE',  ( 50.36024759664407213, -1.282505688586073056, 3.869483523004606518 ) ) ;
#25686=CARTESIAN_POINT ( 'NONE',  ( 57.04536243881683788, 0.7794871794871796045, -1.732743413496389939 ) ) ;
#25690=CARTESIAN_POINT ( 'NONE',  ( -54.44999999999997442, 1.499999999999999556, 4.029888335921975262 ) ) ;
#25692=CARTESIAN_POINT ( 'NONE',  ( -35.85663232820584057, 0.4576450603546802220, -5.200000000000000178 ) ) ;
#25697=CARTESIAN_POINT ( 'NONE',  ( -36.92405921417685732, 5.098435263432259390, -1.807398698456122110 ) ) ;
#25701=DIRECTION ( 'NONE',  ( 1.000000000000000000, -0.000000000000000000, -0.000000000000000000 ) ) ;
#25704=VERTEX_POINT ( 'NONE', #1353 ) ;
#25710=CARTESIAN_POINT ( 'NONE',  ( 58.45000000000001705, -0.8000000000000000444, -1.778341924377873751 ) ) ;
#25713=CARTESIAN_POINT ( 'NONE',  ( 56.95000000000001705, 0.7227197132926967971, -2.497551541979256218 ) ) ;
#25714=ORIENTED_EDGE ( 'NONE', *, *, #17758, .T. ) ;
#25718=ORIENTED_EDGE ( 'NONE', *, *, #2278, .T. ) ;
#25720=VECTOR ( 'NONE', #13402, 1000.000000000000000 ) ;
#25728=CARTESIAN_POINT ( 'NONE',  ( 46.90000017523095011, -4.241673356750442991, -1.073212863078178980 ) ) ;
#25735=LINE ( 'NONE', #4043, #3536 ) ;
#25738=CARTESIAN_POINT ( 'NONE',  ( -36.48174642953024005, -2.847679722116556622, 4.601476325142769497 ) ) ;
#25741=CARTESIAN_POINT ( 'NONE',  ( 51.89999982476908968, -4.241673356750432333, 1.073212863078216506 ) ) ;
#25752=AXIS2_PLACEMENT_3D ( 'NONE', #11869, #29528, #7275 ) ;
#25754=CARTESIAN_POINT ( 'NONE',  ( -36.68133364217572989, 3.736273719777117197, 3.909490113446847381 ) ) ;
#25760=ORIENTED_EDGE ( 'NONE', *, *, #9233, .F. ) ;
#25767=CARTESIAN_POINT ( 'NONE',  ( -36.92405921417686443, -3.062358472872079851, 4.459001320275575608 ) ) ;
#25768=CARTESIAN_POINT ( 'NONE',  ( 57.00000000000001421, 0.6999999999999997335, 1.820027472320129514 ) ) ;
#25773=CARTESIAN_POINT ( 'NONE',  ( 15.03925126672132784, 4.018128179617494133, 3.618665901676702656 ) ) ;
#25782=EDGE_CURVE ( 'NONE', #8110, #11505, #21071, .T. ) ;
#25784=ORIENTED_EDGE ( 'NONE', *, *, #6121, .F. ) ;
#25787=DIRECTION ( 'NONE',  ( 1.000000000000000000, 0.000000000000000000, 0.000000000000000000 ) ) ;
#25791=FACE_OUTER_BOUND ( 'NONE', #3871, .T. ) ;
#25793=DIRECTION ( 'NONE',  ( 0.000000000000000000, 0.000000000000000000, 1.000000000000000000 ) ) ;
#25801=CARTESIAN_POINT ( 'NONE',  ( -54.49998548284560940, 1.548795215916124013, -4.063650232134933482 ) ) ;
#25804=CARTESIAN_POINT ( 'NONE',  ( 57.03906491987265781, -0.7487895892850940927, 1.779428968492786867 ) ) ;
#25806=CARTESIAN_POINT ( 'NONE',  ( -35.85663232820581925, 2.686240680702182360, -4.475885388010699906 ) ) ;
#25807=CARTESIAN_POINT ( 'NONE',  ( -35.85663232820584057, -0.9159215771349644708, 4.311190327366005270 ) ) ;
#25810=CARTESIAN_POINT ( 'NONE',  ( 16.10660252424456829, -0.2875137064282094479, -5.407399902318746676 ) ) ;
#25812=CARTESIAN_POINT ( 'NONE',  ( 51.70000000000001705, -0.1421112804877805724, 1.100000000000005862 ) ) ;
#25816=ORIENTED_EDGE ( 'NONE', *, *, #3991, .T. ) ;
#25818=DIRECTION ( 'NONE',  ( 0.000000000000000000, 0.000000000000000000, -1.000000000000000000 ) ) ;
#25820=CARTESIAN_POINT ( 'NONE',  ( -35.85663232820600399, 4.683225679163309785, 2.703237727951259828 ) ) ;
#25822=VERTEX_POINT ( 'NONE', #28583 ) ;
#25824=CARTESIAN_POINT ( 'NONE',  ( -36.89250464418362441, -5.233646053067086079, 1.367284724151337949 ) ) ;
#25825=CARTESIAN_POINT ( 'NONE',  ( 50.36635169771309961, -1.250438735127598511, 3.874838289045730910 ) ) ;
#25828=AXIS2_PLACEMENT_3D ( 'NONE', #3229, #6545, #18590 ) ;
#25829=ADVANCED_FACE ( 'NONE', ( #26366 ), #27841, .T. ) ;
#25833=TOROIDAL_SURFACE ( 'NONE', #29881, 4.275000000000000355, 0.1000000000000000056 ) ;
#25842=ADVANCED_FACE ( 'NONE', ( #14788 ), #24305, .F. ) ;
#25848=DIRECTION ( 'NONE',  ( 0.000000000000000000, 0.000000000000000000, -1.000000000000000000 ) ) ;
#25853=DIRECTION ( 'NONE',  ( 0.000000000000000000, 6.217248937900876626E-15, 1.000000000000000000 ) ) ;
#25854=CARTESIAN_POINT ( 'NONE',  ( 15.66436536804551061, 5.256245472275793418, -1.286369972357296110 ) ) ;
#25861=CARTESIAN_POINT ( 'NONE',  ( 50.50000002742975624, -0.7904052113206707642, 4.025738854575410919 ) ) ;
#25864=CARTESIAN_POINT ( 'NONE',  ( -44.49999999999997868, 1.499999999999999556, -3.300094695611021312 ) ) ;
#25867=EDGE_LOOP ( 'NONE', ( #11789, #21160, #10285, #25209 ) ) ;
#25868=EDGE_CURVE ( 'NONE', #10898, #26742, #13483, .T. ) ;
#25879=ORIENTED_EDGE ( 'NONE', *, *, #25868, .F. ) ;
#25882=EDGE_CURVE ( 'NONE', #14356, #9001, #18062, .T. ) ;
#25886=EDGE_CURVE ( 'NONE', #16322, #1490, #19582, .T. ) ;
#25888=CARTESIAN_POINT ( 'NONE',  ( 57.00841846112073341, 0.7284616547511407747, -1.797128479182910299 ) ) ;
#25889=CARTESIAN_POINT ( 'NONE',  ( -35.85663232820581925, -2.525801270006313715, 4.794550352686329120 ) ) ;
#25890=CARTESIAN_POINT ( 'NONE',  ( 58.45000000000001705, -0.8000000000000000444, -1.778341924377873751 ) ) ;
#25904=CARTESIAN_POINT ( 'NONE',  ( -36.43290890416756156, 2.776541361171022793, 4.646985486732267745 ) ) ;
#25905=VERTEX_POINT ( 'NONE', #18272 ) ;
#25906=EDGE_CURVE ( 'NONE', #1993, #19631, #19086, .T. ) ;
#25909=CARTESIAN_POINT ( 'NONE',  ( 58.45000000000001705, 0.8000000000000000444, 1.778341924377873751 ) ) ;
#25916=CARTESIAN_POINT ( 'NONE',  ( 57.00000000000001421, -0.7256836306366275524, 1.800271087100996592 ) ) ;
#25921=CARTESIAN_POINT ( 'NONE',  ( 51.82417406112929115, 0.5144554499007042425, 4.312884176178978457 ) ) ;
#25932=CARTESIAN_POINT ( 'NONE',  ( 48.30000000000002558, 0.6462379109120994780, -4.048750000000022276 ) ) ;
#25941=EDGE_LOOP ( 'NONE', ( #5298, #6305, #21101, #30135, #2837 ) ) ;
#25944=DIRECTION ( 'NONE',  ( 0.000000000000000000, -0.000000000000000000, 1.000000000000000000 ) ) ;
#25948=ORIENTED_EDGE ( 'NONE', *, *, #487, .T. ) ;
#25950=CARTESIAN_POINT ( 'NONE',  ( -36.52757395963739384, 3.857619034241715816, 3.790808625284063815 ) ) ;
#25957=CARTESIAN_POINT ( 'NONE',  ( -36.11187263677958725, 3.378578820313965281, -3.972872285093680844 ) ) ;
#25966=CARTESIAN_POINT ( 'NONE',  ( 33.47623932017462778, 4.018128179617509232, 3.618665901676689778 ) ) ;
#25971=DIRECTION ( 'NONE',  ( -1.000000000000000000, -0.000000000000000000, -0.000000000000000000 ) ) ;
#25975=VERTEX_POINT ( 'NONE', #3842 ) ;
#25977=CARTESIAN_POINT ( 'NONE',  ( 50.30000000000001847, -1.391941090707485396, 3.850000000000022737 ) ) ;
#25987=CARTESIAN_POINT ( 'NONE',  ( 0.000000000000000000, 0.000000000000000000, 0.000000000000000000 ) ) ;
#25991=EDGE_CURVE ( 'NONE', #1787, #27011, #14496, .T. ) ;
#25998=CARTESIAN_POINT ( 'NONE',  ( -44.49999999999998579, 9.184850993650734737E-17, 0.7500000000000185407 ) ) ;
#26002=CARTESIAN_POINT ( 'NONE',  ( -36.40878371307407235, -3.917459231545681764, -3.727878977586817744 ) ) ;
#26007=VERTEX_POINT ( 'NONE', #10975 ) ;
#26012=VERTEX_POINT ( 'NONE', #853 ) ;
#26013=CARTESIAN_POINT ( 'NONE',  ( 58.45000000000001705, 0.8000000000000000444, 1.778341924377873751 ) ) ;
#26018=CARTESIAN_POINT ( 'NONE',  ( 15.74504787372188552, 5.074157625981753128, 1.874066637979887373 ) ) ;
#26023=CARTESIAN_POINT ( 'NONE',  ( 58.45000000000001705, -0.8000000000000002665, -2.421260002560650104 ) ) ;
#26024=B_SPLINE_CURVE_WITH_KNOTS ( 'NONE', 3,
 ( #2102, #30769, #1619, #20961, #9079, #9243, #28241, #14293, #18753, #28395, #7182, #11451, #23962, #23482 ),
 .UNSPECIFIED., .F., .F.,
 ( 4, 2, 2, 2, 2, 2, 4 ),
 ( 0.000000000000000000, 0.0003953907277084696219, 0.0005930860915627040805, 0.0006919337734898216080, 0.0007413576144533806428, 0.0007660695349351558233, 0.0007907814554169310039 ),
 .UNSPECIFIED. ) ;
#26026=STYLED_ITEM ( 'NONE', ( #30138 ), #5173 ) ;
#26029=EDGE_LOOP ( 'NONE', ( #19227, #10072, #10751, #27652 ) ) ;
#26031=CARTESIAN_POINT ( 'NONE',  ( 47.00000000000002132, -4.259181259350203419, -1.100000000000000089 ) ) ;
#26033=VECTOR ( 'NONE', #24430, 1000.000000000000000 ) ;
#26042=DIRECTION ( 'NONE',  ( -0.000000000000000000, 0.000000000000000000, -1.000000000000000000 ) ) ;
#26044=PRODUCT_DEFINITION_SHAPE ( 'NONE', 'NONE',  #14745 ) ;
#26046=CYLINDRICAL_SURFACE ( 'NONE', #10508, 3.200000000000000178 ) ;
#26049=AXIS2_PLACEMENT_3D ( 'NONE', #23653, #28710, #26327 ) ;
#26064=ORIENTED_EDGE ( 'NONE', *, *, #25886, .T. ) ;
#26067=VERTEX_POINT ( 'NONE', #25998 ) ;
#26068=CARTESIAN_POINT ( 'NONE',  ( -36.00197790576392975, 4.683225679163309785, 2.703237727951257607 ) ) ;
#26069=LINE ( 'NONE', #18962, #13007 ) ;
#26072=FACE_OUTER_BOUND ( 'NONE', #7675, .T. ) ;
#26073=FACE_BOUND ( 'NONE', #23882, .T. ) ;
#26074=CARTESIAN_POINT ( 'NONE',  ( -54.49454330418567594, -1.526701536696945860, -3.317245250669463630 ) ) ;
#26075=CARTESIAN_POINT ( 'NONE',  ( 57.05000000000001137, 0.7794871794871797155, -1.732743413496401930 ) ) ;
#26077=CARTESIAN_POINT ( 'NONE',  ( 51.80000000000001847, 1.521694824349937303, 3.995005614707771269 ) ) ;
#26080=DIRECTION ( 'NONE',  ( 0.000000000000000000, 1.000000000000000000, 0.000000000000000000 ) ) ;
#26081=DIRECTION ( 'NONE',  ( -0.000000000000000000, 0.9495137264943719346, -0.3137254901960807585 ) ) ;
#26082=AXIS2_PLACEMENT_3D ( 'NONE', #2829, #9974, #12325 ) ;
#26088=EDGE_CURVE ( 'NONE', #9001, #16975, #29493, .T. ) ;
#26091=CARTESIAN_POINT ( 'NONE',  ( -36.77443515226921278, -0.6016956010317862091, 5.375730734456589666 ) ) ;
#26094=CARTESIAN_POINT ( 'NONE',  ( -36.14490256869204643, -5.374748457514320954, 0.5963382560600137827 ) ) ;
#26099=VERTEX_POINT ( 'NONE', #23652 ) ;
#26103=CARTESIAN_POINT ( 'NONE',  ( -45.15971931043468146, 14.70000000000000107, 0.000000000000000000 ) ) ;
#26104=VECTOR ( 'NONE', #7026, 1000.000000000000000 ) ;
#26114=FACE_OUTER_BOUND ( 'NONE', #15506, .T. ) ;
#26117=CARTESIAN_POINT ( 'NONE',  ( 57.00841846112073341, -0.7284616547511407747, 1.797128479182910299 ) ) ;
#26119=CARTESIAN_POINT ( 'NONE',  ( -36.42771574642738841, 2.777216423308057625, -4.646230875016845729 ) ) ;
#26120=CARTESIAN_POINT ( 'NONE',  ( 57.00000000000001421, -0.6999999999999999556, -2.452039967047845437 ) ) ;
#26123=VECTOR ( 'NONE', #9203, 1000.000000000000000 ) ;
#26124=AXIS2_PLACEMENT_3D ( 'NONE', #31073, #29018, #14762 ) ;
#26133=CARTESIAN_POINT ( 'NONE',  ( 33.47623932017462778, -2.199885893005926185, -4.939696249117692339 ) ) ;
#26137=( BOUNDED_SURFACE ( )  B_SPLINE_SURFACE ( 3, 2, ( 
 ( #23552, #1540, #13392 ),
 ( #15941, #25601, #27838 ),
 ( #30835, #30499, #11344 ),
 ( #25768, #23401, #20873 ) ),
 .UNSPECIFIED., .F., .F., .F. ) 
 B_SPLINE_SURFACE_WITH_KNOTS ( ( 4, 4 ),
 ( 3, 3 ),
 ( 6.291704175186453303E-05, 0.0002258017310250082428 ),
 ( 0.000000000000000000, 1.000000000000000000 ),
 .UNSPECIFIED. ) 
 GEOMETRIC_REPRESENTATION_ITEM ( )  RATIONAL_B_SPLINE_SURFACE ( (
 ( 1.000000000000000000, 0.8397191227596314533, 1.000000000000000000),
 ( 1.000000000000000000, 0.8408372669632975249, 1.000000000000000000),
 ( 1.000000000000000000, 0.7715695853058209819, 1.000000000000000000),
 ( 1.000000000000000000, 0.7071067811864981678, 1.000000000000000000) ) ) 
 REPRESENTATION_ITEM ( '' )  SURFACE ( )  );
#26138=DIRECTION ( 'NONE',  ( 0.000000000000000000, 0.000000000000000000, 1.000000000000000000 ) ) ;
#26139=CARTESIAN_POINT ( 'NONE',  ( 15.17214319754843110, -2.686240675664388622, -4.475885398016685279 ) ) ;
#26140=CARTESIAN_POINT ( 'NONE',  ( -36.80043232705879319, 5.283830060792378269, 1.151642405604297981 ) ) ;
#26144=CARTESIAN_POINT ( 'NONE',  ( -36.22955757456080761, -4.863043649742761154, 1.860644097022644994 ) ) ;
#26145=FACE_OUTER_BOUND ( 'NONE', #21269, .T. ) ;
#26152=VERTEX_POINT ( 'NONE', #24110 ) ;
#26161=CIRCLE ( 'NONE', #12994, 4.700000000000000178 ) ;
#26164=CARTESIAN_POINT ( 'NONE',  ( 57.03920447585827702, -0.8156862745098039102, 2.468735688885368429 ) ) ;
#26169=CARTESIAN_POINT ( 'NONE',  ( -36.92398358572908279, 5.231589534716062140, -1.397536681175157502 ) ) ;
#26171=CIRCLE ( 'NONE', #22641, 1.949999999999999956 ) ;
#26172=VECTOR ( 'NONE', #16925, 1000.000000000000000 ) ;
#26174=DIRECTION ( 'NONE',  ( 0.000000000000000000, 0.000000000000000000, -1.000000000000000000 ) ) ;
#26178=VECTOR ( 'NONE', #21882, 1000.000000000000000 ) ;
#26179=CARTESIAN_POINT ( 'NONE',  ( 56.99368740573074632, 0.8156852809530760195, -2.468736017162952656 ) ) ;
#26182=CARTESIAN_POINT ( 'NONE',  ( 48.50000000000354561, -1.426739617988837194, 3.843749999997122746 ) ) ;
#26184=DIRECTION ( 'NONE',  ( 1.000000000000000000, -0.000000000000000000, -0.000000000000000000 ) ) ;
#26187=ORIENTED_EDGE ( 'NONE', *, *, #15795, .F. ) ;
#26188=DIRECTION ( 'NONE',  ( 1.000000000000000000, 0.000000000000000000, 0.000000000000000000 ) ) ;
#26192=ORIENTED_EDGE ( 'NONE', *, *, #28454, .T. ) ;
#26195=DIRECTION ( 'NONE',  ( 1.000000000000000000, 0.000000000000000000, 0.000000000000000000 ) ) ;
#26206=ORIENTED_EDGE ( 'NONE', *, *, #16497, .T. ) ;
#26209=ADVANCED_FACE ( 'NONE', ( #21907 ), #26794, .T. ) ;
#26211=CARTESIAN_POINT ( 'NONE',  ( -36.63359589171324870, -2.513248512186274652, 4.788125582312047435 ) ) ;
#26221=CARTESIAN_POINT ( 'NONE',  ( 51.80349172417631110, 1.030408547777236894, -4.190799094670026648 ) ) ;
#26225=DIRECTION ( 'NONE',  ( 0.000000000000000000, 2.168404344971012812E-15, 1.000000000000000000 ) ) ;
#26226=CARTESIAN_POINT ( 'NONE',  ( -36.11692583559974423, 4.018128194440848233, 3.618665885216990397 ) ) ;
#26233=CARTESIAN_POINT ( 'NONE',  ( 50.41047473690881731, 0.7808213810458778381, 4.027268569371624807 ) ) ;
#26238=FACE_BOUND ( 'NONE', #4231, .T. ) ;
#26252=EDGE_LOOP ( 'NONE', ( #5809, #4456, #994, #15399, #17614, #15601, #8585, #3011, #19511, #16895 ) ) ;
#26256=EDGE_LOOP ( 'NONE', ( #30022, #29480, #22406, #20170 ) ) ;
#26258=CARTESIAN_POINT ( 'NONE',  ( -36.14504829323105639, -4.698774973472870542, 2.676767126782095385 ) ) ;
#26259=ORIENTED_EDGE ( 'NONE', *, *, #19292, .F. ) ;
#26264=VERTEX_POINT ( 'NONE', #2245 ) ;
#26273=DIRECTION ( 'NONE',  ( 1.000000000000000000, 0.000000000000000000, 0.000000000000000000 ) ) ;
#26275=CARTESIAN_POINT ( 'NONE',  ( -35.85663232820584057, 2.199885893005902204, 4.939696249117695892 ) ) ;
#26279=CARTESIAN_POINT ( 'NONE',  ( -35.85663232820584057, -4.945493884734804446, -1.606888370749739448 ) ) ;
#26282=CARTESIAN_POINT ( 'NONE',  ( -35.85663232820581925, 2.525801270006329702, -4.794550352686303363 ) ) ;
#26283=EDGE_CURVE ( 'NONE', #8004, #26599, #1886, .T. ) ;
#26284=CARTESIAN_POINT ( 'NONE',  ( 57.00000000000001421, 0.6999999999999999556, 1.820027472320129736 ) ) ;
#26297=CARTESIAN_POINT ( 'NONE',  ( 33.47623932017462778, 1.734723475976807094E-15, 0.000000000000000000 ) ) ;
#26298=CARTESIAN_POINT ( 'NONE',  ( 51.80000000000001847, -4.131056160354152240, -1.100000000000000089 ) ) ;
#26299=CARTESIAN_POINT ( 'NONE',  ( 15.48609859788817467, -2.964363692626676094, -4.273817190665769594 ) ) ;
#26300=CARTESIAN_POINT ( 'NONE',  ( -36.56390771145526486, 5.076023720898184877, 1.868859051106935398 ) ) ;
#26301=CARTESIAN_POINT ( 'NONE',  ( 15.17256654081411682, -4.804073784580274342, 2.042134692980114963 ) ) ;
#26302=VERTEX_POINT ( 'NONE', #26639 ) ;
#26306=ORIENTED_EDGE ( 'NONE', *, *, #9072, .T. ) ;
#26307=CARTESIAN_POINT ( 'NONE',  ( 56.95640338720422591, 0.7513613876702617267, -2.489093304807997509 ) ) ;
#26312=ORIENTED_EDGE ( 'NONE', *, *, #29545, .F. ) ;
#26315=ORIENTED_EDGE ( 'NONE', *, *, #6684, .T. ) ;
#26320=AXIS2_PLACEMENT_3D ( 'NONE', #23043, #30154, #8761 ) ;
#26322=CARTESIAN_POINT ( 'NONE',  ( 57.05000000000001847, -0.8156862745098041323, 2.468735688885368873 ) ) ;
#26325=LINE ( 'NONE', #16834, #23145 ) ;
#26327=DIRECTION ( 'NONE',  ( 0.000000000000000000, 0.000000000000000000, 1.000000000000000000 ) ) ;
#26331=CARTESIAN_POINT ( 'NONE',  ( 54.40000000000001990, -0.2842225609755594795, -1.577752156565102655E-15 ) ) ;
#26332=EDGE_LOOP ( 'NONE', ( #11777, #3300, #4244, #14298 ) ) ;
#26336=CARTESIAN_POINT ( 'NONE',  ( 48.41300975153458097, -1.088846059295756508, -3.899771020632008423 ) ) ;
#26339=VECTOR ( 'NONE', #26961, 1000.000000000000000 ) ;
#26346=EDGE_CURVE ( 'NONE', #14356, #22384, #13284, .T. ) ;
#26347=CYLINDRICAL_SURFACE ( 'NONE', #27042, 1.000000000000000000 ) ;
#26348=VERTEX_POINT ( 'NONE', #25343 ) ;
#26350=DIRECTION ( 'NONE',  ( -1.000000000000000000, -0.000000000000000000, -0.000000000000000000 ) ) ;
#26359=CARTESIAN_POINT ( 'NONE',  ( -44.49999999999999289, 0.000000000000000000, 0.000000000000000000 ) ) ;
#26362=CARTESIAN_POINT ( 'NONE',  ( 56.97542489291938494, 0.7477441023849552559, 1.746698826563745977 ) ) ;
#26366=FACE_OUTER_BOUND ( 'NONE', #13096, .T. ) ;
#26367=DIRECTION ( 'NONE',  ( 0.000000000000000000, 0.000000000000000000, 1.000000000000000000 ) ) ;
#26368=CARTESIAN_POINT ( 'NONE',  ( 51.70000000000001705, -4.259946800035238290, 0.9999999999999995559 ) ) ;
#26369=CARTESIAN_POINT ( 'NONE',  ( 47.04572677324562591, -4.276948333784439171, 0.9210526315789451246 ) ) ;
#26374=AXIS2_PLACEMENT_3D ( 'NONE', #13214, #13679, #11012 ) ;
#26377=FACE_OUTER_BOUND ( 'NONE', #16226, .T. ) ;
#26388=CARTESIAN_POINT ( 'NONE',  ( 50.40000000000001279, 0.6462379109120992560, 4.048750000000022276 ) ) ;
#26391=CARTESIAN_POINT ( 'NONE',  ( 57.05000000000001137, -0.7500000000000002220, 1.746008434843742796 ) ) ;
#26392=CARTESIAN_POINT ( 'NONE',  ( 57.00221072626734298, 0.7147032416868923654, 1.808443027029684291 ) ) ;
#26395=CARTESIAN_POINT ( 'NONE',  ( -44.49999999999997868, -1.499999999999999556, -4.029888335921975262 ) ) ;
#26399=CIRCLE ( 'NONE', #7196, 1.000000000000000000 ) ;
#26406=ORIENTED_EDGE ( 'NONE', *, *, #26820, .T. ) ;
#26410=ORIENTED_EDGE ( 'NONE', *, *, #18730, .T. ) ;
#26427=CARTESIAN_POINT ( 'NONE',  ( 15.03925126672132961, -4.018128179617538542, -3.618665901676658248 ) ) ;
#26429=CARTESIAN_POINT ( 'NONE',  ( -54.49999999999997868, 0.000000000000000000, 0.000000000000000000 ) ) ;
#26436=CARTESIAN_POINT ( 'NONE',  ( 15.22780280894162708, -3.779372851356274765, 3.883777284340669045 ) ) ;
#26440=DIRECTION ( 'NONE',  ( -1.000000000000000000, -2.586136946169074517E-16, 0.000000000000000000 ) ) ;
#26444=CARTESIAN_POINT ( 'NONE',  ( 15.03925126672132961, 7.778712668717615929E-15, -5.200000000000000178 ) ) ;
#26446=ORIENTED_EDGE ( 'NONE', *, *, #17811, .F. ) ;
#26447=DIRECTION ( 'NONE',  ( 0.000000000000000000, 0.000000000000000000, -1.000000000000000000 ) ) ;
#26448=CARTESIAN_POINT ( 'NONE',  ( 50.50000000000002132, -0.7901969350669644232, 4.025772098418840095 ) ) ;
#26451=CARTESIAN_POINT ( 'NONE',  ( -35.85663232820581925, 5.340403872473301838, 0.9205822173396537300 ) ) ;
#26452=CARTESIAN_POINT ( 'NONE',  ( 15.30042582489636160, -4.683225673667250177, 2.703237737472941493 ) ) ;
#26459=ADVANCED_FACE ( 'NONE', ( #25488 ), #18859, .F. ) ;
#26461=EDGE_LOOP ( 'NONE', ( #15266, #12128, #13011, #29058, #25216 ) ) ;
#26470=AXIS2_PLACEMENT_3D ( 'NONE', #26297, #4598, #26447 ) ;
#26471=CARTESIAN_POINT ( 'NONE',  ( -54.49454330418567594, -1.526701536696946082, 3.317245250669463630 ) ) ;
#26477=CARTESIAN_POINT ( 'NONE',  ( 47.01039059310604529, -4.157292525004591788, 1.048498855808312813 ) ) ;
#26481=ORIENTED_EDGE ( 'NONE', *, *, #10430, .F. ) ;
#26490=VECTOR ( 'NONE', #8714, 1000.000000000000000 ) ;
#26494=ORIENTED_EDGE ( 'NONE', *, *, #14228, .F. ) ;
#26495=CARTESIAN_POINT ( 'NONE',  ( 15.81621483022873420, 4.847650360853553053, 2.396424556482827928 ) ) ;
#26496=ORIENTED_EDGE ( 'NONE', *, *, #5706, .F. ) ;
#26499=ORIENTED_EDGE ( 'NONE', *, *, #16917, .T. ) ;
#26500=CARTESIAN_POINT ( 'NONE',  ( 19.23646557533807666, 5.338914163118007039, 6.538284140784940128E-16 ) ) ;
#26503=VERTEX_POINT ( 'NONE', #15991 ) ;
#26504=DIRECTION ( 'NONE',  ( 0.000000000000000000, -1.000000000000000000, 0.000000000000000000 ) ) ;
#26510=CARTESIAN_POINT ( 'NONE',  ( 56.96931127949304141, 0.7396072067343685275, 1.750137474527811321 ) ) ;
#26513=CIRCLE ( 'NONE', #13858, 4.100000000000022737 ) ;
#26516=EDGE_CURVE ( 'NONE', #1141, #25117, #15836, .T. ) ;
#26523=CARTESIAN_POINT ( 'NONE',  ( 51.90000000000001279, 1.029992063861229212E-15, -4.375000000000002665 ) ) ;
#26525=DIRECTION ( 'NONE',  ( 1.000000000000000000, -0.000000000000000000, -0.000000000000000000 ) ) ;
#26535=CARTESIAN_POINT ( 'NONE',  ( 50.34896831693479413, 1.383117500627097263, 3.859810431918047957 ) ) ;
#26538=LINE ( 'NONE', #24015, #1538 ) ;
#26539=CARTESIAN_POINT ( 'NONE',  ( 57.00000000000001421, 0.7049799947465446026, 1.816196764953787124 ) ) ;
#26541=CARTESIAN_POINT ( 'NONE',  ( 56.95000000000001705, 0.6820512820512815155, -1.773360101234998210 ) ) ;
#26554=FACE_OUTER_BOUND ( 'NONE', #31159, .T. ) ;
#26555=CARTESIAN_POINT ( 'NONE',  ( 15.03925126672133139, -4.383220986679487119, -0.4611378927914498438 ) ) ;
#26558=CARTESIAN_POINT ( 'NONE',  ( 48.40000000000001990, 0.6304760106459518232, 3.950000000000022826 ) ) ;
#26559=ORIENTED_EDGE ( 'NONE', *, *, #6765, .F. ) ;
#26561=CARTESIAN_POINT ( 'NONE',  ( 15.74652664997117490, -0.2088129849845545005, -5.405094643512597941 ) ) ;
#26571=ORIENTED_EDGE ( 'NONE', *, *, #15081, .T. ) ;
#26576=DIRECTION ( 'NONE',  ( -1.000000000000000000, -2.586136946169074517E-16, 0.000000000000000000 ) ) ;
#26584=AXIS2_PLACEMENT_3D ( 'NONE', #4515, #23988, #19258 ) ;
#26587=CARTESIAN_POINT ( 'NONE',  ( 16.07512358269929109, -2.917650619476095386, 4.554978966839795973 ) ) ;
#26590=VERTEX_POINT ( 'NONE', #6655 ) ;
#26592=EDGE_CURVE ( 'NONE', #19631, #1993, #23142, .T. ) ;
#26599=VERTEX_POINT ( 'NONE', #13913 ) ;
#26600=CARTESIAN_POINT ( 'NONE',  ( -44.49999999999997868, -1.499999999999999556, -4.029888335921975262 ) ) ;
#26602=UNCERTAINTY_MEASURE_WITH_UNIT (LENGTH_MEASURE( 1.000000000000000082E-05 ), #7468, 'distance_accuracy_value', 'NONE');
#26606=VECTOR ( 'NONE', #11129, 1000.000000000000000 ) ;
#26608=ORIENTED_EDGE ( 'NONE', *, *, #21720, .F. ) ;
#26609=CARTESIAN_POINT ( 'NONE',  ( 58.45000000000001705, 0.000000000000000000, 0.000000000000000000 ) ) ;
#26610=AXIS2_PLACEMENT_3D ( 'NONE', #10665, #25379, #8132 ) ;
#26618=CARTESIAN_POINT ( 'NONE',  ( -36.04518387042616467, -5.340403875751214002, -0.9205822004571946326 ) ) ;
#26624=ORIENTED_EDGE ( 'NONE', *, *, #5008, .T. ) ;
#26633=CARTESIAN_POINT ( 'NONE',  ( 34.55000000000001847, 0.000000000000000000, 2.600000000000000089 ) ) ;
#26638=AXIS2_PLACEMENT_3D ( 'NONE', #5099, #21757, #28862 ) ;
#26639=CARTESIAN_POINT ( 'NONE',  ( 51.70000000000001705, -4.179189514726507682, 0.9999999999999997780 ) ) ;
#26640=CARTESIAN_POINT ( 'NONE',  ( -36.38012252111052902, -1.026563698233164956, -5.312790900508132630 ) ) ;
#26641=AXIS2_PLACEMENT_3D ( 'NONE', #1188, #6578, #23052 ) ;
#26642=ADVANCED_FACE ( 'NONE', ( #19186 ), #4593, .T. ) ;
#26645=CARTESIAN_POINT ( 'NONE',  ( 15.18459684427940104, -2.199885893005965265, 4.939696249117676352 ) ) ;
#26646=CARTESIAN_POINT ( 'NONE',  ( 15.67083574136752411, 5.009497273852853816, -2.047744636826899445 ) ) ;
#26653=CARTESIAN_POINT ( 'NONE',  ( 48.45869172792486523, -1.344780351710840982, -3.858600739747802599 ) ) ;
#26659=AXIS2_PLACEMENT_3D ( 'NONE', #26444, #2835, #4738 ) ;
#26669=DIRECTION ( 'NONE',  ( -0.000000000000000000, 0.000000000000000000, 1.000000000000000000 ) ) ;
#26670=CIRCLE ( 'NONE', #18080, 1.000000000000000000 ) ;
#26677=ADVANCED_FACE ( 'NONE', ( #16648 ), #20234, .F. ) ;
#26679=ORIENTED_EDGE ( 'NONE', *, *, #15556, .T. ) ;
#26681=EDGE_CURVE ( 'NONE', #18396, #3567, #7278, .T. ) ;
#26683=FACE_OUTER_BOUND ( 'NONE', #29280, .T. ) ;
#26685=CARTESIAN_POINT ( 'NONE',  ( 56.95000000000001705, 0.6820512820512819596, 1.773360101234998210 ) ) ;
#26690=EDGE_CURVE ( 'NONE', #7967, #2624, #726, .T. ) ;
#26692=CARTESIAN_POINT ( 'NONE',  ( 51.75288078123234925, -4.174487749534351977, 1.011178756798950307 ) ) ;
#26696=VECTOR ( 'NONE', #20541, 1000.000000000000000 ) ;
#26715=( BOUNDED_SURFACE ( )  B_SPLINE_SURFACE ( 3, 2, ( 
 ( #29445, #12212, #21891 ),
 ( #27067, #26618, #179 ),
 ( #5388, #26919, #5229 ),
 ( #2859, #15048, #14736 ),
 ( #481, #12348, #5086 ),
 ( #9834, #28993, #14588 ),
 ( #29597, #7466, #12511 ),
 ( #22197, #2706, #24397 ),
 ( #22035, #10146, #17136 ),
 ( #332, #19667, #3018 ),
 ( #12661, #633, #10294 ),
 ( #7921, #24091, #17594 ),
 ( #4759, #14418, #2402 ),
 ( #12066, #23128, #30068 ),
 ( #18067, #18227, #3328 ),
 ( #15825, #15683, #22962 ) ),
 .UNSPECIFIED., .F., .F., .T. ) 
 B_SPLINE_SURFACE_WITH_KNOTS ( ( 4, 2, 2, 2, 2, 2, 2, 4 ),
 ( 3, 3 ),
 ( 0.001780502285214257806, 0.002558945925323789783, 0.002753556835351172669, 0.002948167745378555554, 0.003337389565433321326, 0.003726611385488087097, 0.004115833205542852868, 0.004894276845652385279 ),
 ( 0.000000000000000000, 1.000000000000000000 ),
 .UNSPECIFIED. ) 
 GEOMETRIC_REPRESENTATION_ITEM ( )  RATIONAL_B_SPLINE_SURFACE ( (
 ( 1.000000000000000000, 0.9418517008537213853, 1.000000000000000000),
 ( 1.000000000000000000, 0.9417987965884944135, 1.000000000000000000),
 ( 1.000000000000000000, 0.9418198861734204952, 1.000000000000000000),
 ( 1.000000000000000000, 0.9434060303845512863, 1.000000000000000000),
 ( 1.000000000000000000, 0.9437939819948102382, 1.000000000000000000),
 ( 1.000000000000000000, 0.9445989566712813534, 1.000000000000000000),
 ( 1.000000000000000000, 0.9450169930049779898, 1.000000000000000000),
 ( 1.000000000000000000, 0.9461610507673671178, 1.000000000000000000),
 ( 1.000000000000000000, 0.9467217966427039499, 1.000000000000000000),
 ( 1.000000000000000000, 0.9467345476124477965, 1.000000000000000000),
 ( 1.000000000000000000, 0.9461964028052916031, 1.000000000000000000),
 ( 1.000000000000000000, 0.9446801822473822607, 1.000000000000000000),
 ( 1.000000000000000000, 0.9437582546537023331, 1.000000000000000000),
 ( 1.000000000000000000, 0.9418129560294634661, 1.000000000000000000),
 ( 1.000000000000000000, 0.9418016889778226819, 1.000000000000000000),
 ( 1.000000000000000000, 0.9418517008537213853, 1.000000000000000000) ) ) 
 REPRESENTATION_ITEM ( '' )  SURFACE ( )  );
#26719=CARTESIAN_POINT ( 'NONE',  ( 57.04073536323585358, 0.7493370604887438224, 1.778939771162194372 ) ) ;
#26722=EDGE_CURVE ( 'NONE', #9911, #21964, #21651, .T. ) ;
#26726=CARTESIAN_POINT ( 'NONE',  ( -35.85663232820581925, -3.426725943139554253, -3.937891353488750301 ) ) ;
#26728=CARTESIAN_POINT ( 'NONE',  ( 15.03925126672133139, -5.377732432866646484, -0.5657657256215582464 ) ) ;
#26732=CARTESIAN_POINT ( 'NONE',  ( 47.00000000000002132, -3.726179070414207928, 1.100000000000000533 ) ) ;
#26735=ORIENTED_EDGE ( 'NONE', *, *, #22066, .F. ) ;
#26736=CARTESIAN_POINT ( 'NONE',  ( -54.49608498031047787, 1.530604779201329091, 4.051096982736678953 ) ) ;
#26738=CARTESIAN_POINT ( 'NONE',  ( 15.39414421509791353, 0.2904410314644420565, -5.200000000384609855 ) ) ;
#26739=CARTESIAN_POINT ( 'NONE',  ( -35.85663232820579083, -4.861582140531640839, 2.394243978978324972 ) ) ;
#26742=VERTEX_POINT ( 'NONE', #17845 ) ;
#26744=DIRECTION ( 'NONE',  ( 0.000000000000000000, 0.000000000000000000, -1.000000000000000000 ) ) ;
#26746=CARTESIAN_POINT ( 'NONE',  ( -54.48478889579405404, -1.513794642953540270, -4.039462313877657529 ) ) ;
#26758=DIRECTION ( 'NONE',  ( -1.000000000000000000, -0.000000000000000000, -0.000000000000000000 ) ) ;
#26767=CIRCLE ( 'NONE', #7067, 5.338914163118009704 ) ;
#26771=CARTESIAN_POINT ( 'NONE',  ( 15.66436536804551594, -2.847679722116473133, -4.601476325142666468 ) ) ;
#26778=CARTESIAN_POINT ( 'NONE',  ( 56.95000053796676553, -0.7321038892619347038, -1.754109389045036771 ) ) ;
#26785=CIRCLE ( 'NONE', #23763, 10.00000000000000178 ) ;
#26790=CARTESIAN_POINT ( 'NONE',  ( 50.45717930666029361, 1.210123066480781606, 3.917958458743180827 ) ) ;
#26793=CIRCLE ( 'NONE', #1511, 1.000000000000000000 ) ;
#26794=CYLINDRICAL_SURFACE ( 'NONE', #26638, 0.05000000000000012768 ) ;
#26795=LINE ( 'NONE', #27086, #24050 ) ;
#26796=CARTESIAN_POINT ( 'NONE',  ( 46.99360240935735078, -4.235057606083818982, 1.098058400101960652 ) ) ;
#26804=CARTESIAN_POINT ( 'NONE',  ( -35.85663232820584057, -3.056483311920853208, -4.206888370749738648 ) ) ;
#26807=ORIENTED_EDGE ( 'NONE', *, *, #31098, .T. ) ;
#26808=VECTOR ( 'NONE', #9421, 1000.000000000000000 ) ;
#26809=CARTESIAN_POINT ( 'NONE',  ( 16.00221665700884088, -4.939398376933302082, 2.210903708596471340 ) ) ;
#26811=ORIENTED_EDGE ( 'NONE', *, *, #10229, .F. ) ;
#26814=AXIS2_PLACEMENT_3D ( 'NONE', #15128, #10222, #19891 ) ;
#26820=EDGE_CURVE ( 'NONE', #24297, #16594, #4913, .T. ) ;
#26824=EDGE_LOOP ( 'NONE', ( #9790, #4611, #28035, #3241 ) ) ;
#26826=CARTESIAN_POINT ( 'NONE',  ( 51.78977120336473661, -4.154252208774217969, -1.054526470899727508 ) ) ;
#26828=DIRECTION ( 'NONE',  ( 1.000000000000000000, 3.125586771759065906E-16, 0.000000000000000000 ) ) ;
#26832=CARTESIAN_POINT ( 'NONE',  ( -36.31440869660537629, -3.100731772197714342, 4.174739983989991465 ) ) ;
#26841=DIRECTION ( 'NONE',  ( 0.000000000000000000, 0.000000000000000000, -1.000000000000000000 ) ) ;
#26850=CARTESIAN_POINT ( 'NONE',  ( -44.49999999999999289, -1.499999999999999556, 4.029888335921975262 ) ) ;
#26851=EDGE_CURVE ( 'NONE', #25588, #24297, #13222, .T. ) ;
#26859=CARTESIAN_POINT ( 'NONE',  ( 36.55000000000001847, 2.265596578422603100E-16, 1.850000000000000089 ) ) ;
#26860=CARTESIAN_POINT ( 'NONE',  ( -35.85663232820579793, -4.018128179617549200, -3.618665901676661800 ) ) ;
#26864=VERTEX_POINT ( 'NONE', #8949 ) ;
#26865=EDGE_CURVE ( 'NONE', #24464, #473, #9123, .T. ) ;
#26866=CARTESIAN_POINT ( 'NONE',  ( 15.03925126672132784, 5.377732432866636714, 0.5657657256216092057 ) ) ;
#26867=CARTESIAN_POINT ( 'NONE',  ( -36.48821680285139735, -2.849134329833951096, -4.601168830303078217 ) ) ;
#26872=ADVANCED_FACE ( 'NONE', ( #21648 ), #26046, .F. ) ;
#26877=ORIENTED_EDGE ( 'NONE', *, *, #28613, .F. ) ;
#26881=CARTESIAN_POINT ( 'NONE',  ( -54.46439202372638277, -1.502116081466616793, -4.031358338852112588 ) ) ;
#26882=CARTESIAN_POINT ( 'NONE',  ( -35.85663232820584057, 3.275050215668857234, 2.949461045527371983 ) ) ;
#26885=CARTESIAN_POINT ( 'NONE',  ( 34.50000000000001421, 0.000000000000000000, -2.649999999999999911 ) ) ;
#26889=CARTESIAN_POINT ( 'NONE',  ( 51.70000000000001705, -4.179189514726508570, -0.9000000000000002442 ) ) ;
#26894=LINE ( 'NONE', #24375, #19081 ) ;
#26895=CARTESIAN_POINT ( 'NONE',  ( 15.03925126672132961, 1.123735532908305634, 5.289358697221540950 ) ) ;
#26907=CARTESIAN_POINT ( 'NONE',  ( 56.95000000000001705, 0.000000000000000000, 0.000000000000000000 ) ) ;
#26908=CARTESIAN_POINT ( 'NONE',  ( 57.00555950015162665, 0.7236022373656367801, -2.438089627148707805 ) ) ;
#26910=DIRECTION ( 'NONE',  ( 6.938893903907228378E-15, 1.734723475976807094E-15, 1.000000000000000000 ) ) ;
#26911=VERTEX_POINT ( 'NONE', #13833 ) ;
#26915=ORIENTED_EDGE ( 'NONE', *, *, #21435, .T. ) ;
#26918=AXIS2_PLACEMENT_3D ( 'NONE', #13306, #15716, #25363 ) ;
#26919=CARTESIAN_POINT ( 'NONE',  ( -36.22818246778668794, -5.326563020867394194, -0.9981196555229843170 ) ) ;
#26920=ORIENTED_EDGE ( 'NONE', *, *, #21672, .T. ) ;
#26923=DIRECTION ( 'NONE',  ( 0.000000000000000000, 0.000000000000000000, 1.000000000000000000 ) ) ;
#26928=CARTESIAN_POINT ( 'NONE',  ( 48.39103590182073589, -1.199904535326233646, -3.921111011342365504 ) ) ;
#26930=CARTESIAN_POINT ( 'NONE',  ( -54.47366401599046526, -1.505709097230404803, 3.303769268891089350 ) ) ;
#26932=FACE_OUTER_BOUND ( 'NONE', #27182, .T. ) ;
#26934=CARTESIAN_POINT ( 'NONE',  ( -36.22955757456079340, -0.2668145608218571163, -5.199999998579026617 ) ) ;
#26935=CIRCLE ( 'NONE', #2169, 2.600000000000000089 ) ;
#26939=CARTESIAN_POINT ( 'NONE',  ( 57.05000000000001847, -0.7500000000000000000, 2.421260002560650104 ) ) ;
#26941=ORIENTED_EDGE ( 'NONE', *, *, #708, .F. ) ;
#26942=DIRECTION ( 'NONE',  ( 0.000000000000000000, 0.000000000000000000, -1.000000000000000000 ) ) ;
#26944=CARTESIAN_POINT ( 'NONE',  ( 15.98305126557416855, 3.597789892641498621, -4.037455662930067746 ) ) ;
#26946=CARTESIAN_POINT ( 'NONE',  ( 57.00000000000001421, 0.7263660278559024297, 2.436986164851962844 ) ) ;
#26951=ORIENTED_EDGE ( 'NONE', *, *, #26283, .F. ) ;
#26955=CARTESIAN_POINT ( 'NONE',  ( 57.05000000000001847, -0.8000000000000002665, 2.421260002560650104 ) ) ;
#26959=CARTESIAN_POINT ( 'NONE',  ( -44.49999999999999289, 0.000000000000000000, 0.000000000000000000 ) ) ;
#26961=DIRECTION ( 'NONE',  ( 1.000000000000000000, 2.586136946169074517E-16, -0.000000000000000000 ) ) ;
#26965=FACE_OUTER_BOUND ( 'NONE', #17874, .T. ) ;
#26966=CARTESIAN_POINT ( 'NONE',  ( -54.45487361440510909, -1.499999999999999112, 4.029888335921975262 ) ) ;
#26970=CARTESIAN_POINT ( 'NONE',  ( 57.02007310689670305, 0.7405013978967619481, 2.427462356522636533 ) ) ;
#26971=APPLICATION_CONTEXT ( 'automotive_design' ) ;
#26972=CARTESIAN_POINT ( 'NONE',  ( -36.77443515226921278, -3.646557212684091276, 3.995389720703579339 ) ) ;
#26981=B_SPLINE_CURVE_WITH_KNOTS ( 'NONE', 3,
 ( #9047, #5183, #14832, #23454, #1923, #1744, #135, #24493, #18874, #11414 ),
 .UNSPECIFIED., .F., .F.,
 ( 4, 2, 2, 2, 4 ),
 ( 0.000000000000000000, 0.0004363777631660865864, 0.0006545666447491310181, 0.0007636610855406569202, 0.0008727555263321828223 ),
 .UNSPECIFIED. ) ;
#26982=VERTEX_POINT ( 'NONE', #23847 ) ;
#26991=ORIENTED_EDGE ( 'NONE', *, *, #14851, .F. ) ;
#26992=LINE ( 'NONE', #28917, #13023 ) ;
#26998=CARTESIAN_POINT ( 'NONE',  ( 15.61033468494299470, -4.977801270594324201, -2.126472881633288736 ) ) ;
#26999=CIRCLE ( 'NONE', #11846, 4.786668705877438867 ) ;
#27001=EDGE_CURVE ( 'NONE', #6668, #15602, #25303, .T. ) ;
#27003=DIRECTION ( 'NONE',  ( 1.000000000000000000, 0.000000000000000000, -0.000000000000000000 ) ) ;
#27004=CARTESIAN_POINT ( 'NONE',  ( 50.40671278470074412, 1.343285922954075007, -3.873819829599202791 ) ) ;
#27007=CARTESIAN_POINT ( 'NONE',  ( 15.90468948301723273, -4.892019442464182077, -2.306425897666045000 ) ) ;
#27011=VERTEX_POINT ( 'NONE', #7991 ) ;
#27012=EDGE_CURVE ( 'NONE', #5143, #24008, #13841, .T. ) ;
#27013=CARTESIAN_POINT ( 'NONE',  ( -37.18272003341173360, -24.59258869922088309, -3.011723503324820852E-15 ) ) ;
#27017=ORIENTED_EDGE ( 'NONE', *, *, #1351, .F. ) ;
#27018=CARTESIAN_POINT ( 'NONE',  ( 15.56274145962646926, 1.026563698233153632, -5.312790900508132630 ) ) ;
#27020=CARTESIAN_POINT ( 'NONE',  ( -36.11780688638071268, -5.377732434016947671, 0.5657657146878161125 ) ) ;
#27022=CARTESIAN_POINT ( 'NONE',  ( 58.45000000000001705, 0.8156862745098041323, -2.468735688885368873 ) ) ;
#27029=FACE_OUTER_BOUND ( 'NONE', #5028, .T. ) ;
#27031=FACE_OUTER_BOUND ( 'NONE', #8497, .T. ) ;
#27035=SPHERICAL_SURFACE ( 'NONE', #25490, 0.05000000000000000278 ) ;
#27036=CARTESIAN_POINT ( 'NONE',  ( 15.97944027357902108, -0.5584590966806823875, 5.380195666604553395 ) ) ;
#27041=CARTESIAN_POINT ( 'NONE',  ( 15.61033468494288101, -3.560621078037094378, 4.077054076718838793 ) ) ;
#27042=AXIS2_PLACEMENT_3D ( 'NONE', #9255, #21454, #68 ) ;
#27043=DIRECTION ( 'NONE',  ( 0.000000000000000000, 1.000000000000000000, -0.000000000000000000 ) ) ;
#27044=CIRCLE ( 'NONE', #11899, 4.349999999999997868 ) ;
#27056=CARTESIAN_POINT ( 'NONE',  ( -54.49999999999997868, 5.725223786013876262E-16, -4.650000000000000355 ) ) ;
#27057=CARTESIAN_POINT ( 'NONE',  ( 58.45000000000001705, 0.000000000000000000, 0.000000000000000000 ) ) ;
#27062=CIRCLE ( 'NONE', #27557, 4.000000000000022204 ) ;
#27063=CARTESIAN_POINT ( 'NONE',  ( 33.47623932017462778, 5.377732432866649148, -0.5657657256215208319 ) ) ;
#27066=CARTESIAN_POINT ( 'NONE',  ( -44.49999999999997868, 0.000000000000000000, 4.299999999999998046 ) ) ;
#27067=CARTESIAN_POINT ( 'NONE',  ( -36.11692583559979397, -5.377732435184391591, -0.5657657035909954280 ) ) ;
#27071=DIRECTION ( 'NONE',  ( 0.000000000000000000, 0.000000000000000000, -1.000000000000000000 ) ) ;
#27077=EDGE_CURVE ( 'NONE', #20165, #10936, #14973, .T. ) ;
#27080=CARTESIAN_POINT ( 'NONE',  ( 50.36545094904631270, 1.397701019745849704, 3.854421226863028682 ) ) ;
#27083=CARTESIAN_POINT ( 'NONE',  ( 51.80000000000001137, -4.144693941441892626, -1.074391609828098781 ) ) ;
#27086=CARTESIAN_POINT ( 'NONE',  ( -35.85663232820584057, 3.426725943139506292, 3.937891353488775170 ) ) ;
#27089=CARTESIAN_POINT ( 'NONE',  ( 48.47372026270296885, 1.373706569044511605, -3.853361913240786585 ) ) ;
#27090=CIRCLE ( 'NONE', #14956, 1.949999999999999956 ) ;
#27091=CARTESIAN_POINT ( 'NONE',  ( 54.49969840703174384, -0.002993017367578260958, -4.282759600741087525 ) ) ;
#27096=CARTESIAN_POINT ( 'NONE',  ( -54.49999999999997868, 1.549999999999999600, -3.332135201338624952 ) ) ;
#27106=ORIENTED_EDGE ( 'NONE', *, *, #6509, .T. ) ;
#27107=CARTESIAN_POINT ( 'NONE',  ( 16.08093158123429944, -5.226279933021935165, 1.394410282272784407 ) ) ;
#27111=CIRCLE ( 'NONE', #15988, 0.4576450603546999840 ) ;
#27112=CARTESIAN_POINT ( 'NONE',  ( 15.74652664997094220, 5.205077242910887136, 1.471673150993847212 ) ) ;
#27113=EDGE_LOOP ( 'NONE', ( #25081, #26915, #4144, #18644 ) ) ;
#27118=CIRCLE ( 'NONE', #2354, 0.1000000000000002554 ) ;
#27120=ORIENTED_EDGE ( 'NONE', *, *, #17120, .T. ) ;
#27128=CARTESIAN_POINT ( 'NONE',  ( 51.76135430833949158, -4.169908074913990070, -1.021033875312352457 ) ) ;
#27132=CARTESIAN_POINT ( 'NONE',  ( 57.00319509709754584, -0.7184317838911207232, 2.441240553461111684 ) ) ;
#27133=CARTESIAN_POINT ( 'NONE',  ( -35.98994760229914647, -3.426725948577701519, 3.937891352654260491 ) ) ;
#27138=CARTESIAN_POINT ( 'NONE',  ( 50.36545094904631270, -1.397701019745800854, -3.854421226863028238 ) ) ;
#27140=ADVANCED_FACE ( 'NONE', ( #29498 ), #5459, .T. ) ;
#27147=ORIENTED_EDGE ( 'NONE', *, *, #12813, .F. ) ;
#27148=ORIENTED_EDGE ( 'NONE', *, *, #11563, .F. ) ;
#27154=CARTESIAN_POINT ( 'NONE',  ( 16.10660252424455763, 5.231589534716049705, 1.397536681175259199 ) ) ;
#27163=LINE ( 'NONE', #21965, #10627 ) ;
#27165=EDGE_LOOP ( 'NONE', ( #9295, #30052, #19613, #9695 ) ) ;
#27169=CARTESIAN_POINT ( 'NONE',  ( 15.61552784268253546, -5.277544294472352071, -1.204650266290682170 ) ) ;
#27173=CIRCLE ( 'NONE', #24639, 0.09999999999999986677 ) ;
#27175=AXIS2_PLACEMENT_3D ( 'NONE', #14435, #5243, #14893 ) ;
#27179=DIRECTION ( 'NONE',  ( 1.000000000000000000, 0.000000000000000000, -0.000000000000000000 ) ) ;
#27182=EDGE_LOOP ( 'NONE', ( #35, #8339, #6869, #2890 ) ) ;
#27183=CIRCLE ( 'NONE', #21130, 1.000000000000000000 ) ;
#27184=CARTESIAN_POINT ( 'NONE',  ( -54.49999999999997868, 0.000000000000000000, 2.168404344971008868E-14 ) ) ;
#27185=CARTESIAN_POINT ( 'NONE',  ( -36.58361892165925155, -3.265074799938336270, -4.311675893544455462 ) ) ;
#27195=FACE_OUTER_BOUND ( 'NONE', #3189, .T. ) ;
#27196=ADVANCED_FACE ( 'NONE', ( #8449 ), #12871, .T. ) ;
#27199=CARTESIAN_POINT ( 'NONE',  ( 57.05000000000001847, -0.7500000000000000000, -1.778341924377873751 ) ) ;
#27201=LINE ( 'NONE', #5510, #12060 ) ;
#27214=CARTESIAN_POINT ( 'NONE',  ( 15.29449157529454695, -2.734387802834054693, 4.440904455451909705 ) ) ;
#27218=CARTESIAN_POINT ( 'NONE',  ( -36.63359589171280106, 4.847650360853540619, -2.396424556482824375 ) ) ;
#27227=DIRECTION ( 'NONE',  ( 0.000000000000000000, -1.000000000000000000, 0.000000000000000000 ) ) ;
#27234=ORIENTED_EDGE ( 'NONE', *, *, #6121, .T. ) ;
#27238=CARTESIAN_POINT ( 'NONE',  ( 50.34137136386934230, 1.344608935533184946, 3.858631320448700386 ) ) ;
#27241=DIRECTION ( 'NONE',  ( -1.000000000000000000, -0.000000000000000000, -0.000000000000000000 ) ) ;
#27242=EDGE_CURVE ( 'NONE', #24297, #26503, #838, .T. ) ;
#27247=CARTESIAN_POINT ( 'NONE',  ( 48.29999997257028355, -0.7904052113206601060, -4.025738854575411807 ) ) ;
#27248=CARTESIAN_POINT ( 'NONE',  ( 15.74652664997094575, 0.2088129849845392905, 5.405094643512426522 ) ) ;
#27254=CARTESIAN_POINT ( 'NONE',  ( 58.50000000000001421, 0.8000000000000000444, -2.421260002560649660 ) ) ;
#27256=CARTESIAN_POINT ( 'NONE',  ( 15.18463186935387377, -4.018128179617967533, 3.618665901676295427 ) ) ;
#27258=DIRECTION ( 'NONE',  ( 0.000000000000000000, -2.168404344971008128E-16, -1.000000000000000000 ) ) ;
#27260=CARTESIAN_POINT ( 'NONE',  ( 50.40000000000001279, -0.7707709757764150682, -3.938803467580344719 ) ) ;
#27263=CARTESIAN_POINT ( 'NONE',  ( 15.44259799936806132, 3.232943006030417621, -4.078682900256741739 ) ) ;
#27266=EDGE_CURVE ( 'NONE', #16594, #16545, #29134, .T. ) ;
#27267=ORIENTED_EDGE ( 'NONE', *, *, #25179, .T. ) ;
#27268=FACE_OUTER_BOUND ( 'NONE', #5590, .T. ) ;
#27269=LINE ( 'NONE', #5586, #26490 ) ;
#27272=EDGE_CURVE ( 'NONE', #10142, #20943, #9927, .T. ) ;
#27287=VECTOR ( 'NONE', #1680, 1000.000000000000000 ) ;
#27291=DIRECTION ( 'NONE',  ( 1.000000000000000000, 0.000000000000000000, 0.000000000000000000 ) ) ;
#27294=DIRECTION ( 'NONE',  ( 1.000000000000000000, 0.000000000000000000, -4.738179285253040686E-16 ) ) ;
#27296=DIRECTION ( 'NONE',  ( 1.000000000000000000, -0.000000000000000000, -0.000000000000000000 ) ) ;
#27300=CARTESIAN_POINT ( 'NONE',  ( 48.43454905095371998, -1.397701019745800854, 3.854421226863028238 ) ) ;
#27307=ORIENTED_EDGE ( 'NONE', *, *, #12120, .T. ) ;
#27311=CARTESIAN_POINT ( 'NONE',  ( -35.85663232820584057, -4.804073783693461941, 2.042134687550347216 ) ) ;
#27314=ORIENTED_EDGE ( 'NONE', *, *, #476, .T. ) ;
#27322=EDGE_CURVE ( 'NONE', #12623, #5273, #8288, .T. ) ;
#27326=CARTESIAN_POINT ( 'NONE',  ( 51.80690729991166421, -4.271967808728815541, -0.9446991603439683916 ) ) ;
#27335=EDGE_LOOP ( 'NONE', ( #11728, #7042, #9532, #27147 ) ) ;
#27337=CARTESIAN_POINT ( 'NONE',  ( -36.31440869660545445, -3.012234853004159163, -4.239036759381638930 ) ) ;
#27340=EDGE_CURVE ( 'NONE', #7731, #8913, #27118, .T. ) ;
#27345=CARTESIAN_POINT ( 'NONE',  ( -36.43290890416664496, -5.277544294472357400, 1.204650266290678395 ) ) ;
#27347=CARTESIAN_POINT ( 'NONE',  ( 48.30000000000001847, -0.6462379109120514054, -4.048750000000023164 ) ) ;
#27350=DIRECTION ( 'NONE',  ( 0.000000000000000000, 0.000000000000000000, -1.000000000000000000 ) ) ;
#27352=CARTESIAN_POINT ( 'NONE',  ( 57.00381193298470350, -0.7199075706197948232, -1.804244861858284255 ) ) ;
#27355=DIRECTION ( 'NONE',  ( 0.000000000000000000, 1.000000000000000000, 0.000000000000000000 ) ) ;
#27361=ADVANCED_FACE ( 'NONE', ( #21293 ), #4630, .F. ) ;
#27367=CARTESIAN_POINT ( 'NONE',  ( 15.56274145962601629, 2.292272662152952112, 4.901537128432109647 ) ) ;
#27369=( BOUNDED_SURFACE ( )  B_SPLINE_SURFACE ( 3, 2, ( 
 ( #11084, #26282, #25806 ),
 ( #23603, #16313, #30721 ),
 ( #3957, #11568, #4262 ),
 ( #9343, #11392, #13907 ),
 ( #9026, #26119, #18378 ),
 ( #28663, #6979, #23136 ),
 ( #20765, #30874, #2054 ),
 ( #11717, #28185, #28014 ),
 ( #16644, #9193, #11232 ),
 ( #6801, #19012, #1904 ),
 ( #1721, #6650, #21244 ),
 ( #20908, #23437, #18855 ),
 ( #15985, #28497, #1424 ),
 ( #25647, #16463, #25957 ),
 ( #4435, #4588, #30540 ),
 ( #21077, #30390, #14083 ) ),
 .UNSPECIFIED., .F., .F., .T. ) 
 B_SPLINE_SURFACE_WITH_KNOTS ( ( 4, 2, 2, 2, 2, 2, 2, 4 ),
 ( 3, 3 ),
 ( 0.001780502285214230051, 0.002558945925323756823, 0.002753556835351138841, 0.002948167745378520426, 0.003337389565433284029, 0.003726611385488047632, 0.004115833205542811235, 0.004894276845652338441 ),
 ( 0.000000000000000000, 1.000000000000000000 ),
 .UNSPECIFIED. ) 
 GEOMETRIC_REPRESENTATION_ITEM ( )  RATIONAL_B_SPLINE_SURFACE ( (
 ( 1.000000000000000000, 0.9418517008537241608, 1.000000000000000000),
 ( 1.000000000000000000, 0.9417987965885392665, 1.000000000000000000),
 ( 1.000000000000000000, 0.9418198861733664273, 1.000000000000000000),
 ( 1.000000000000000000, 0.9434060303845691609, 1.000000000000000000),
 ( 1.000000000000000000, 0.9437939819947983588, 1.000000000000000000),
 ( 1.000000000000000000, 0.9445989566712983398, 1.000000000000000000),
 ( 1.000000000000000000, 0.9450169930049727718, 1.000000000000000000),
 ( 1.000000000000000000, 0.9461610507673836601, 1.000000000000000000),
 ( 1.000000000000000000, 0.9467217966425610642, 1.000000000000000000),
 ( 1.000000000000000000, 0.9467345476125937909, 1.000000000000000000),
 ( 1.000000000000000000, 0.9461964028053096998, 1.000000000000000000),
 ( 1.000000000000000000, 0.9446801822473712695, 1.000000000000000000),
 ( 1.000000000000000000, 0.9437582546537136574, 1.000000000000000000),
 ( 1.000000000000000000, 0.9418129560294529190, 1.000000000000000000),
 ( 1.000000000000000000, 0.9418016889778366707, 1.000000000000000000),
 ( 1.000000000000000000, 0.9418517008537241608, 1.000000000000000000) ) ) 
 REPRESENTATION_ITEM ( '' )  SURFACE ( )  );
#27372=CARTESIAN_POINT ( 'NONE',  ( 33.47623932017462778, 2.199885893005997239, -4.939696249117661253 ) ) ;
#27373=CARTESIAN_POINT ( 'NONE',  ( 48.45103168306561514, 1.383117500626982910, -3.859810431918025309 ) ) ;
#27375=EDGE_CURVE ( 'NONE', #8120, #13995, #6695, .T. ) ;
#27378=EDGE_CURVE ( 'NONE', #9785, #4498, #30136, .T. ) ;
#27380=CARTESIAN_POINT ( 'NONE',  ( 16.10705563471231017, -3.305069970238163179, -4.282766538619540597 ) ) ;
#27382=EDGE_CURVE ( 'NONE', #11505, #17419, #16281, .T. ) ;
#27383=EDGE_LOOP ( 'NONE', ( #22456, #15432, #15715, #2298 ) ) ;
#27386=CIRCLE ( 'NONE', #13223, 0.05000000000000143219 ) ;
#27390=CARTESIAN_POINT ( 'NONE',  ( 51.75086608074121841, -4.173104349845818462, 1.013903299540405145 ) ) ;
#27393=ADVANCED_FACE ( 'NONE', ( #28237 ), #29864, .T. ) ;
#27396=ORIENTED_EDGE ( 'NONE', *, *, #24412, .T. ) ;
#27401=CARTESIAN_POINT ( 'NONE',  ( 15.57907767661755827, -0.5233326973447697261, 5.388419908789401802 ) ) ;
#27411=EDGE_LOOP ( 'NONE', ( #18333, #4022, #6098, #21620 ) ) ;
#27413=CARTESIAN_POINT ( 'NONE',  ( 58.50000000000001421, 0.8000000000000000444, 1.778341924377873751 ) ) ;
#27416=CARTESIAN_POINT ( 'NONE',  ( 15.03925126672132606, 2.525801270006352350, -4.794550352686297146 ) ) ;
#27418=DIRECTION ( 'NONE',  ( 0.000000000000000000, 1.000000000000000000, 1.532429380227459806E-15 ) ) ;
#27424=CARTESIAN_POINT ( 'NONE',  ( 15.59140265158956318, -5.360483378448148706, 0.7132926830812496011 ) ) ;
#27427=CARTESIAN_POINT ( 'NONE',  ( 15.90468948301722740, 5.313409993919706586, -1.009519134730147316 ) ) ;
#27431=DIRECTION ( 'NONE',  ( 0.000000000000000000, 0.000000000000000000, -1.000000000000000000 ) ) ;
#27434=DIRECTION ( 'NONE',  ( -2.459562394685754633E-16, 0.9510565162951565288, -0.3090169943749382919 ) ) ;
#27439=FACE_OUTER_BOUND ( 'NONE', #9092, .T. ) ;
#27442=DIRECTION ( 'NONE',  ( 2.586136946169074517E-16, -1.000000000000000000, 0.000000000000000000 ) ) ;
#27445=EDGE_CURVE ( 'NONE', #10332, #4498, #20046, .T. ) ;
#27447=DIRECTION ( 'NONE',  ( 1.000000000000000000, -0.000000000000000000, -0.000000000000000000 ) ) ;
#27452=ORIENTED_EDGE ( 'NONE', *, *, #28610, .T. ) ;
#27453=CARTESIAN_POINT ( 'NONE',  ( -54.44999999999997442, 1.499999999999998890, 3.300094695611021756 ) ) ;
#27463=VERTEX_POINT ( 'NONE', #13151 ) ;
#27469=CARTESIAN_POINT ( 'NONE',  ( 15.48686146417452747, -4.979756346315167725, -1.501439362221205442 ) ) ;
#27472=ADVANCED_FACE ( 'NONE', ( #7947 ), #28137, .T. ) ;
#27473=CARTESIAN_POINT ( 'NONE',  ( 51.70000000000001705, -4.276948333784438283, -0.9210526315789475671 ) ) ;
#27476=EDGE_CURVE ( 'NONE', #29070, #5429, #15840, .T. ) ;
#27485=CARTESIAN_POINT ( 'NONE',  ( 15.03925126672132961, 2.686240680702102424, 4.475885388010754085 ) ) ;
#27491=CARTESIAN_POINT ( 'NONE',  ( 15.41170998834775041, -0.6969927240735035445, -5.374332520738491326 ) ) ;
#27492=CARTESIAN_POINT ( 'NONE',  ( -37.18272003341174781, 24.59258869922085111, 0.000000000000000000 ) ) ;
#27494=DIRECTION ( 'NONE',  ( 1.000000000000000000, 5.172273892338151992E-16, 0.000000000000000000 ) ) ;
#27498=CARTESIAN_POINT ( 'NONE',  ( 57.03643325641707662, -0.7481242503215885797, -1.780024810282529790 ) ) ;
#27503=TOROIDAL_SURFACE ( 'NONE', #10302, 4.349999999999997868, 0.05000000000000000278 ) ;
#27510=CARTESIAN_POINT ( 'NONE',  ( 15.68751737981905947, 2.884962146574134856, 4.577321775072962673 ) ) ;
#27511=AXIS2_PLACEMENT_3D ( 'NONE', #25599, #11048, #9149 ) ;
#27523=CARTESIAN_POINT ( 'NONE',  ( 50.46977479615470230, -1.142230555601075004, 3.938343097974785767 ) ) ;
#27525=CARTESIAN_POINT ( 'NONE',  ( 47.00000000000002132, -4.131056160354152240, 1.099999999999999867 ) ) ;
#27535=CIRCLE ( 'NONE', #14386, 4.275000000000000355 ) ;
#27536=EDGE_CURVE ( 'NONE', #13205, #26264, #1350, .T. ) ;
#27540=VECTOR ( 'NONE', #14503, 1000.000000000000000 ) ;
#27542=EDGE_CURVE ( 'NONE', #20590, #12071, #17769, .T. ) ;
#27546=CARTESIAN_POINT ( 'NONE',  ( 48.40000000000002700, -0.7711297561635785947, -3.938774833552663335 ) ) ;
#27547=CARTESIAN_POINT ( 'NONE',  ( 16.10705563471230661, 0.1565107631088668017, 5.407502298984289801 ) ) ;
#27555=DIRECTION ( 'NONE',  ( 1.000000000000000000, 0.000000000000000000, 0.000000000000000000 ) ) ;
#27557=AXIS2_PLACEMENT_3D ( 'NONE', #6546, #2100, #11764 ) ;
#27560=DIRECTION ( 'NONE',  ( -1.000000000000000000, -0.000000000000000000, -0.000000000000000000 ) ) ;
#27562=CARTESIAN_POINT ( 'NONE',  ( 15.81621483022862762, 3.777141534544376178, -3.869853550719620117 ) ) ;
#27564=DIRECTION ( 'NONE',  ( 1.000000000000000000, -0.000000000000000000, -0.000000000000000000 ) ) ;
#27569=ORIENTED_EDGE ( 'NONE', *, *, #813, .T. ) ;
#27571=DIRECTION ( 'NONE',  ( -1.000000000000000000, -0.000000000000000000, -0.000000000000000000 ) ) ;
#27580=DIRECTION ( 'NONE',  ( 4.117859380279907901E-15, -0.9495137264943731559, -0.3137254901960768172 ) ) ;
#27582=DIRECTION ( 'NONE',  ( 1.000000000000000000, 9.742518634745315608E-17, -4.338815227902241051E-17 ) ) ;
#27583=CIRCLE ( 'NONE', #13916, 4.100000000000022737 ) ;
#27584=AXIS2_PLACEMENT_3D ( 'NONE', #19187, #28827, #19480 ) ;
#27587=B_SPLINE_CURVE_WITH_KNOTS ( 'NONE', 3,
 ( #16992, #29322, #19372, #27089, #21912, #7322, #5412, #2723, #7634, #19979, #15223, #192, #29618, #24870 ),
 .UNSPECIFIED., .F., .F.,
 ( 4, 2, 2, 2, 2, 2, 4 ),
 ( 0.000000000000000000, 2.506106230924540920E-05, 5.012212461849081840E-05, 0.0001002442492369731529, 0.0002004884984739371985, 0.0004009769969478685966, 0.0008019539938957305795 ),
 .UNSPECIFIED. ) ;
#27588=AXIS2_PLACEMENT_3D ( 'NONE', #29164, #2717, #19368 ) ;
#27591=FACE_OUTER_BOUND ( 'NONE', #21526, .T. ) ;
#27600=B_SPLINE_CURVE_WITH_KNOTS ( 'NONE', 3,
 ( #21396, #6980, #16645, #15620, #17988, #25264, #10552, #20381, #20229, #15907, #1049, #29701, #5967, #8318 ),
 .UNSPECIFIED., .F., .F.,
 ( 4, 2, 2, 2, 2, 2, 4 ),
 ( 0.000000000000000000, 0.0003953907277084696219, 0.0005930860915627040805, 0.0006919337734898216080, 0.0007413576144533806428, 0.0007660695349351558233, 0.0007907814554169310039 ),
 .UNSPECIFIED. ) ;
#27607=VERTEX_POINT ( 'NONE', #29940 ) ;
#27608=DIRECTION ( 'NONE',  ( 1.000000000000000000, -0.000000000000000000, -0.000000000000000000 ) ) ;
#27617=CARTESIAN_POINT ( 'NONE',  ( 57.05000000000001847, 0.8000000000000000444, 2.421260002560649660 ) ) ;
#27619=EDGE_CURVE ( 'NONE', #16975, #26152, #3376, .T. ) ;
#27622=ORIENTED_EDGE ( 'NONE', *, *, #2418, .F. ) ;
#27623=AXIS2_PLACEMENT_3D ( 'NONE', #16517, #4308, #21292 ) ;
#27628=EDGE_CURVE ( 'NONE', #29888, #6920, #11401, .T. ) ;
#27631=CARTESIAN_POINT ( 'NONE',  ( 46.99423841112505329, -4.272136569073790469, -0.9439330974869863944 ) ) ;
#27650=CARTESIAN_POINT ( 'NONE',  ( 56.95000000000001705, -0.6820512820512819596, 1.773360101234998210 ) ) ;
#27652=ORIENTED_EDGE ( 'NONE', *, *, #13678, .F. ) ;
#27657=CARTESIAN_POINT ( 'NONE',  ( 15.22842924604238135, -0.7747498452696431892, -5.363501451415723764 ) ) ;
#27660=DIRECTION ( 'NONE',  ( -1.000000000000000000, 0.000000000000000000, 0.000000000000000000 ) ) ;
#27673=DIRECTION ( 'NONE',  ( -1.000000000000000000, -0.000000000000000000, -0.000000000000000000 ) ) ;
#27675=CARTESIAN_POINT ( 'NONE',  ( -36.43290890416757577, 5.277544294472448883, -1.204650266290766103 ) ) ;
#27678=CARTESIAN_POINT ( 'NONE',  ( -35.85663232820584057, -2.686240680702168593, 4.475885388010719446 ) ) ;
#27679=DIRECTION ( 'NONE',  ( 1.000000000000000000, 0.000000000000000000, 0.000000000000000000 ) ) ;
#27681=TOROIDAL_SURFACE ( 'NONE', #4421, 2.549999999999999822, 0.05000000000000000278 ) ;
#27684=CARTESIAN_POINT ( 'NONE',  ( 15.81621483022873775, 2.513248512186213812, 4.788125582312069639 ) ) ;
#27685=VECTOR ( 'NONE', #749, 1000.000000000000000 ) ;
#27688=AXIS2_PLACEMENT_3D ( 'NONE', #9157, #21509, #24025 ) ;
#27705=ORIENTED_EDGE ( 'NONE', *, *, #20198, .T. ) ;
#27711=LINE ( 'NONE', #10913, #4651 ) ;
#27718=EDGE_CURVE ( 'NONE', #19839, #24615, #6810, .T. ) ;
#27722=CARTESIAN_POINT ( 'NONE',  ( 15.44259799936806665, -0.2181161761757533513, 5.200000001420971962 ) ) ;
#27732=ORIENTED_EDGE ( 'NONE', *, *, #23755, .F. ) ;
#27733=CARTESIAN_POINT ( 'NONE',  ( 50.34896831693479413, -1.383117500627048635, -3.859810431918047957 ) ) ;
#27740=DIRECTION ( 'NONE',  ( 1.000000000000000000, 0.000000000000000000, 0.000000000000000000 ) ) ;
#27742=ORIENTED_EDGE ( 'NONE', *, *, #29746, .T. ) ;
#27746=VERTEX_POINT ( 'NONE', #4443 ) ;
#27748=FACE_OUTER_BOUND ( 'NONE', #28435, .T. ) ;
#27751=DIRECTION ( 'NONE',  ( 1.000000000000000000, 0.000000000000000000, 4.738179285253022937E-16 ) ) ;
#27755=CIRCLE ( 'NONE', #29762, 0.05000000000000017625 ) ;
#27756=EDGE_CURVE ( 'NONE', #12845, #10038, #5399, .T. ) ;
#27758=CARTESIAN_POINT ( 'NONE',  ( 36.50000000000002132, 0.8000000000000000444, -1.778341924377873751 ) ) ;
#27759=DIRECTION ( 'NONE',  ( 0.000000000000000000, 0.000000000000000000, 1.000000000000000000 ) ) ;
#27760=FACE_OUTER_BOUND ( 'NONE', #28558, .T. ) ;
#27764=CIRCLE ( 'NONE', #14108, 1.000000000000000000 ) ;
#27765=DIRECTION ( 'NONE',  ( 1.000000000000000000, 0.000000000000000000, 0.000000000000000000 ) ) ;
#27768=CARTESIAN_POINT ( 'NONE',  ( -54.49454330418567594, 1.526701536696945638, -3.317245250669464518 ) ) ;
#27769=DIRECTION ( 'NONE',  ( 1.000000000000000000, 0.000000000000000000, -0.000000000000000000 ) ) ;
#27775=AXIS2_PLACEMENT_3D ( 'NONE', #16172, #13765, #23451 ) ;
#27776=ADVANCED_FACE ( 'NONE', ( #28507 ), #1581, .T. ) ;
#27778=DIRECTION ( 'NONE',  ( 1.000000000000000000, 0.000000000000000000, 0.000000000000000000 ) ) ;
#27787=EDGE_LOOP ( 'NONE', ( #6550, #18436, #4993, #6704 ) ) ;
#27788=CARTESIAN_POINT ( 'NONE',  ( 36.55000000000001847, 0.000000000000000000, -1.850000000000000089 ) ) ;
#27793=ORIENTED_EDGE ( 'NONE', *, *, #9024, .F. ) ;
#27796=CARTESIAN_POINT ( 'NONE',  ( 47.04662468001162523, -4.276948325786881888, -0.9210526687159725778 ) ) ;
#27803=DIRECTION ( 'NONE',  ( -1.000000000000000000, -0.000000000000000000, -0.000000000000000000 ) ) ;
#27815=EDGE_LOOP ( 'NONE', ( #16866, #7851, #1549 ) ) ;
#27831=CARTESIAN_POINT ( 'NONE',  ( -35.85663232820584057, -1.793057972834796621, -4.026191436120394762 ) ) ;
#27832=DIRECTION ( 'NONE',  ( 0.000000000000000000, 0.000000000000000000, 1.000000000000000000 ) ) ;
#27834=CARTESIAN_POINT ( 'NONE',  ( -36.89017861347081606, 5.034707333629178549, -1.977875755500439148 ) ) ;
#27837=CARTESIAN_POINT ( 'NONE',  ( -36.52679053911622020, -3.858136107555833583, 3.790289750283442505 ) ) ;
#27838=CARTESIAN_POINT ( 'NONE',  ( 56.99229849798533820, 0.7794861535680733811, 1.732743875013533108 ) ) ;
#27841=( BOUNDED_SURFACE ( )  B_SPLINE_SURFACE ( 3, 2, ( 
 ( #18785, #25889, #11649 ),
 ( #23993, #16564, #4192 ),
 ( #14320, #30961, #9276 ),
 ( #26211, #13829, #6732 ),
 ( #9602, #19262, #6426 ),
 ( #16086, #25738, #4046 ),
 ( #13689, #23370, #1650 ),
 ( #28428, #11309, #29494 ),
 ( #7667, #15102, #17326 ),
 ( #22397, #17485, #26832 ),
 ( #9891, #5134, #19406 ),
 ( #26972, #687, #29212 ),
 ( #21797, #21945, #12563 ),
 ( #12406, #3072, #7809 ),
 ( #17035, #7525, #27133 ),
 ( #14934, #12118, #5280 ) ),
 .UNSPECIFIED., .F., .F., .T. ) 
 B_SPLINE_SURFACE_WITH_KNOTS ( ( 4, 2, 2, 2, 2, 2, 2, 4 ),
 ( 3, 3 ),
 ( 0.001780502285214260842, 0.002558945925323795421, 0.002753556835351178740, 0.002948167745378562493, 0.003337389565433329999, 0.003726611385488097505, 0.004115833205542865011, 0.004894276845652399156 ),
 ( 0.000000000000000000, 1.000000000000000000 ),
 .UNSPECIFIED. ) 
 GEOMETRIC_REPRESENTATION_ITEM ( )  RATIONAL_B_SPLINE_SURFACE ( (
 ( 1.000000000000000000, 0.9418517008537223845, 1.000000000000000000),
 ( 1.000000000000000000, 0.9417987965885066259, 1.000000000000000000),
 ( 1.000000000000000000, 0.9418198861734071725, 1.000000000000000000),
 ( 1.000000000000000000, 0.9434060303845559492, 1.000000000000000000),
 ( 1.000000000000000000, 0.9437939819948627518, 1.000000000000000000),
 ( 1.000000000000000000, 0.9445989566712328367, 1.000000000000000000),
 ( 1.000000000000000000, 0.9450169930049197031, 1.000000000000000000),
 ( 1.000000000000000000, 0.9461610507674824699, 1.000000000000000000),
 ( 1.000000000000000000, 0.9467217966428496112, 1.000000000000000000),
 ( 1.000000000000000000, 0.9467345476123045778, 1.000000000000000000),
 ( 1.000000000000000000, 0.9461964028052702869, 1.000000000000000000),
 ( 1.000000000000000000, 0.9446801822474044652, 1.000000000000000000),
 ( 1.000000000000000000, 0.9437582546536025241, 1.000000000000000000),
 ( 1.000000000000000000, 0.9418129560296703007, 1.000000000000000000),
 ( 1.000000000000000000, 0.9418016889776684719, 1.000000000000000000),
 ( 1.000000000000000000, 0.9418517008537214963, 1.000000000000000000) ) ) 
 REPRESENTATION_ITEM ( '' )  SURFACE ( )  );
#27842=CARTESIAN_POINT ( 'NONE',  ( 15.41586008885044912, 3.272294129011773745, 4.050092634494075305 ) ) ;
#27845=CARTESIAN_POINT ( 'NONE',  ( 51.75429853018303561, -4.276948333784438283, 0.9210526315789470120 ) ) ;
#27847=B_SPLINE_CURVE_WITH_KNOTS ( 'NONE', 3,
 ( #9794, #3133, #17241, #26881, #10411, #12774, #22455, #19462, #26746, #14839, #7424, #20095, #4883, #14548, #24212, #24500, #2525, #5045, #12174 ),
 .UNSPECIFIED., .F., .F.,
 ( 4, 3, 3, 3, 3, 3, 4 ),
 ( 0.000000000000000000, 1.462084321540209121E-05, 2.917085440492037316E-05, 4.467649728434973632E-05, 6.285390091960512901E-05, 8.531547445983615763E-05, 8.677858956768834506E-05 ),
 .UNSPECIFIED. ) ;
#27854=ORIENTED_EDGE ( 'NONE', *, *, #19717, .F. ) ;
#27856=CARTESIAN_POINT ( 'NONE',  ( 57.00000000000001421, 0.6999999999999999556, -2.452039967047845437 ) ) ;
#27859=ORIENTED_EDGE ( 'NONE', *, *, #22069, .T. ) ;
#27864=LINE ( 'NONE', #20757, #2588 ) ;
#27866=ORIENTED_EDGE ( 'NONE', *, *, #3366, .T. ) ;
#27870=CARTESIAN_POINT ( 'NONE',  ( 15.29449157529479031, 0.3981319440499709872, 5.199999999410283458 ) ) ;
#27878=CARTESIAN_POINT ( 'NONE',  ( 58.50000000000001421, -0.8000000000000000444, -1.745709025009608784 ) ) ;
#27881=AXIS2_PLACEMENT_3D ( 'NONE', #20730, #3610, #30358 ) ;
#27883=DIRECTION ( 'NONE',  ( 1.000000000000000000, 0.000000000000000000, 0.000000000000000000 ) ) ;
#27886=DIRECTION ( 'NONE',  ( 0.000000000000000000, 0.000000000000000000, 1.000000000000000000 ) ) ;
#27892=EDGE_LOOP ( 'NONE', ( #11842, #19257, #22624, #17319 ) ) ;
#27894=CARTESIAN_POINT ( 'NONE',  ( 47.00000000000002132, -3.726179070414207928, -1.100000000000000089 ) ) ;
#27898=ORIENTED_EDGE ( 'NONE', *, *, #8648, .T. ) ;
#27902=CARTESIAN_POINT ( 'NONE',  ( 56.95000000000001705, 0.6820512820512819596, -1.773360101234998210 ) ) ;
#27903=EDGE_LOOP ( 'NONE', ( #20755, #6681, #18838, #12431 ) ) ;
#27905=AXIS2_PLACEMENT_3D ( 'NONE', #11225, #20900, #30530 ) ;
#27911=LINE ( 'NONE', #18421, #5442 ) ;
#27913=CARTESIAN_POINT ( 'NONE',  ( 15.03925126672132784, 3.817150320980686296, -2.203324261490496205 ) ) ;
#27916=DIRECTION ( 'NONE',  ( 0.000000000000000000, 0.000000000000000000, -1.000000000000000000 ) ) ;
#27922=CARTESIAN_POINT ( 'NONE',  ( -36.89831264271882105, -0.2888463313200454463, -5.401384060636567064 ) ) ;
#27925=FACE_OUTER_BOUND ( 'NONE', #1100, .T. ) ;
#27936=AXIS2_PLACEMENT_3D ( 'NONE', #5194, #7121, #12028 ) ;
#27940=CARTESIAN_POINT ( 'NONE',  ( 47.10000000000002274, -4.276948333784442724, -0.9210526315789473450 ) ) ;
#27944=CARTESIAN_POINT ( 'NONE',  ( 15.70940947763170215, 3.858136107555762528, 3.790289750283494019 ) ) ;
#27945=EDGE_CURVE ( 'NONE', #13205, #11230, #8943, .T. ) ;
#27954=VERTEX_POINT ( 'NONE', #2385 ) ;
#27956=VERTEX_POINT ( 'NONE', #7447 ) ;
#27971=FACE_OUTER_BOUND ( 'NONE', #24697, .T. ) ;
#27973=ORIENTED_EDGE ( 'NONE', *, *, #22207, .F. ) ;
#27974=CARTESIAN_POINT ( 'NONE',  ( -35.85663232820592583, 5.086913985776147840, -1.171642053949061291 ) ) ;
#27989=CARTESIAN_POINT ( 'NONE',  ( 56.95000000000001705, -0.6999999999999999556, 1.820027472320129736 ) ) ;
#27990=ORIENTED_EDGE ( 'NONE', *, *, #17811, .T. ) ;
#27994=CARTESIAN_POINT ( 'NONE',  ( 46.90000000000001279, -4.227689052994015206, -1.125730994152046804 ) ) ;
#27996=CARTESIAN_POINT ( 'NONE',  ( 48.37881665787880081, 1.311095223031216284, 3.884869838566831657 ) ) ;
#27997=CARTESIAN_POINT ( 'NONE',  ( 15.03925126672133139, -4.945493884734786683, -1.606888370749751882 ) ) ;
#28006=ADVANCED_FACE ( 'NONE', ( #6012 ), #15893, .T. ) ;
#28014=CARTESIAN_POINT ( 'NONE',  ( -36.30347965937281174, 2.964363692626830638, -4.273817190665726962 ) ) ;
#28015=EDGE_CURVE ( 'NONE', #12844, #12135, #18669, .T. ) ;
#28017=CIRCLE ( 'NONE', #2255, 0.04999999999999991257 ) ;
#28022=AXIS2_PLACEMENT_3D ( 'NONE', #605, #2822, #15014 ) ;
#28030=CARTESIAN_POINT ( 'NONE',  ( 15.17214319754856966, -5.086913993735587169, 1.171642046065942910 ) ) ;
#28031=COLOUR_RGB ( '', 0.40784314, 0.44705882, 0.49803922) ;
#28035=ORIENTED_EDGE ( 'NONE', *, *, #21348, .F. ) ;
#28036=CIRCLE ( 'NONE', #740, 3.299999999999999822 ) ;
#28039=EDGE_CURVE ( 'NONE', #19112, #13995, #8972, .T. ) ;
#28049=CIRCLE ( 'NONE', #6308, 4.299999999999998046 ) ;
#28054=CARTESIAN_POINT ( 'NONE',  ( 46.90000000000001279, 1.734723475976807094E-15, 0.000000000000000000 ) ) ;
#28058=CARTESIAN_POINT ( 'NONE',  ( 57.04126813003668417, 0.7492316407094400388, 2.421767203557310122 ) ) ;
#28059=CARTESIAN_POINT ( 'NONE',  ( -36.52757395963740095, 4.797343084509227751, -2.497389432263917186 ) ) ;
#28071=CARTESIAN_POINT ( 'NONE',  ( -36.72207054450174724, -0.6818242347930901781, -5.365311767243446717 ) ) ;
#28076=DIRECTION ( 'NONE',  ( 0.000000000000000000, 0.000000000000000000, 1.000000000000000000 ) ) ;
#28077=EDGE_LOOP ( 'NONE', ( #30642, #24046, #7049, #26951, #21272 ) ) ;
#28078=ORIENTED_EDGE ( 'NONE', *, *, #21332, .T. ) ;
#28082=EDGE_CURVE ( 'NONE', #1571, #15671, #22128, .T. ) ;
#28093=AXIS2_PLACEMENT_3D ( 'NONE', #12559, #24300, #5275 ) ;
#28096=CARTESIAN_POINT ( 'NONE',  ( 16.10667815269233216, -0.1434351685890333516, 5.407416993630366875 ) ) ;
#28097=CARTESIAN_POINT ( 'NONE',  ( 56.95000000000001705, -0.7137254901960785602, -2.500119182087999548 ) ) ;
#28101=DIRECTION ( 'NONE',  ( -0.000000000000000000, 1.000000000000000000, 0.000000000000000000 ) ) ;
#28102=CARTESIAN_POINT ( 'NONE',  ( 57.02118883257515591, 0.7413508443325595998, -1.786034507790101866 ) ) ;
#28103=CARTESIAN_POINT ( 'NONE',  ( 47.00000000000002132, -3.726179070414207928, 1.041421356237309803 ) ) ;
#28106=CARTESIAN_POINT ( 'NONE',  ( -53.99999999999997868, 0.000000000000000000, 0.000000000000000000 ) ) ;
#28107=AXIS2_PLACEMENT_3D ( 'NONE', #14890, #19821, #10154 ) ;
#28113=VERTEX_POINT ( 'NONE', #8819 ) ;
#28117=VECTOR ( 'NONE', #26184, 1000.000000000000000 ) ;
#28130=CARTESIAN_POINT ( 'NONE',  ( 15.03925126672132961, 0.4576450603547064788, -5.200000000000000178 ) ) ;
#28133=ORIENTED_EDGE ( 'NONE', *, *, #22207, .T. ) ;
#28135=AXIS2_PLACEMENT_3D ( 'NONE', #16841, #30809, #51 ) ;
#28137=TOROIDAL_SURFACE ( 'NONE', #4881, -24.59258869922086888, 30.00000000000000000 ) ;
#28146=AXIS2_PLACEMENT_3D ( 'NONE', #24045, #28807, #2356 ) ;
#28148=DIRECTION ( 'NONE',  ( 1.000000000000000000, 0.000000000000000000, 0.000000000000000000 ) ) ;
#28151=DIRECTION ( 'NONE',  ( 4.670714851210922627E-16, -0.9333474217026305197, -0.3589743589743593088 ) ) ;
#28157=CARTESIAN_POINT ( 'NONE',  ( 48.30000000000002558, 0.6462379109120998111, 4.048750000000022276 ) ) ;
#28161=LINE ( 'NONE', #18839, #8291 ) ;
#28166=CARTESIAN_POINT ( 'NONE',  ( 54.50000000000002132, -0.2842225609755594795, -1.577752156565102655E-15 ) ) ;
#28176=CARTESIAN_POINT ( 'NONE',  ( -35.85663232820584057, 1.793057972832144520, 4.026191436122060097 ) ) ;
#28180=AXIS2_PLACEMENT_3D ( 'NONE', #10210, #12733, #29224 ) ;
#28182=CARTESIAN_POINT ( 'NONE',  ( 57.03052440771394060, -0.7462437932013319397, 1.781707539322121336 ) ) ;
#28184=VERTEX_POINT ( 'NONE', #9938 ) ;
#28185=CARTESIAN_POINT ( 'NONE',  ( -36.56242893520638404, 3.003531019938693536, -4.498666779076329725 ) ) ;
#28186=DIRECTION ( 'NONE',  ( -0.000000000000000000, 0.000000000000000000, 1.000000000000000000 ) ) ;
#28188=CARTESIAN_POINT ( 'NONE',  ( 15.32752150720753725, -1.093737229520474363, -5.295968199484771155 ) ) ;
#28191=CARTESIAN_POINT ( 'NONE',  ( -44.49999999999997868, 0.000000000000000000, 0.000000000000000000 ) ) ;
#28194=ADVANCED_FACE ( 'NONE', ( #10093 ), #2507, .F. ) ;
#28197=CARTESIAN_POINT ( 'NONE',  ( 50.30848954602731737, -1.391941090707485396, -3.850000000000024070 ) ) ;
#28205=CARTESIAN_POINT ( 'NONE',  ( 15.95705409078442649, -4.926689578693679294, 2.233438676318023397 ) ) ;
#28208=CARTESIAN_POINT ( 'NONE',  ( 50.39884346364544854, -0.8930148142854128501, 3.925689827643444652 ) ) ;
#28209=AXIS2_PLACEMENT_3D ( 'NONE', #22925, #23392, #1379 ) ;
#28219=VERTEX_POINT ( 'NONE', #28724 ) ;
#28223=EDGE_LOOP ( 'NONE', ( #12973, #20355, #16940, #19581 ) ) ;
#28226=CARTESIAN_POINT ( 'NONE',  ( -35.85663232820584057, -4.018128179617557194, 3.618665901676652918 ) ) ;
#28230=AXIS2_PLACEMENT_3D ( 'NONE', #9734, #29345, #10333 ) ;
#28233=EDGE_CURVE ( 'NONE', #27954, #21815, #9492, .T. ) ;
#28235=DIRECTION ( 'NONE',  ( -1.520093157366848107E-16, 0.5877852522924625900, 0.8090169943749551118 ) ) ;
#28237=FACE_OUTER_BOUND ( 'NONE', #5734, .T. ) ;
#28241=CARTESIAN_POINT ( 'NONE',  ( 50.36024759664407213, 1.282505688586122572, -3.869483523004607406 ) ) ;
#28244=CARTESIAN_POINT ( 'NONE',  ( 50.50000000000001421, -0.6462379109120508502, 4.048750000000023164 ) ) ;
#28246=ORIENTED_EDGE ( 'NONE', *, *, #20116, .T. ) ;
#28257=ORIENTED_EDGE ( 'NONE', *, *, #5592, .F. ) ;
#28263=CARTESIAN_POINT ( 'NONE',  ( 46.99978405390194780, -4.243814194680251006, -1.064485530476996455 ) ) ;
#28274=EDGE_CURVE ( 'NONE', #22777, #30315, #30720, .T. ) ;
#28280=EDGE_LOOP ( 'NONE', ( #1000, #7311, #21951, #18802 ) ) ;
#28281=ORIENTED_EDGE ( 'NONE', *, *, #22298, .T. ) ;
#28291=CARTESIAN_POINT ( 'NONE',  ( 47.00000000000002132, 2.428612866367529932E-14, 0.000000000000000000 ) ) ;
#28297=DIRECTION ( 'NONE',  ( 1.000000000000000000, -0.000000000000000000, -0.000000000000000000 ) ) ;
#28298=CARTESIAN_POINT ( 'NONE',  ( -35.85663232820584057, -4.945493884734804446, -1.606888370749739448 ) ) ;
#28299=DIRECTION ( 'NONE',  ( 0.000000000000000000, 0.000000000000000000, 1.000000000000000000 ) ) ;
#28300=ORIENTED_EDGE ( 'NONE', *, *, #4075, .T. ) ;
#28301=CARTESIAN_POINT ( 'NONE',  ( -36.26369610968575330, 5.012449653004628303, -1.400819699605756696 ) ) ;
#28304=VECTOR ( 'NONE', #19160, 1000.000000000000000 ) ;
#28305=DIRECTION ( 'NONE',  ( 0.000000000000000000, 0.9663289263986323263, -0.2573099415204678220 ) ) ;
#28306=CARTESIAN_POINT ( 'NONE',  ( 57.00000000000001421, -0.6999999999999999556, 2.452039967047845437 ) ) ;
#28311=CARTESIAN_POINT ( 'NONE',  ( 50.42115343657336268, 0.9200365198983971871, -3.998286360709619736 ) ) ;
#28315=VERTEX_POINT ( 'NONE', #12237 ) ;
#28318=CARTESIAN_POINT ( 'NONE',  ( -36.76447480099743359, 0.6031025731809287471, 5.374022845360671319 ) ) ;
#28323=ORIENTED_EDGE ( 'NONE', *, *, #15229, .F. ) ;
#28325=CARTESIAN_POINT ( 'NONE',  ( 48.50000000000002132, 1.391941090707540685, 3.850000000000022293 ) ) ;
#28333=LINE ( 'NONE', #1708, #24121 ) ;
#28340=DIRECTION ( 'NONE',  ( 2.459562394685743786E-16, -0.9510565162951521989, -0.3090169943749515591 ) ) ;
#28341=ADVANCED_FACE ( 'NONE', ( #15076 ), #30239, .T. ) ;
#28342=VERTEX_POINT ( 'NONE', #3519 ) ;
#28343=DIRECTION ( 'NONE',  ( -1.000000000000000000, -0.000000000000000000, -0.000000000000000000 ) ) ;
#28348=CARTESIAN_POINT ( 'NONE',  ( 57.01182421275571954, -0.7322894606377696736, -2.432677346698721266 ) ) ;
#28358=CARTESIAN_POINT ( 'NONE',  ( -44.49999999999997868, 1.499999999999999556, 4.029888335921975262 ) ) ;
#28360=CARTESIAN_POINT ( 'NONE',  ( -36.30347965937241383, 4.980680447166604630, 1.498595263773591757 ) ) ;
#28364=CARTESIAN_POINT ( 'NONE',  ( -36.77443515226921278, -5.298557911012516719, 1.088945631943563752 ) ) ;
#28365=CARTESIAN_POINT ( 'NONE',  ( -35.85663232820584767, 4.817150320980633005, 2.203324261490556157 ) ) ;
#28367=EDGE_LOOP ( 'NONE', ( #18061, #20087, #4380, #14449, #4445 ) ) ;
#28369=AXIS2_PLACEMENT_3D ( 'NONE', #8687, #11076, #1416 ) ;
#28375=ORIENTED_EDGE ( 'NONE', *, *, #12639, .T. ) ;
#28382=VECTOR ( 'NONE', #28476, 1000.000000000000000 ) ;
#28387=ADVANCED_FACE ( 'NONE', ( #30407 ), #20318, .T. ) ;
#28391=CARTESIAN_POINT ( 'NONE',  ( 50.50000000000002132, 2.428612866367529932E-14, -4.000000000000022204 ) ) ;
#28395=CARTESIAN_POINT ( 'NONE',  ( 50.33036399986576015, 1.366688880095624503, -3.854642372925540350 ) ) ;
#28407=CARTESIAN_POINT ( 'NONE',  ( 16.07279755198631577, 5.034707333629180326, 1.977875755500474231 ) ) ;
#28411=CARTESIAN_POINT ( 'NONE',  ( -35.85663232820584057, -1.123735532908286316, 5.289358697221548944 ) ) ;
#28415=ADVANCED_FACE ( 'NONE', ( #1440 ), #8711, .F. ) ;
#28418=EDGE_LOOP ( 'NONE', ( #10058, #11969, #24702, #1455 ) ) ;
#28422=CARTESIAN_POINT ( 'NONE',  ( 56.97364842551142061, -0.7795706648299629560, -2.480376902516343129 ) ) ;
#28423=ORIENTED_EDGE ( 'NONE', *, *, #5976, .T. ) ;
#28425=CARTESIAN_POINT ( 'NONE',  ( 58.50000000000001421, -0.8000000000000000444, 2.471260002560649927 ) ) ;
#28427=DIRECTION ( 'NONE',  ( -1.000000000000000000, 0.000000000000000000, 0.000000000000000000 ) ) ;
#28428=CARTESIAN_POINT ( 'NONE',  ( -36.89017861346991367, -2.910597594660151000, 4.559461819278090466 ) ) ;
#28430=AXIS2_PLACEMENT_3D ( 'NONE', #12433, #22125, #112 ) ;
#28431=EDGE_CURVE ( 'NONE', #2309, #15602, #17087, .T. ) ;
#28432=DIRECTION ( 'NONE',  ( 0.000000000000000000, 1.000000000000000000, 0.000000000000000000 ) ) ;
#28435=EDGE_LOOP ( 'NONE', ( #14410, #18510, #20676, #5430 ) ) ;
#28443=DIRECTION ( 'NONE',  ( -1.000000000000000000, 0.000000000000000000, 0.000000000000000000 ) ) ;
#28445=ORIENTED_EDGE ( 'NONE', *, *, #26516, .T. ) ;
#28446=CARTESIAN_POINT ( 'NONE',  ( 51.70000000000001705, -4.276948333784438283, 0.9210526315789470120 ) ) ;
#28450=CARTESIAN_POINT ( 'NONE',  ( -36.52679053911622731, 4.797009389500119347, 2.498041539401855360 ) ) ;
#28452=ORIENTED_EDGE ( 'NONE', *, *, #24799, .F. ) ;
#28453=CARTESIAN_POINT ( 'NONE',  ( 57.00000000000001421, -0.6999999999999996225, 1.820027472320129736 ) ) ;
#28454=EDGE_CURVE ( 'NONE', #6920, #23306, #16562, .T. ) ;
#28462=FACE_OUTER_BOUND ( 'NONE', #19310, .T. ) ;
#28466=ADVANCED_FACE ( 'NONE', ( #3975 ), #22579, .T. ) ;
#28471=CARTESIAN_POINT ( 'NONE',  ( -36.92443669619682112, -0.1565107631087878926, 5.407502298984291578 ) ) ;
#28473=VERTEX_POINT ( 'NONE', #18557 ) ;
#28474=CARTESIAN_POINT ( 'NONE',  ( -54.46439202372638277, 1.502116081466616793, 4.031358338852112588 ) ) ;
#28476=DIRECTION ( 'NONE',  ( -0.000000000000000000, 0.000000000000000000, 1.000000000000000000 ) ) ;
#28479=EDGE_LOOP ( 'NONE', ( #14328, #27120, #19076, #14686, #19954, #7650, #14914, #15461, #18445, #11635 ) ) ;
#28483=DIRECTION ( 'NONE',  ( 6.938893903907228378E-15, 8.673617379884035472E-16, 1.000000000000000000 ) ) ;
#28488=DIRECTION ( 'NONE',  ( -1.000000000000000000, -2.586136946169074517E-16, 0.000000000000000000 ) ) ;
#28490=CARTESIAN_POINT ( 'NONE',  ( -35.85663232820584057, 3.275050215670975540, -2.949461045525604508 ) ) ;
#28492=DIRECTION ( 'NONE',  ( 1.000000000000000000, 0.000000000000000000, 0.000000000000000000 ) ) ;
#28494=CARTESIAN_POINT ( 'NONE',  ( -54.49983703358571319, 1.542636180423123449, -4.059406436927352146 ) ) ;
#28496=CARTESIAN_POINT ( 'NONE',  ( 57.00000000000001421, -0.6999999999999999556, 1.820027472320129736 ) ) ;
#28497=CARTESIAN_POINT ( 'NONE',  ( -36.43290890416709971, 3.561547362098881120, -4.076645242318375217 ) ) ;
#28500=CARTESIAN_POINT ( 'NONE',  ( 15.70940947763170925, -0.8934212604923321699, -5.334164326942877565 ) ) ;
#28504=CIRCLE ( 'NONE', #29027, 0.4576450603546982632 ) ;
#28507=FACE_OUTER_BOUND ( 'NONE', #25867, .T. ) ;
#28513=CARTESIAN_POINT ( 'NONE',  ( -36.04518387042686101, 5.340403875751171370, 0.9205822004573066542 ) ) ;
#28517=CARTESIAN_POINT ( 'NONE',  ( -35.98952425903308949, -4.804073785499180183, 2.042134698606323351 ) ) ;
#28518=CARTESIAN_POINT ( 'NONE',  ( -35.85663232820584057, 4.945493884734773360, 1.606888370749773864 ) ) ;
#28527=ORIENTED_EDGE ( 'NONE', *, *, #4331, .T. ) ;
#28537=CARTESIAN_POINT ( 'NONE',  ( -35.85663232820584767, 5.377732432866631385, -0.5657657256215208319 ) ) ;
#28539=( BOUNDED_SURFACE ( )  B_SPLINE_SURFACE ( 3, 2, ( 
 ( #8909, #18596, #28244 ),
 ( #13330, #16212, #25861 ),
 ( #4163, #5934, #15591 ),
 ( #23028, #25237, #3556 ),
 ( #13193, #2258, #9246 ),
 ( #9399, #4635, #23813 ),
 ( #21608, #14138, #4789 ),
 ( #7033, #2105, #11769 ),
 ( #13966, #30772, #28873 ),
 ( #21444, #2432, #7331 ) ),
 .UNSPECIFIED., .F., .F., .F. ) 
 B_SPLINE_SURFACE_WITH_KNOTS ( ( 4, 2, 2, 2, 4 ),
 ( 3, 3 ),
 ( 0.0004005301535625021940, 0.0008279283193725978313, 0.001041627402277645704, 0.001148476943730169586, 0.001255326485182693469 ),
 ( 0.000000000000000000, 1.000000000000000000 ),
 .UNSPECIFIED. ) 
 GEOMETRIC_REPRESENTATION_ITEM ( )  RATIONAL_B_SPLINE_SURFACE ( (
 ( 1.000000000000000000, 0.7071067811865475727, 1.000000000000000000),
 ( 1.000000000000000000, 0.7463463187144472322, 1.000000000000000000),
 ( 1.000000000000000000, 0.7946150999565784190, 1.000000000000000000),
 ( 1.000000000000000000, 0.8720431506958271628, 1.000000000000000000),
 ( 1.000000000000000000, 0.8987780092779085184, 1.000000000000000000),
 ( 1.000000000000000000, 0.9375340664365013899, 1.000000000000000000),
 ( 1.000000000000000000, 0.9504270566176250545, 1.000000000000000000),
 ( 1.000000000000000000, 0.9732249474031241521, 1.000000000000000000),
 ( 1.000000000000000000, 0.9839441327696755168, 1.000000000000000000),
 ( 1.000000000000000000, 0.9842509842514762797, 1.000000000000000000) ) ) 
 REPRESENTATION_ITEM ( '' )  SURFACE ( )  );
#28540=CARTESIAN_POINT ( 'NONE',  ( 46.92078115823489526, -4.254539148539595139, 1.020319270753726082 ) ) ;
#28542=CARTESIAN_POINT ( 'NONE',  ( 15.56274145962646394, 5.369990034204301210, -0.6654225812208519608 ) ) ;
#28547=ORIENTED_EDGE ( 'NONE', *, *, #20025, .T. ) ;
#28549=CARTESIAN_POINT ( 'NONE',  ( 48.47377487419020525, -1.373801017329605134, -3.853344662332955473 ) ) ;
#28557=VERTEX_POINT ( 'NONE', #7291 ) ;
#28558=EDGE_LOOP ( 'NONE', ( #10182, #3825, #183, #1414, #18837, #25119, #3514, #17280, #20564 ) ) ;
#28559=CARTESIAN_POINT ( 'NONE',  ( 16.07512358269905306, 5.233646053067070980, 1.367284724151327513 ) ) ;
#28562=ADVANCED_FACE ( 'NONE', ( #5220 ), #7471, .T. ) ;
#28565=CARTESIAN_POINT ( 'NONE',  ( 58.45000000000001705, 0.8000000000000000444, 2.421260002560649660 ) ) ;
#28568=EDGE_CURVE ( 'NONE', #6093, #30315, #7747, .T. ) ;
#28575=CARTESIAN_POINT ( 'NONE',  ( 56.96603746669009638, -0.7703957983921196906, -2.483260519405945388 ) ) ;
#28579=ADVANCED_FACE ( 'NONE', ( #12203 ), #24079, .T. ) ;
#28583=CARTESIAN_POINT ( 'NONE',  ( 50.50000000000002132, 0.6462379109121000331, -4.048750000000023164 ) ) ;
#28585=CYLINDRICAL_SURFACE ( 'NONE', #12442, 4.700000000000000178 ) ;
#28587=DIRECTION ( 'NONE',  ( 1.000000000000000000, 0.000000000000000000, 0.000000000000000000 ) ) ;
#28599=CARTESIAN_POINT ( 'NONE',  ( -36.76447480099743359, 3.646691605040315309, 3.993181011920730050 ) ) ;
#28602=ORIENTED_EDGE ( 'NONE', *, *, #6084, .T. ) ;
#28610=EDGE_CURVE ( 'NONE', #30315, #13545, #14578, .T. ) ;
#28613=EDGE_CURVE ( 'NONE', #24288, #21815, #23, .T. ) ;
#28630=CARTESIAN_POINT ( 'NONE',  ( -36.11780688638206982, -1.123735543662337300, 5.289358694936827199 ) ) ;
#28632=ADVANCED_FACE ( 'NONE', ( #170 ), #29297, .T. ) ;
#28635=CARTESIAN_POINT ( 'NONE',  ( -35.85663232820583346, -5.377732432866661583, 0.5657657256215455899 ) ) ;
#28636=ORIENTED_EDGE ( 'NONE', *, *, #24908, .T. ) ;
#28642=ORIENTED_EDGE ( 'NONE', *, *, #5008, .F. ) ;
#28643=DIRECTION ( 'NONE',  ( 1.000000000000000000, 0.000000000000000000, -0.000000000000000000 ) ) ;
#28644=LINE ( 'NONE', #19165, #17679 ) ;
#28645=AXIS2_PLACEMENT_3D ( 'NONE', #13497, #6229, #15587 ) ;
#28646=LINE ( 'NONE', #16776, #26172 ) ;
#28663=CARTESIAN_POINT ( 'NONE',  ( -36.76447480099743359, 2.670851142931450539, -4.702170608191241108 ) ) ;
#28669=VECTOR ( 'NONE', #6505, 1000.000000000000000 ) ;
#28675=DIRECTION ( 'NONE',  ( 1.000000000000000000, 2.586136946169074517E-16, -0.000000000000000000 ) ) ;
#28677=EDGE_CURVE ( 'NONE', #17963, #18266, #4954, .T. ) ;
#28682=CARTESIAN_POINT ( 'NONE',  ( 15.74504787372211645, -3.003531019938647795, -4.498666779076351929 ) ) ;
#28683=CARTESIAN_POINT ( 'NONE',  ( -36.68133364217572989, 5.320649567603461527, 0.9667173501064365571 ) ) ;
#28684=CARTESIAN_POINT ( 'NONE',  ( 15.41217651307628600, -5.027944117023993797, 1.353132643598594864 ) ) ;
#28685=ORIENTED_EDGE ( 'NONE', *, *, #4355, .T. ) ;
#28691=AXIS2_PLACEMENT_3D ( 'NONE', #20818, #31216, #30448 ) ;
#28694=ORIENTED_EDGE ( 'NONE', *, *, #4275, .F. ) ;
#28695=( NAMED_UNIT ( * ) SI_UNIT ( $, .STERADIAN. ) SOLID_ANGLE_UNIT ( ) );
#28697=CARTESIAN_POINT ( 'NONE',  ( -54.44999999999997442, 1.499999999999998890, 3.300094695611021756 ) ) ;
#28701=ORIENTED_EDGE ( 'NONE', *, *, #19113, .T. ) ;
#28706=DIRECTION ( 'NONE',  ( -1.000000000000000000, 0.000000000000000000, 0.000000000000000000 ) ) ;
#28707=CARTESIAN_POINT ( 'NONE',  ( -35.85663232820584057, 4.945493884734773360, 1.606888370749773864 ) ) ;
#28709=DIRECTION ( 'NONE',  ( -1.000000000000000000, -0.000000000000000000, -0.000000000000000000 ) ) ;
#28710=DIRECTION ( 'NONE',  ( -1.000000000000000000, 0.000000000000000000, 0.000000000000000000 ) ) ;
#28713=CARTESIAN_POINT ( 'NONE',  ( 47.10000000000002984, -4.259946800035232073, 0.9999999999999998890 ) ) ;
#28715=CARTESIAN_POINT ( 'NONE',  ( 15.74504787372188552, 5.206628483174362998, -1.466363261642694704 ) ) ;
#28718=AXIS2_PLACEMENT_3D ( 'NONE', #4555, #4395, #23879 ) ;
#28722=CARTESIAN_POINT ( 'NONE',  ( -35.85663232820584767, -4.383220986680273157, 0.4611378927884406398 ) ) ;
#28723=CARTESIAN_POINT ( 'NONE',  ( 48.40000000000001990, -0.6304760106459033064, -3.950000000000022826 ) ) ;
#28724=CARTESIAN_POINT ( 'NONE',  ( 56.95000000000001705, 2.326828918379971365E-16, 1.899999999999999911 ) ) ;
#28727=EDGE_LOOP ( 'NONE', ( #2403, #22565, #18566, #15561 ) ) ;
#28728=CYLINDRICAL_SURFACE ( 'NONE', #7569, 1.899999999999999911 ) ;
#28735=CARTESIAN_POINT ( 'NONE',  ( 48.41845806530709240, -1.153441674035701636, 3.890342980189690270 ) ) ;
#28737=ORIENTED_EDGE ( 'NONE', *, *, #4673, .F. ) ;
#28738=DIRECTION ( 'NONE',  ( 1.000000000000000000, -0.000000000000000000, -0.000000000000000000 ) ) ;
#28739=CARTESIAN_POINT ( 'NONE',  ( 48.40000000000001990, 1.391941090707534245, -3.850000000000022737 ) ) ;
#28741=AXIS2_PLACEMENT_3D ( 'NONE', #6605, #18334, #23242 ) ;
#28748=LINE ( 'NONE', #28425, #19087 ) ;
#28755=DIRECTION ( 'NONE',  ( -1.000000000000000000, -0.000000000000000000, -0.000000000000000000 ) ) ;
#28757=ADVANCED_FACE ( 'NONE', ( #16603 ), #3931, .T. ) ;
#28758=CIRCLE ( 'NONE', #19659, 4.700000000000000178 ) ;
#28759=TOROIDAL_SURFACE ( 'NONE', #9563, 1.850000000000000089, 0.05000000000000000278 ) ;
#28761=ORIENTED_EDGE ( 'NONE', *, *, #24260, .T. ) ;
#28768=ORIENTED_EDGE ( 'NONE', *, *, #30372, .F. ) ;
#28769=DIRECTION ( 'NONE',  ( -1.000000000000000000, -2.586136946169074517E-16, 0.000000000000000000 ) ) ;
#28770=EDGE_CURVE ( 'NONE', #18491, #6711, #22672, .T. ) ;
#28772=CARTESIAN_POINT ( 'NONE',  ( 50.36079629521400847, 1.278211010209494347, 3.870212229389975889 ) ) ;
#28774=CARTESIAN_POINT ( 'NONE',  ( 56.99229187639506478, -0.7794873559220516501, 1.732743334125896428 ) ) ;
#28775=CARTESIAN_POINT ( 'NONE',  ( 57.03643325641707662, 0.7481242503215885797, 1.780024810282529790 ) ) ;
#28782=DIRECTION ( 'NONE',  ( -1.000000000000000000, 0.000000000000000000, 0.000000000000000000 ) ) ;
#28786=CARTESIAN_POINT ( 'NONE',  ( -36.14490256869205353, -1.093737229520479470, 5.295968199484772931 ) ) ;
#28788=AXIS2_PLACEMENT_3D ( 'NONE', #16241, #8942, #25565 ) ;
#28792=CARTESIAN_POINT ( 'NONE',  ( -54.47366401599046526, 1.505709097230404359, 3.303769268891089794 ) ) ;
#28795=CARTESIAN_POINT ( 'NONE',  ( -54.49999999999997868, 1.549999999999999600, 4.064480286580312907 ) ) ;
#28796=VERTEX_POINT ( 'NONE', #16426 ) ;
#28797=CARTESIAN_POINT ( 'NONE',  ( 15.49676243306307732, 0.05686983728432184332, -5.199999998843000348 ) ) ;
#28800=VERTEX_POINT ( 'NONE', #2331 ) ;
#28801=ORIENTED_EDGE ( 'NONE', *, *, #15021, .F. ) ;
#28804=AXIS2_PLACEMENT_3D ( 'NONE', #2844, #9989, #7609 ) ;
#28807=DIRECTION ( 'NONE',  ( 1.000000000000000000, 0.000000000000000000, 0.000000000000000000 ) ) ;
#28808=ORIENTED_EDGE ( 'NONE', *, *, #14964, .T. ) ;
#28819=EDGE_CURVE ( 'NONE', #26590, #9481, #19619, .T. ) ;
#28820=DIRECTION ( 'NONE',  ( 0.000000000000000000, 0.000000000000000000, -1.000000000000000000 ) ) ;
#28821=CARTESIAN_POINT ( 'NONE',  ( 57.05000000000001847, -0.8000000000000000444, 2.471260002560650371 ) ) ;
#28824=VECTOR ( 'NONE', #8677, 1000.000000000000114 ) ;
#28825=AXIS2_PLACEMENT_3D ( 'NONE', #8392, #28186, #22969 ) ;
#28827=DIRECTION ( 'NONE',  ( 1.000000000000000000, 2.586136946169074517E-16, -0.000000000000000000 ) ) ;
#28829=CIRCLE ( 'NONE', #2531, 4.650000000000000355 ) ;
#28835=CARTESIAN_POINT ( 'NONE',  ( 50.50000000000002132, -0.6462379109120509613, 4.048750000000023164 ) ) ;
#28836=CARTESIAN_POINT ( 'NONE',  ( -36.48174642953026137, 5.256245472275701047, 1.286369972357462199 ) ) ;
#28837=CARTESIAN_POINT ( 'NONE',  ( 15.29449157529473702, -4.822464347458966571, 1.985534350301629392 ) ) ;
#28839=ORIENTED_EDGE ( 'NONE', *, *, #23367, .F. ) ;
#28842=CARTESIAN_POINT ( 'NONE',  ( 56.95000000000001705, 0.7137254901960785602, -2.500119182087999548 ) ) ;
#28856=ADVANCED_FACE ( 'NONE', ( #9639 ), #17297, .T. ) ;
#28862=DIRECTION ( 'NONE',  ( 0.000000000000000000, 0.000000000000000000, 1.000000000000000000 ) ) ;
#28864=CARTESIAN_POINT ( 'NONE',  ( 47.10000000000002984, -4.179189514726507682, 0.9999999999999997780 ) ) ;
#28866=CARTESIAN_POINT ( 'NONE',  ( 15.94709373951304343, 5.297368390263439863, -1.087079755157641880 ) ) ;
#28870=DIRECTION ( 'NONE',  ( 1.000000000000000000, 0.000000000000000000, 0.000000000000000000 ) ) ;
#28872=CARTESIAN_POINT ( 'NONE',  ( 48.40000000000002700, -0.6304760106459033064, 3.950000000000022826 ) ) ;
#28873=CARTESIAN_POINT ( 'NONE',  ( 50.33755732750837097, -1.426738769040649224, 3.843750315111184257 ) ) ;
#28875=DIRECTION ( 'NONE',  ( 1.000000000000000000, 2.586136946169074517E-16, -0.000000000000000000 ) ) ;
#28909=CARTESIAN_POINT ( 'NONE',  ( -35.85663232820584767, 3.817150320980676081, -2.203324261490498426 ) ) ;
#28912=DIRECTION ( 'NONE',  ( 1.000000000000000000, 0.000000000000000000, 0.000000000000000000 ) ) ;
#28914=VERTEX_POINT ( 'NONE', #24191 ) ;
#28917=CARTESIAN_POINT ( 'NONE',  ( 33.47623932017462778, -5.377732432866642931, 0.5657657256215455899 ) ) ;
#28919=CARTESIAN_POINT ( 'NONE',  ( -36.14490256869206064, 4.698781674909465522, 2.676750094560181203 ) ) ;
#28921=CARTESIAN_POINT ( 'NONE',  ( 56.95000000000001705, -0.6820512820512815155, 1.773360101234998210 ) ) ;
#28929=DIRECTION ( 'NONE',  ( 0.000000000000000000, -1.000000000000000000, -1.224646799147352961E-16 ) ) ;
#28931=EDGE_CURVE ( 'NONE', #9397, #17741, #30214, .T. ) ;
#28933=CARTESIAN_POINT ( 'NONE',  ( -36.89831264271880684, 0.2888463313200247407, 5.401384060636566176 ) ) ;
#28937=CARTESIAN_POINT ( 'NONE',  ( -54.49865678108456279, 1.537045020190657585, 3.323865043138458208 ) ) ;
#28940=CARTESIAN_POINT ( 'NONE',  ( -54.49409853110120139, 1.525884777627347644, 4.047834655405393889 ) ) ;
#28942=CARTESIAN_POINT ( 'NONE',  ( 15.49702763512084047, -0.05469410396135043068, -5.200000001156997342 ) ) ;
#28951=ORIENTED_EDGE ( 'NONE', *, *, #13531, .F. ) ;
#28955=CARTESIAN_POINT ( 'NONE',  ( 16.08093158123429944, -2.941172302009019468, -4.539591111929662581 ) ) ;
#28960=AXIS2_PLACEMENT_3D ( 'NONE', #19108, #28755, #7068 ) ;
#28961=DIRECTION ( 'NONE',  ( 1.000000000000000000, 0.000000000000000000, 0.000000000000000000 ) ) ;
#28962=ADVANCED_FACE ( 'NONE', ( #3106 ), #29041, .T. ) ;
#28965=CARTESIAN_POINT ( 'NONE',  ( 15.56274145962646926, -3.953287617511611174, 3.694739123711129558 ) ) ;
#28966=CARTESIAN_POINT ( 'NONE',  ( 48.39188949082539182, 1.340787288841451819, -3.874691554877328414 ) ) ;
#28975=ORIENTED_EDGE ( 'NONE', *, *, #15447, .T. ) ;
#28980=CARTESIAN_POINT ( 'NONE',  ( -36.77443515226919857, 4.926689578693665972, 2.233438676318016292 ) ) ;
#28981=DIRECTION ( 'NONE',  ( 1.000000000000000000, 0.000000000000000000, 0.000000000000000000 ) ) ;
#28983=ORIENTED_EDGE ( 'NONE', *, *, #28039, .T. ) ;
#28987=ORIENTED_EDGE ( 'NONE', *, *, #6615, .T. ) ;
#28988=EDGE_CURVE ( 'NONE', #17666, #7967, #7406, .T. ) ;
#28993=CARTESIAN_POINT ( 'NONE',  ( -36.48174642952978530, -5.256245472275803188, -1.286369972357330749 ) ) ;
#28999=EDGE_CURVE ( 'NONE', #11630, #10988, #10240, .T. ) ;
#29009=CARTESIAN_POINT ( 'NONE',  ( -36.48821680285183788, 0.3995010896672961942, -5.397102918580238828 ) ) ;
#29012=CARTESIAN_POINT ( 'NONE',  ( 54.49932581792542408, -0.002837702348961988318, -4.287546236934917765 ) ) ;
#29018=DIRECTION ( 'NONE',  ( 1.000000000000000000, -0.000000000000000000, -0.000000000000000000 ) ) ;
#29019=CARTESIAN_POINT ( 'NONE',  ( 48.43975240335598897, -1.282505688586073944, -3.869483523004607406 ) ) ;
#29027=AXIS2_PLACEMENT_3D ( 'NONE', #23159, #11103, #18398 ) ;
#29031=EDGE_LOOP ( 'NONE', ( #26494, #12215, #3477, #17827, #180 ) ) ;
#29034=CARTESIAN_POINT ( 'NONE',  ( 48.47372026270297596, -1.373706569044463199, 3.853361913240786141 ) ) ;
#29037=CARTESIAN_POINT ( 'NONE',  ( 54.49860577577695864, -0.002682860454229076680, 4.292318283074051166 ) ) ;
#29040=VERTEX_POINT ( 'NONE', #27485 ) ;
#29041=( BOUNDED_SURFACE ( )  B_SPLINE_SURFACE ( 3, 2, ( 
 ( #26860, #19759, #26726 ),
 ( #8021, #14678, #5488 ),
 ( #14816, #12754, #21973 ),
 ( #20067, #263, #127 ),
 ( #432, #12294, #2795 ),
 ( #14826, #10392, #9937 ),
 ( #24804, #19616, #5649 ),
 ( #22438, #20077, #581 ),
 ( #5025, #27185, #9780 ),
 ( #3114, #21841, #27337 ),
 ( #29253, #24344, #10092 ),
 ( #19763, #26867, #733 ),
 ( #14984, #29714, #2505 ),
 ( #17081, #29394, #19446 ),
 ( #15302, #12451, #8029 ),
 ( #5177, #17534, #17694 ) ),
 .UNSPECIFIED., .F., .F., .F. ) 
 B_SPLINE_SURFACE_WITH_KNOTS ( ( 4, 2, 2, 2, 2, 2, 2, 4 ),
 ( 3, 3 ),
 ( 0.001780502285214259975, 0.002558945925323794120, 0.002753556835351177873, 0.002948167745378561192, 0.003337389565433328265, 0.003726611385488095337, 0.004115833205542862409, 0.004894276845652396554 ),
 ( 0.000000000000000000, 1.000000000000000000 ),
 .UNSPECIFIED. ) 
 GEOMETRIC_REPRESENTATION_ITEM ( )  RATIONAL_B_SPLINE_SURFACE ( (
 ( 1.000000000000000000, 0.9418517008537217183, 1.000000000000000000),
 ( 1.000000000000000000, 0.9417987965885166179, 1.000000000000000000),
 ( 1.000000000000000000, 0.9418198861733918514, 1.000000000000000000),
 ( 1.000000000000000000, 0.9434060303845587248, 1.000000000000000000),
 ( 1.000000000000000000, 0.9437939819948625297, 1.000000000000000000),
 ( 1.000000000000000000, 0.9445989566712326146, 1.000000000000000000),
 ( 1.000000000000000000, 0.9450169930050459355, 1.000000000000000000),
 ( 1.000000000000000000, 0.9461610507672288950, 1.000000000000000000),
 ( 1.000000000000000000, 0.9467217966428351783, 1.000000000000000000),
 ( 1.000000000000000000, 0.9467345476123190107, 1.000000000000000000),
 ( 1.000000000000000000, 0.9461964028051400577, 1.000000000000000000),
 ( 1.000000000000000000, 0.9446801822475351385, 1.000000000000000000),
 ( 1.000000000000000000, 0.9437582546536535943, 1.000000000000000000),
 ( 1.000000000000000000, 0.9418129560295680491, 1.000000000000000000),
 ( 1.000000000000000000, 0.9418016889777458545, 1.000000000000000000),
 ( 1.000000000000000000, 0.9418517008537214963, 1.000000000000000000) ) ) 
 REPRESENTATION_ITEM ( '' )  SURFACE ( )  );
#29042=DIRECTION ( 'NONE',  ( 0.000000000000000000, -0.2745098039215694841, 0.9615843008030765526 ) ) ;
#29046=CARTESIAN_POINT ( 'NONE',  ( 34.55000000000001847, 0.000000000000000000, 0.000000000000000000 ) ) ;
#29048=CARTESIAN_POINT ( 'NONE',  ( 57.05000000000001847, -0.8000000000000000444, 1.778341924377873751 ) ) ;
#29051=B_SPLINE_CURVE_WITH_KNOTS ( 'NONE', 3,
 ( #28723, #9574, #11617, #26336, #14447, #6702, #29019, #17002, #26653, #11454, #28549, #9082, #19232, #21770 ),
 .UNSPECIFIED., .F., .F.,
 ( 4, 2, 2, 2, 2, 2, 4 ),
 ( 0.000000000000000000, 0.0003953907277084696219, 0.0005930860915627040805, 0.0006919337734898216080, 0.0007413576144533806428, 0.0007660695349351558233, 0.0007907814554169310039 ),
 .UNSPECIFIED. ) ;
#29053=CARTESIAN_POINT ( 'NONE',  ( 36.50000000000002132, 0.8000000000000000444, 1.778341924377873751 ) ) ;
#29055=AXIS2_PLACEMENT_3D ( 'NONE', #22003, #7729, #17391 ) ;
#29056=VERTEX_POINT ( 'NONE', #4162 ) ;
#29057=EDGE_CURVE ( 'NONE', #1093, #3490, #2921, .T. ) ;
#29058=ORIENTED_EDGE ( 'NONE', *, *, #9608, .T. ) ;
#29062=DIRECTION ( 'NONE',  ( 0.000000000000000000, 0.000000000000000000, -1.000000000000000000 ) ) ;
#29070=VERTEX_POINT ( 'NONE', #4013 ) ;
#29073=CARTESIAN_POINT ( 'NONE',  ( 50.36610310744725183, 1.399562922973069057, 3.853849143137397792 ) ) ;
#29079=CARTESIAN_POINT ( 'NONE',  ( 56.99229187639506478, 0.7794873559220516501, -1.732743334125896428 ) ) ;
#29085=CIRCLE ( 'NONE', #26049, 0.04999999999999991257 ) ;
#29094=ORIENTED_EDGE ( 'NONE', *, *, #3069, .F. ) ;
#29095=ADVANCED_FACE ( 'NONE', ( #5978 ), #12915, .T. ) ;
#29096=CARTESIAN_POINT ( 'NONE',  ( -36.92398358572909700, -5.231589534716087009, 1.397536681175191475 ) ) ;
#29099=CARTESIAN_POINT ( 'NONE',  ( 15.03925126672126034, 0.7747498368337761843, -5.363501452440937456 ) ) ;
#29100=CARTESIAN_POINT ( 'NONE',  ( -36.56242893520637693, -5.074157625981839281, 1.874066637979944883 ) ) ;
#29103=ORIENTED_EDGE ( 'NONE', *, *, #7527, .T. ) ;
#29105=DIRECTION ( 'NONE',  ( 0.000000000000000000, 1.000000000000000000, 0.000000000000000000 ) ) ;
#29117=PLANE ( 'NONE',  #1730 ) ;
#29121=CARTESIAN_POINT ( 'NONE',  ( 15.17214319754859098, -3.426725954212797465, 3.937891351789523320 ) ) ;
#29125=DIRECTION ( 'NONE',  ( 0.000000000000000000, 0.000000000000000000, -1.000000000000000000 ) ) ;
#29127=CARTESIAN_POINT ( 'NONE',  ( -35.85663232820584057, -0.4576450603546987628, 5.200000000000000178 ) ) ;
#29131=ORIENTED_EDGE ( 'NONE', *, *, #13737, .F. ) ;
#29133=DIRECTION ( 'NONE',  ( 0.000000000000000000, -0.000000000000000000, -1.000000000000000000 ) ) ;
#29134=CIRCLE ( 'NONE', #21060, 0.05000000000000012768 ) ;
#29138=DIRECTION ( 'NONE',  ( 0.000000000000000000, 0.000000000000000000, 1.000000000000000000 ) ) ;
#29157=AXIS2_PLACEMENT_3D ( 'NONE', #9355, #30731, #13919 ) ;
#29158=EDGE_LOOP ( 'NONE', ( #13407, #26406, #29684 ) ) ;
#29162=CARTESIAN_POINT ( 'NONE',  ( 50.37722501620130799, 1.384253668070434484, 3.859284659399053741 ) ) ;
#29163=SPHERICAL_SURFACE ( 'NONE', #5561, 0.05000000000000000278 ) ;
#29164=CARTESIAN_POINT ( 'NONE',  ( -53.99999999999997868, 0.000000000000000000, 0.000000000000000000 ) ) ;
#29171=CARTESIAN_POINT ( 'NONE',  ( -36.48174642953001978, -0.4008586329626669387, -5.396496690166842747 ) ) ;
#29172=CARTESIAN_POINT ( 'NONE',  ( -44.49999999999999289, 1.499999999999999556, 4.029888335921975262 ) ) ;
#29175=EDGE_LOOP ( 'NONE', ( #10483, #13137, #11749, #12512 ) ) ;
#29181=DIRECTION ( 'NONE',  ( 0.000000000000000000, 0.000000000000000000, 1.000000000000000000 ) ) ;
#29184=EDGE_CURVE ( 'NONE', #16975, #1787, #9398, .T. ) ;
#29186=CARTESIAN_POINT ( 'NONE',  ( 58.50000000000001421, -0.8000000000000000444, 1.778341924377873751 ) ) ;
#29188=ORIENTED_EDGE ( 'NONE', *, *, #10494, .T. ) ;
#29190=ORIENTED_EDGE ( 'NONE', *, *, #5716, .F. ) ;
#29192=CARTESIAN_POINT ( 'NONE',  ( 16.10667815269232150, 5.187083072802369799, -1.534568794951123083 ) ) ;
#29193=EDGE_LOOP ( 'NONE', ( #8716, #29103, #22308, #6530 ) ) ;
#29195=AXIS2_PLACEMENT_3D ( 'NONE', #25909, #11516, #21194 ) ;
#29198=CARTESIAN_POINT ( 'NONE',  ( 54.50000000000002132, -0.003160834336558230456, 4.277587663180611344 ) ) ;
#29208=CARTESIAN_POINT ( 'NONE',  ( 57.00000000000001421, -0.6999999999999999556, 2.452039967047845437 ) ) ;
#29212=CARTESIAN_POINT ( 'NONE',  ( -36.26369610968609436, -3.231775792180338502, 4.079530926931252743 ) ) ;
#29219=EDGE_CURVE ( 'NONE', #2736, #10297, #7929, .T. ) ;
#29224=DIRECTION ( 'NONE',  ( 0.000000000000000000, 0.000000000000000000, -1.000000000000000000 ) ) ;
#29225=FACE_OUTER_BOUND ( 'NONE', #25592, .T. ) ;
#29243=ADVANCED_FACE ( 'NONE', ( #4957 ), #19175, .T. ) ;
#29244=EDGE_CURVE ( 'NONE', #4962, #30274, #18126, .T. ) ;
#29245=EDGE_CURVE ( 'NONE', #12911, #8533, #5982, .T. ) ;
#29249=PLANE ( 'NONE',  #20544 ) ;
#29253=CARTESIAN_POINT ( 'NONE',  ( -36.89250464418453390, -2.917650619476045204, -4.554978966839832388 ) ) ;
#29256=ADVANCED_FACE ( 'NONE', ( #29329 ), #727, .T. ) ;
#29259=CARTESIAN_POINT ( 'NONE',  ( 15.57907767661750320, 0.5233326973447868236, -5.388419908789428447 ) ) ;
#29261=B_SPLINE_CURVE_WITH_KNOTS ( 'NONE', 3,
 ( #15905, #18303, #1647, #13216, #27944, #30799, #4188, #22899, #13360, #20837, #1346, #10845, #4041, #6260, #30625, #1506 ),
 .UNSPECIFIED., .F., .F.,
 ( 4, 2, 2, 2, 2, 2, 2, 4 ),
 ( 1.734723475976807094E-18, 0.0004351083927046436742, 0.0008702167854092856137, 0.001740433570818568625, 0.002175541963523209155, 0.002610650356227849252, 0.003045758748932490215, 0.003480867141637130312 ),
 .UNSPECIFIED. ) ;
#29262=DIRECTION ( 'NONE',  ( 0.000000000000000000, 0.000000000000000000, -1.000000000000000000 ) ) ;
#29267=CARTESIAN_POINT ( 'NONE',  ( -44.49999999999998579, -1.843099986694572142E-14, 0.000000000000000000 ) ) ;
#29280=EDGE_LOOP ( 'NONE', ( #6524, #8872, #1289, #9655 ) ) ;
#29289=ORIENTED_EDGE ( 'NONE', *, *, #5434, .F. ) ;
#29293=ORIENTED_EDGE ( 'NONE', *, *, #22286, .T. ) ;
#29297=CYLINDRICAL_SURFACE ( 'NONE', #16077, 2.600000000000000089 ) ;
#29299=ORIENTED_EDGE ( 'NONE', *, *, #30878, .T. ) ;
#29300=CARTESIAN_POINT ( 'NONE',  ( 48.50000000000002132, -1.426739617975173013, 3.843750000000023093 ) ) ;
#29301=ORIENTED_EDGE ( 'NONE', *, *, #29808, .F. ) ;
#29305=VERTEX_POINT ( 'NONE', #14905 ) ;
#29307=CIRCLE ( 'NONE', #18697, 4.375000000000000000 ) ;
#29310=AXIS2_PLACEMENT_3D ( 'NONE', #8190, #3454, #20713 ) ;
#29314=CARTESIAN_POINT ( 'NONE',  ( 50.30000000000001847, 1.426739617975221641, 3.843750000000023093 ) ) ;
#29315=CARTESIAN_POINT ( 'NONE',  ( -54.48531357662248809, -1.514292094527452948, 3.309285685900293039 ) ) ;
#29316=ADVANCED_FACE ( 'NONE', ( #29466 ), #30665, .T. ) ;
#29318=AXIS2_PLACEMENT_3D ( 'NONE', #30271, #15860, #16022 ) ;
#29320=CARTESIAN_POINT ( 'NONE',  ( -35.85663232820579793, -1.123735532908308965, -5.289358697221545391 ) ) ;
#29322=CARTESIAN_POINT ( 'NONE',  ( 48.49151045397272952, 1.391941090707534689, -3.850000000000023181 ) ) ;
#29327=DIRECTION ( 'NONE',  ( 1.000000000000000000, 2.586136946169074517E-16, -0.000000000000000000 ) ) ;
#29328=CARTESIAN_POINT ( 'NONE',  ( -36.92398358572908990, -5.053896291911982530, -1.944420249220666586 ) ) ;
#29329=FACE_OUTER_BOUND ( 'NONE', #3655, .T. ) ;
#29332=ORIENTED_EDGE ( 'NONE', *, *, #28568, .T. ) ;
#29335=CARTESIAN_POINT ( 'NONE',  ( 15.71019289815287934, -5.349060760730925068, 0.7993770229878324196 ) ) ;
#29338=ORIENTED_EDGE ( 'NONE', *, *, #11047, .F. ) ;
#29341=CIRCLE ( 'NONE', #26814, 4.375000000000000000 ) ;
#29342=CARTESIAN_POINT ( 'NONE',  ( 58.50000000000001421, 0.8156862745098042433, -2.468735688885369317 ) ) ;
#29345=DIRECTION ( 'NONE',  ( 0.000000000000000000, 1.000000000000000000, 0.000000000000000000 ) ) ;
#29348=EDGE_LOOP ( 'NONE', ( #10062, #2144, #29512 ) ) ;
#29352=CARTESIAN_POINT ( 'NONE',  ( -54.45981523601835761, -1.500740478982482973, 4.030402907299741599 ) ) ;
#29354=CARTESIAN_POINT ( 'NONE',  ( 47.00000000000002132, 1.734723475976807094E-15, 0.000000000000000000 ) ) ;
#29356=CARTESIAN_POINT ( 'NONE',  ( 57.01549179440438309, 0.7366256376427431363, 2.429951667075468613 ) ) ;
#29357=DIRECTION ( 'NONE',  ( 0.000000000000000000, 1.000000000000000000, 0.000000000000000000 ) ) ;
#29359=CARTESIAN_POINT ( 'NONE',  ( 50.31874172786521626, -1.426739617975169905, -3.843750000000023537 ) ) ;
#29366=DIRECTION ( 'NONE',  ( 0.000000000000000000, 0.000000000000000000, -1.000000000000000000 ) ) ;
#29368=CARTESIAN_POINT ( 'NONE',  ( 15.03925126672132784, 5.377732432866636714, 0.5657657256216092057 ) ) ;
#29371=EDGE_CURVE ( 'NONE', #25975, #23625, #10955, .T. ) ;
#29382=CARTESIAN_POINT ( 'NONE',  ( 57.02942257420237837, 0.7458803891215903814, 1.782029179052657009 ) ) ;
#29383=CARTESIAN_POINT ( 'NONE',  ( 15.45522337368516119, -4.885888067249546829, -1.790336215468742997 ) ) ;
#29386=EDGE_CURVE ( 'NONE', #22370, #15602, #6198, .T. ) ;
#29388=CARTESIAN_POINT ( 'NONE',  ( 50.30000000000001847, 1.409901620910219311, -3.850000000000021849 ) ) ;
#29389=CARTESIAN_POINT ( 'NONE',  ( 15.03925126672133139, -4.683225679163337318, -2.703237727951242508 ) ) ;
#29394=CARTESIAN_POINT ( 'NONE',  ( -36.22909104983324369, -2.595074437875156903, -4.757608386864808914 ) ) ;
#29397=CARTESIAN_POINT ( 'NONE',  ( 50.42181344116571751, 1.309616516426969302, -3.885368734293527471 ) ) ;
#29400=CARTESIAN_POINT ( 'NONE',  ( -35.85663232820584057, 0.4576450603546987628, 5.200000000000000178 ) ) ;
#29401=CARTESIAN_POINT ( 'NONE',  ( -36.89017861347080185, -5.034707333629141246, 1.977875755500610122 ) ) ;
#29402=CARTESIAN_POINT ( 'NONE',  ( 48.30260100412290569, -0.9326869175216284669, -3.995127421239667687 ) ) ;
#29415=CARTESIAN_POINT ( 'NONE',  ( 57.00357781822870606, -0.7683521053270409018, 1.737709711729638729 ) ) ;
#29418=CYLINDRICAL_SURFACE ( 'NONE', #13686, 0.09999999999999982514 ) ;
#29419=FACE_OUTER_BOUND ( 'NONE', #15718, .T. ) ;
#29420=CARTESIAN_POINT ( 'NONE',  ( 16.08093158123429589, -0.2888463313200277383, 5.401384060636566176 ) ) ;
#29429=ORIENTED_EDGE ( 'NONE', *, *, #813, .F. ) ;
#29433=CARTESIAN_POINT ( 'NONE',  ( 15.74652664997095286, -3.345968172200381119, -4.250076229745499923 ) ) ;
#29437=VERTEX_POINT ( 'NONE', #7146 ) ;
#29438=DIRECTION ( 'NONE',  ( 1.000000000000000000, -0.000000000000000000, -0.000000000000000000 ) ) ;
#29441=ORIENTED_EDGE ( 'NONE', *, *, #8319, .T. ) ;
#29443=CARTESIAN_POINT ( 'NONE',  ( 50.40000000000001990, 0.6304760106459513791, 3.950000000000022826 ) ) ;
#29445=CARTESIAN_POINT ( 'NONE',  ( -35.85663232820578372, -5.377732432866659806, -0.5657657256215627983 ) ) ;
#29452=CARTESIAN_POINT ( 'NONE',  ( 48.42176022524417789, -1.183413901109541477, -3.885761703493072261 ) ) ;
#29453=CARTESIAN_POINT ( 'NONE',  ( -54.46926330052497178, -1.503605180550109388, 3.302415457191588910 ) ) ;
#29461=CARTESIAN_POINT ( 'NONE',  ( 15.49676243306307377, 4.963067629822636384, -1.552801941062253999 ) ) ;
#29464=CARTESIAN_POINT ( 'NONE',  ( 50.38490132722630932, -1.114141714781589521, -3.896173399896524003 ) ) ;
#29466=FACE_OUTER_BOUND ( 'NONE', #16821, .T. ) ;
#29471=EDGE_CURVE ( 'NONE', #26348, #19839, #19069, .T. ) ;
#29472=EDGE_LOOP ( 'NONE', ( #9668, #11477, #11101, #2002 ) ) ;
#29476=CARTESIAN_POINT ( 'NONE',  ( 15.44631504820157097, 5.012449653004692252, 1.400819699606158819 ) ) ;
#29480=ORIENTED_EDGE ( 'NONE', *, *, #7850, .F. ) ;
#29481=DIRECTION ( 'NONE',  ( 0.000000000000000000, 0.000000000000000000, -1.000000000000000000 ) ) ;
#29482=EDGE_LOOP ( 'NONE', ( #29710, #30452, #10067, #16609 ) ) ;
#29485=CARTESIAN_POINT ( 'NONE',  ( 48.40000000000001990, -4.899999999999999467, 3.850000000000022737 ) ) ;
#29488=CARTESIAN_POINT ( 'NONE',  ( 51.71101551635177884, -4.179189514726506793, -1.000000000000000000 ) ) ;
#29489=CARTESIAN_POINT ( 'NONE',  ( -54.49998548284560940, -1.548795215916124457, 4.063650232134933482 ) ) ;
#29491=CYLINDRICAL_SURFACE ( 'NONE', #25576, 1.000000000000000000 ) ;
#29493=B_SPLINE_CURVE_WITH_KNOTS ( 'NONE', 3,
 ( #28537, #4305, #18584, #11442, #9387, #16514, #26169, #25697, #21288, #18422, #6540, #28059, #6380, #4476, #11271, #23802 ),
 .UNSPECIFIED., .F., .F.,
 ( 4, 2, 2, 2, 2, 2, 2, 4 ),
 ( 0.000000000000000000, 0.0004351083927046389579, 0.0008702167854092779159, 0.001740433570818555615, 0.002175541963523194844, 0.002610650356227833639, 0.003045758748932472868, 0.003480867141637111663 ),
 .UNSPECIFIED. ) ;
#29494=CARTESIAN_POINT ( 'NONE',  ( -36.30347965937246357, -2.964363692626382552, 4.273817190665925914 ) ) ;
#29496=ADVANCED_FACE ( 'NONE', ( #21564 ), #16958, .T. ) ;
#29497=CARTESIAN_POINT ( 'NONE',  ( 47.00000000000002132, -3.726179070414207928, -1.100000000000000089 ) ) ;
#29498=FACE_OUTER_BOUND ( 'NONE', #30822, .T. ) ;
#29499=CARTESIAN_POINT ( 'NONE',  ( -54.49999999999997868, 1.549582583372307809, -3.331868970650947226 ) ) ;
#29501=VECTOR ( 'NONE', #9285, 1000.000000000000000 ) ;
#29504=ADVANCED_FACE ( 'NONE', ( #16658 ), #938, .T. ) ;
#29509=CARTESIAN_POINT ( 'NONE',  ( 15.70940947763170215, 5.349174094756180331, 0.7986533162261519880 ) ) ;
#29510=DIRECTION ( 'NONE',  ( 1.000000000000000000, 0.000000000000000000, 0.000000000000000000 ) ) ;
#29512=ORIENTED_EDGE ( 'NONE', *, *, #20410, .T. ) ;
#29520=CARTESIAN_POINT ( 'NONE',  ( 15.03925126672132961, 4.018128179617504792, 3.618665901676689778 ) ) ;
#29523=CARTESIAN_POINT ( 'NONE',  ( 15.49702763512084225, -4.962395293451320022, -1.554871187131938726 ) ) ;
#29524=CIRCLE ( 'NONE', #18430, 0.09999999999999982514 ) ;
#29528=DIRECTION ( 'NONE',  ( -1.000000000000000000, 0.000000000000000000, 0.000000000000000000 ) ) ;
#29531=EDGE_CURVE ( 'NONE', #8120, #24812, #25615, .T. ) ;
#29532=DIRECTION ( 'NONE',  ( 1.000000000000000000, 0.000000000000000000, 0.000000000000000000 ) ) ;
#29542=ORIENTED_EDGE ( 'NONE', *, *, #21332, .F. ) ;
#29545=EDGE_CURVE ( 'NONE', #24288, #30697, #12372, .T. ) ;
#29554=FACE_OUTER_BOUND ( 'NONE', #21787, .T. ) ;
#29555=EDGE_LOOP ( 'NONE', ( #12140, #7603, #871, #29131 ) ) ;
#29559=ORIENTED_EDGE ( 'NONE', *, *, #9122, .F. ) ;
#29562=DIRECTION ( 'NONE',  ( 1.000000000000000000, 0.000000000000000000, 0.000000000000000000 ) ) ;
#29569=CARTESIAN_POINT ( 'NONE',  ( 15.48686146417447240, 3.146183597690325850, 4.141717300434360816 ) ) ;
#29571=ADVANCED_FACE ( 'NONE', ( #9004 ), #1946, .T. ) ;
#29585=CARTESIAN_POINT ( 'NONE',  ( 15.67083574136752944, -3.495540671458118531, -4.131527132740935748 ) ) ;
#29588=AXIS2_PLACEMENT_3D ( 'NONE', #25812, #8700, #2061 ) ;
#29597=CARTESIAN_POINT ( 'NONE',  ( -36.80043232705877898, -5.283830060792408467, -1.151642405604301089 ) ) ;
#29607=CARTESIAN_POINT ( 'NONE',  ( 15.03925126672122836, -1.123735532908289647, 5.289358697221546279 ) ) ;
#29609=AXIS2_PLACEMENT_3D ( 'NONE', #24979, #20271, #3472 ) ;
#29615=CARTESIAN_POINT ( 'NONE',  ( -36.27260443516959043, -0.1928884786869198564, -5.200000000471145079 ) ) ;
#29616=AXIS2_PLACEMENT_3D ( 'NONE', #25306, #22800, #15181 ) ;
#29618=CARTESIAN_POINT ( 'NONE',  ( 48.40000000000002700, 0.7618928438397208902, -3.939512004971702730 ) ) ;
#29624=CARTESIAN_POINT ( 'NONE',  ( 50.46980263351819929, -1.141995257496313476, -3.938405479918980490 ) ) ;
#29627=CARTESIAN_POINT ( 'NONE',  ( 15.68751737981905947, 3.461789369942972705, -4.158232265984232789 ) ) ;
#29632=CARTESIAN_POINT ( 'NONE',  ( 47.02986096046866749, -4.166824046520646974, 1.027859347733066198 ) ) ;
#29635=ORIENTED_EDGE ( 'NONE', *, *, #15229, .T. ) ;
#29637=ORIENTED_EDGE ( 'NONE', *, *, #5495, .T. ) ;
#29639=TOROIDAL_SURFACE ( 'NONE', #10924, 1.949999999999999956, 0.05000000000000000278 ) ;
#29640=CARTESIAN_POINT ( 'NONE',  ( 15.03925126672132784, 5.086913985776138070, 1.171642053949162543 ) ) ;
#29641=ORIENTED_EDGE ( 'NONE', *, *, #7870, .T. ) ;
#29652=TOROIDAL_SURFACE ( 'NONE', #23591, 1.949999999999999956, 0.05000000000000000278 ) ;
#29668=CARTESIAN_POINT ( 'NONE',  ( -54.48531357662248809, 1.514292094527452504, -3.309285685900293927 ) ) ;
#29673=AXIS2_PLACEMENT_3D ( 'NONE', #751, #10412, #22159 ) ;
#29682=CARTESIAN_POINT ( 'NONE',  ( 15.18463186935387377, 4.683225679163116162, 2.703237727951770086 ) ) ;
#29684=ORIENTED_EDGE ( 'NONE', *, *, #27266, .T. ) ;
#29689=VERTEX_POINT ( 'NONE', #21376 ) ;
#29692=CARTESIAN_POINT ( 'NONE',  ( 51.80000000000001847, 1.734723475976807094E-15, 0.000000000000000000 ) ) ;
#29694=AXIS2_PLACEMENT_3D ( 'NONE', #9575, #30333, #8638 ) ;
#29695=CARTESIAN_POINT ( 'NONE',  ( 15.29449157529455938, -5.068523420888935149, -1.228242390833362618 ) ) ;
#29699=TOROIDAL_SURFACE ( 'NONE', #4416, 3.299999999999999822, 0.1000000000000000056 ) ;
#29701=CARTESIAN_POINT ( 'NONE',  ( 48.48449022203101322, 1.386241252175322014, 3.851058308531627450 ) ) ;
#29710=ORIENTED_EDGE ( 'NONE', *, *, #31306, .T. ) ;
#29714=CARTESIAN_POINT ( 'NONE',  ( -36.43290890416665206, -2.776541361170759892, -4.646985486732256199 ) ) ;
#29719=VECTOR ( 'NONE', #4917, 1000.000000000000000 ) ;
#29720=ORIENTED_EDGE ( 'NONE', *, *, #27272, .T. ) ;
#29723=CARTESIAN_POINT ( 'NONE',  ( 48.30000000000003268, -0.7901969350669647563, -4.025772098418840983 ) ) ;
#29724=DIRECTION ( 'NONE',  ( -0.000000000000000000, -0.000000000000000000, 1.000000000000000000 ) ) ;
#29734=EDGE_CURVE ( 'NONE', #518, #12299, #6422, .T. ) ;
#29737=DIRECTION ( 'NONE',  ( 0.000000000000000000, 0.000000000000000000, -1.000000000000000000 ) ) ;
#29743=CARTESIAN_POINT ( 'NONE',  ( 15.22780280894163241, 2.525801254963248699, 4.794550361020370133 ) ) ;
#29746=EDGE_CURVE ( 'NONE', #19238, #11901, #2567, .T. ) ;
#29749=CARTESIAN_POINT ( 'NONE',  ( -36.22818246778845719, 4.895960019030868082, -2.323379425334441084 ) ) ;
#29755=CARTESIAN_POINT ( 'NONE',  ( 50.30000000000001847, -1.426739617975173013, 3.843750000000023093 ) ) ;
#29756=CARTESIAN_POINT ( 'NONE',  ( 57.03907689491666844, 0.7490795634100378964, -2.421870079683545285 ) ) ;
#29757=DIRECTION ( 'NONE',  ( -0.000000000000000000, -0.000000000000000000, 1.000000000000000000 ) ) ;
#29762=AXIS2_PLACEMENT_3D ( 'NONE', #14717, #24379, #12195 ) ;
#29766=CARTESIAN_POINT ( 'NONE',  ( 51.76087627324522344, -4.170474612306438011, 1.019817338724548383 ) ) ;
#29769=DIRECTION ( 'NONE',  ( 1.000000000000000000, 0.000000000000000000, -0.000000000000000000 ) ) ;
#29772=ORIENTED_EDGE ( 'NONE', *, *, #29901, .F. ) ;
#29776=FACE_OUTER_BOUND ( 'NONE', #11890, .T. ) ;
#29777=ADVANCED_FACE ( 'NONE', ( #918 ), #17373, .T. ) ;
#29780=AXIS2_PLACEMENT_3D ( 'NONE', #26804, #5253, #24421 ) ;
#29789=LINE ( 'NONE', #8104, #25053 ) ;
#29792=CARTESIAN_POINT ( 'NONE',  ( 15.48609859788814980, 3.148602930107248898, -4.139959549308847464 ) ) ;
#29794=CARTESIAN_POINT ( 'NONE',  ( 57.03821272586434787, 0.7500000328843418052, 2.490438846756156899 ) ) ;
#29800=CARTESIAN_POINT ( 'NONE',  ( 16.10667815269233216, -5.187083072802361805, 1.534568794951160609 ) ) ;
#29804=CARTESIAN_POINT ( 'NONE',  ( 15.48686146417451326, 4.979756346315124205, 1.501439362221289597 ) ) ;
#29806=STYLED_ITEM ( 'NONE', ( #19039 ), #12719 ) ;
#29808=EDGE_CURVE ( 'NONE', #23361, #26099, #12302, .T. ) ;
#29816=ORIENTED_EDGE ( 'NONE', *, *, #3407, .T. ) ;
#29821=FACE_OUTER_BOUND ( 'NONE', #18617, .T. ) ;
#29822=CARTESIAN_POINT ( 'NONE',  ( 15.03925126672132961, -3.426725943139564912, 3.937891353488729429 ) ) ;
#29833=CARTESIAN_POINT ( 'NONE',  ( -54.49983832461118283, 1.542920080254278181, 3.327619142904491234 ) ) ;
#29841=ORIENTED_EDGE ( 'NONE', *, *, #324, .F. ) ;
#29852=CARTESIAN_POINT ( 'NONE',  ( 16.10705563471231372, -5.191204783933229372, -1.522159526382844907 ) ) ;
#29856=AXIS2_PLACEMENT_3D ( 'NONE', #9804, #4890, #2198 ) ;
#29864=( BOUNDED_SURFACE ( )  B_SPLINE_SURFACE ( 3, 2, ( 
 ( #8902, #18899, #19225 ),
 ( #2098, #13795, #16206 ),
 ( #28542, #20957, #23658 ),
 ( #6852, #23807, #30589 ),
 ( #18589, #6544, #21438 ),
 ( #28866, #25854, #1951 ),
 ( #23478, #19061, #30765 ),
 ( #1772, #28715, #5103 ),
 ( #7776, #22057, #29461 ),
 ( #5413, #652, #353 ),
 ( #17152, #22216, #19980 ),
 ( #12230, #26646, #16994 ),
 ( #24114, #19688, #24415 ),
 ( #14754, #17444, #9854 ),
 ( #17294, #21913, #505 ),
 ( #2724, #12368, #16840 ) ),
 .UNSPECIFIED., .F., .F., .F. ) 
 B_SPLINE_SURFACE_WITH_KNOTS ( ( 4, 2, 2, 2, 2, 2, 2, 4 ),
 ( 3, 3 ),
 ( 0.001780502285214183430, 0.002558945925323759425, 0.002753556835351153587, 0.002948167745378547314, 0.003337389565433335203, 0.003726611385488123093, 0.004115833205542910982, 0.004894276845652486760 ),
 ( 0.000000000000000000, 1.000000000000000000 ),
 .UNSPECIFIED. ) 
 GEOMETRIC_REPRESENTATION_ITEM ( )  RATIONAL_B_SPLINE_SURFACE ( (
 ( 1.000000000000000000, 0.9418517008537252710, 1.000000000000000000),
 ( 1.000000000000000000, 0.9417987965885095125, 1.000000000000000000),
 ( 1.000000000000000000, 0.9418198861734097260, 1.000000000000000000),
 ( 1.000000000000000000, 0.9434060303845585027, 1.000000000000000000),
 ( 1.000000000000000000, 0.9437939819948245601, 1.000000000000000000),
 ( 1.000000000000000000, 0.9445989566712741370, 1.000000000000000000),
 ( 1.000000000000000000, 0.9450169930050026368, 1.000000000000000000),
 ( 1.000000000000000000, 0.9461610507673267056, 1.000000000000000000),
 ( 1.000000000000000000, 0.9467217966427221576, 1.000000000000000000),
 ( 1.000000000000000000, 0.9467345476124371384, 1.000000000000000000),
 ( 1.000000000000000000, 0.9461964028052947118, 1.000000000000000000),
 ( 1.000000000000000000, 0.9446801822473851473, 1.000000000000000000),
 ( 1.000000000000000000, 0.9437582546536329442, 1.000000000000000000),
 ( 1.000000000000000000, 0.9418129560296130132, 1.000000000000000000),
 ( 1.000000000000000000, 0.9418016889777165446, 1.000000000000000000),
 ( 1.000000000000000000, 0.9418517008537247159, 1.000000000000000000) ) ) 
 REPRESENTATION_ITEM ( '' )  SURFACE ( )  );
#29873=EDGE_LOOP ( 'NONE', ( #6836, #27396, #28761, #15429 ) ) ;
#29876=CIRCLE ( 'NONE', #28369, 0.05000000000000008604 ) ;
#29880=CARTESIAN_POINT ( 'NONE',  ( -35.85663232820584057, -0.9159215771353976798, -4.311190327365980401 ) ) ;
#29881=AXIS2_PLACEMENT_3D ( 'NONE', #10420, #5830, #22165 ) ;
#29884=ORIENTED_EDGE ( 'NONE', *, *, #4116, .T. ) ;
#29886=FACE_OUTER_BOUND ( 'NONE', #13228, .T. ) ;
#29887=DIRECTION ( 'NONE',  ( 0.000000000000000000, 0.000000000000000000, -1.000000000000000000 ) ) ;
#29888=VERTEX_POINT ( 'NONE', #8500 ) ;
#29892=CARTESIAN_POINT ( 'NONE',  ( -36.92398358572908990, -3.410993390446888096, 4.205682099886847602 ) ) ;
#29898=CARTESIAN_POINT ( 'NONE',  ( 15.95705409078442294, -2.672993279333548688, 4.702725322014869924 ) ) ;
#29899=DIRECTION ( 'NONE',  ( 0.000000000000000000, 0.4102564102564100201, -0.9119702176296790030 ) ) ;
#29901=EDGE_CURVE ( 'NONE', #22384, #27011, #5425, .T. ) ;
#29906=CARTESIAN_POINT ( 'NONE',  ( -35.85663232820584057, -4.804073783693452171, -2.042134687550364092 ) ) ;
#29917=VERTEX_POINT ( 'NONE', #3903 ) ;
#29929=CARTESIAN_POINT ( 'NONE',  ( 47.00970077834632121, -4.153760649298012808, -1.055564289358534635 ) ) ;
#29931=CARTESIAN_POINT ( 'NONE',  ( 48.43418025728714582, -1.399739523915389583, -3.853780793998481169 ) ) ;
#29933=CARTESIAN_POINT ( 'NONE',  ( 16.10624235918717417, -0.1627367787821556444, 5.407318510437581160 ) ) ;
#29934=CARTESIAN_POINT ( 'NONE',  ( 57.04707324256202128, -0.7500000000000492939, -2.421260002560643443 ) ) ;
#29940=CARTESIAN_POINT ( 'NONE',  ( -45.15971931043468146, -4.700000000000000178, 5.808909232612072777E-16 ) ) ;
#29945=CARTESIAN_POINT ( 'NONE',  ( -36.89831264271880684, 2.941172302009069206, -4.539591111929616396 ) ) ;
#29949=DIRECTION ( 'NONE',  ( 1.000000000000000000, 0.000000000000000000, 0.000000000000000000 ) ) ;
#29953=ORIENTED_EDGE ( 'NONE', *, *, #12892, .F. ) ;
#29958=CARTESIAN_POINT ( 'NONE',  ( 16.10667815269233216, 3.294441450831234075, -4.290383166762102185 ) ) ;
#29959=DIRECTION ( 'NONE',  ( 0.000000000000000000, 1.000000000000000000, 0.000000000000000000 ) ) ;
#29964=CARTESIAN_POINT ( 'NONE',  ( 57.00357781822870606, 0.7683521053270409018, -1.737709711729638729 ) ) ;
#29967=VERTEX_POINT ( 'NONE', #8789 ) ;
#29970=CARTESIAN_POINT ( 'NONE',  ( 51.90000000000001279, 1.734723475976807094E-15, 0.000000000000000000 ) ) ;
#29974=CARTESIAN_POINT ( 'NONE',  ( -54.44999999999997442, 0.000000000000000000, 4.299999999999998046 ) ) ;
#29978=CARTESIAN_POINT ( 'NONE',  ( -54.48833221701376317, 1.517896399908648108, -3.311598511235000153 ) ) ;
#29979=CARTESIAN_POINT ( 'NONE',  ( 48.33000880451179881, -1.140870969100513888, 3.938727831757874664 ) ) ;
#29980=EDGE_CURVE ( 'NONE', #23272, #29040, #19275, .T. ) ;
#29989=CARTESIAN_POINT ( 'NONE',  ( 47.00000000000002132, -3.726179070414207928, -1.710435481158852467 ) ) ;
#30015=ORIENTED_EDGE ( 'NONE', *, *, #6217, .T. ) ;
#30017=ORIENTED_EDGE ( 'NONE', *, *, #19680, .F. ) ;
#30018=CARTESIAN_POINT ( 'NONE',  ( 15.44631504820156209, -0.2166734227622303666, -5.199999998324986272 ) ) ;
#30022=ORIENTED_EDGE ( 'NONE', *, *, #21112, .T. ) ;
#30023=DIRECTION ( 'NONE',  ( 1.000000000000000000, 0.000000000000000000, -0.000000000000000000 ) ) ;
#30032=CARTESIAN_POINT ( 'NONE',  ( -35.85663232820584057, -4.804073783693452171, -2.042134687550364092 ) ) ;
#30040=CARTESIAN_POINT ( 'NONE',  ( 15.03925126672132961, -2.199885893005964377, 4.939696249117675464 ) ) ;
#30045=CYLINDRICAL_SURFACE ( 'NONE', #17386, 1.000000000000000000 ) ;
#30052=ORIENTED_EDGE ( 'NONE', *, *, #14039, .T. ) ;
#30055=CARTESIAN_POINT ( 'NONE',  ( 48.37884656342667711, 0.9200365198983960768, 3.998286360709680576 ) ) ;
#30057=ORIENTED_EDGE ( 'NONE', *, *, #15952, .T. ) ;
#30058=VERTEX_POINT ( 'NONE', #9617 ) ;
#30062=ORIENTED_EDGE ( 'NONE', *, *, #16853, .T. ) ;
#30064=DIRECTION ( 'NONE',  ( -1.000000000000000000, -0.000000000000000000, -0.000000000000000000 ) ) ;
#30068=CARTESIAN_POINT ( 'NONE',  ( -36.11187263677958015, -4.822464347459074929, -1.985534350301396911 ) ) ;
#30069=CARTESIAN_POINT ( 'NONE',  ( 46.90000000000001279, 2.258259982612300799E-15, -4.275000000000000355 ) ) ;
#30072=CARTESIAN_POINT ( 'NONE',  ( 47.02303712724481244, -4.162962223351915902, -1.036150832289954193 ) ) ;
#30082=AXIS2_PLACEMENT_3D ( 'NONE', #5879, #10929, #8556 ) ;
#30089=DIRECTION ( 'NONE',  ( 0.000000000000000000, 0.000000000000000000, -1.000000000000000000 ) ) ;
#30099=DIRECTION ( 'NONE',  ( 0.000000000000000000, 0.000000000000000000, -1.000000000000000000 ) ) ;
#30115=CARTESIAN_POINT ( 'NONE',  ( 56.95000000000001705, -0.6917305289283675052, -1.769637370168020141 ) ) ;
#30116=AXIS2_PLACEMENT_3D ( 'NONE', #941, #3619, #5837 ) ;
#30119=EDGE_CURVE ( 'NONE', #618, #1564, #12036, .T. ) ;
#30122=CARTESIAN_POINT ( 'NONE',  ( -35.85663232820584057, 4.817150320979497913, 2.203324261490556157 ) ) ;
#30124=EDGE_CURVE ( 'NONE', #3567, #30652, #18391, .T. ) ;
#30129=CIRCLE ( 'NONE', #15474, 4.100000000000022737 ) ;
#30135=ORIENTED_EDGE ( 'NONE', *, *, #11641, .F. ) ;
#30136=CIRCLE ( 'NONE', #15990, 4.384222560975607585 ) ;
#30138=PRESENTATION_STYLE_ASSIGNMENT (( #20815 ) ) ;
#30142=ORIENTED_EDGE ( 'NONE', *, *, #29734, .F. ) ;
#30148=AXIS2_PLACEMENT_3D ( 'NONE', #17916, #20772, #13150 ) ;
#30152=AXIS2_PLACEMENT_3D ( 'NONE', #14614, #2107, #24280 ) ;
#30153=ORIENTED_EDGE ( 'NONE', *, *, #19523, .F. ) ;
#30154=DIRECTION ( 'NONE',  ( 0.000000000000000000, 1.000000000000000000, 0.000000000000000000 ) ) ;
#30155=EDGE_CURVE ( 'NONE', #21818, #29917, #23655, .T. ) ;
#30157=B_SPLINE_CURVE_WITH_KNOTS ( 'NONE', 3,
 ( #26077, #21205, #11528, #9475, #25921, #21032, #4226, #11348, #23556, #1856, #4391, #30837, #18816, #21360, #14038, #3400 ),
 .UNSPECIFIED., .F., .F.,
 ( 4, 2, 2, 2, 2, 2, 2, 4 ),
 ( 2.168404344971008868E-19, 0.0007944403960943761467, 0.001191660594141564274, 0.001390270693165157959, 0.001489575742676953717, 0.001539228267432849644, 0.001564054529810800318, 0.001588880792188750992 ),
 .UNSPECIFIED. ) ;
#30158=FACE_OUTER_BOUND ( 'NONE', #6775, .T. ) ;
#30165=VECTOR ( 'NONE', #9860, 1000.000000000000000 ) ;
#30177=CIRCLE ( 'NONE', #15012, 2.600000000000000089 ) ;
#30180=EDGE_LOOP ( 'NONE', ( #11420, #20595, #15632, #1790 ) ) ;
#30187=AXIS2_PLACEMENT_3D ( 'NONE', #21737, #9691, #7298 ) ;
#30188=VERTEX_POINT ( 'NONE', #27311 ) ;
#30191=CARTESIAN_POINT ( 'NONE',  ( 57.03513260258041839, -0.7477432062408043700, -1.780365573899210574 ) ) ;
#30195=DIRECTION ( 'NONE',  ( 1.000000000000000000, -0.000000000000000000, -0.000000000000000000 ) ) ;
#30197=CARTESIAN_POINT ( 'NONE',  ( -36.58413561666694847, 5.174628573245025898, -1.572974725650795991 ) ) ;
#30201=AXIS2_PLACEMENT_3D ( 'NONE', #140, #17547, #746 ) ;
#30205=EDGE_CURVE ( 'NONE', #15656, #25275, #3425, .T. ) ;
#30209=CARTESIAN_POINT ( 'NONE',  ( 15.49702763512084402, 3.100731772197714342, 4.174739983989972814 ) ) ;
#30210=AXIS2_PLACEMENT_3D ( 'NONE', #22783, #30494, #15646 ) ;
#30212=SPHERICAL_SURFACE ( 'NONE', #30116, 0.05000000000000000278 ) ;
#30214=CIRCLE ( 'NONE', #11011, 1.000000000000000000 ) ;
#30219=CARTESIAN_POINT ( 'NONE',  ( 48.46694841591348535, 1.365427245289844826, -3.854926352964885172 ) ) ;
#30229=FACE_BOUND ( 'NONE', #7449, .T. ) ;
#30231=CARTESIAN_POINT ( 'NONE',  ( 56.95000000000001705, 0.6820512820512819596, -1.773360101234998210 ) ) ;
#30239=( BOUNDED_SURFACE ( )  B_SPLINE_SURFACE ( 3, 2, ( 
 ( #24733, #7498, #10169 ),
 ( #26946, #19838, #12689 ),
 ( #8257, #29794, #6056 ),
 ( #3358, #8566, #22844 ) ),
 .UNSPECIFIED., .F., .F., .F. ) 
 B_SPLINE_SURFACE_WITH_KNOTS ( ( 4, 4 ),
 ( 3, 3 ),
 ( 7.146054570217184225E-05, 0.0002313930902385299038 ),
 ( 0.000000000000000000, 1.000000000000000000 ),
 .UNSPECIFIED. ) 
 GEOMETRIC_REPRESENTATION_ITEM ( )  RATIONAL_B_SPLINE_SURFACE ( (
 ( 1.000000000000000000, 0.7071067811864972796, 1.000000000000000000),
 ( 1.000000000000000000, 0.6583912147046423469, 1.000000000000000000),
 ( 1.000000000000000000, 0.5850387677749523396, 1.000000000000000000),
 ( 1.000000000000000000, 0.5857791861290068125, 1.000000000000000000) ) ) 
 REPRESENTATION_ITEM ( '' )  SURFACE ( )  );
#30243=FACE_OUTER_BOUND ( 'NONE', #30413, .T. ) ;
#30245=CARTESIAN_POINT ( 'NONE',  ( 15.41586008885035142, 0.2667568399900541176, 5.200000000294856761 ) ) ;
#30250=TOROIDAL_SURFACE ( 'NONE', #17639, 1.949999999999999956, 0.05000000000000000278 ) ;
#30251=AXIS2_PLACEMENT_3D ( 'NONE', #26959, #4973, #12552 ) ;
#30257=FACE_OUTER_BOUND ( 'NONE', #16814, .T. ) ;
#30258=CARTESIAN_POINT ( 'NONE',  ( 15.03925126672132961, -1.793057972834775970, -4.026191436120402756 ) ) ;
#30260=CARTESIAN_POINT ( 'NONE',  ( 47.10000000000002274, -4.179189514726508570, 0.8999999999999996891 ) ) ;
#30261=EDGE_LOOP ( 'NONE', ( #18399, #24856 ) ) ;
#30270=ORIENTED_EDGE ( 'NONE', *, *, #3503, .T. ) ;
#30271=CARTESIAN_POINT ( 'NONE',  ( -35.85663232820584767, 3.817150320980632561, 2.203324261490556157 ) ) ;
#30274=VERTEX_POINT ( 'NONE', #30231 ) ;
#30283=ADVANCED_FACE ( 'NONE', ( #8831 ), #15968, .T. ) ;
#30284=DIRECTION ( 'NONE',  ( 0.000000000000000000, -1.000000000000000000, 0.000000000000000000 ) ) ;
#30291=LINE ( 'NONE', #12725, #11988 ) ;
#30294=CARTESIAN_POINT ( 'NONE',  ( 15.03925126672133139, -4.804073783693452171, 2.042134687550334338 ) ) ;
#30306=EDGE_LOOP ( 'NONE', ( #7741, #29429, #23599, #24027 ) ) ;
#30312=DIRECTION ( 'NONE',  ( 1.000000000000000000, 0.000000000000000000, 0.000000000000000000 ) ) ;
#30313=ADVANCED_FACE ( 'NONE', ( #23425 ), #19615, .T. ) ;
#30315=VERTEX_POINT ( 'NONE', #6483 ) ;
#30316=CARTESIAN_POINT ( 'NONE',  ( 47.10000000000002274, -4.259946800035237402, -1.000000000000000222 ) ) ;
#30324=CARTESIAN_POINT ( 'NONE',  ( 57.04171473382086077, 0.7493275531345221507, -1.778946371510476077 ) ) ;
#30327=AXIS2_PLACEMENT_3D ( 'NONE', #7195, #26669, #26195 ) ;
#30329=DIRECTION ( 'NONE',  ( 0.000000000000000000, -1.000000000000000000, 0.000000000000000000 ) ) ;
#30331=EDGE_LOOP ( 'NONE', ( #26192, #15427, #28685, #8157 ) ) ;
#30333=DIRECTION ( 'NONE',  ( -1.000000000000000000, -0.000000000000000000, -0.000000000000000000 ) ) ;
#30342=LINE ( 'NONE', #15785, #22753 ) ;
#30343=VERTEX_POINT ( 'NONE', #30380 ) ;
#30346=ORIENTED_EDGE ( 'NONE', *, *, #29219, .T. ) ;
#30349=CARTESIAN_POINT ( 'NONE',  ( 48.30000000000001847, 2.428612866367529932E-14, 0.000000000000000000 ) ) ;
#30352=CARTESIAN_POINT ( 'NONE',  ( -36.11780688638203429, 5.377732434016818885, -0.5657657146887259403 ) ) ;
#30353=EDGE_CURVE ( 'NONE', #6738, #8886, #22643, .T. ) ;
#30358=DIRECTION ( 'NONE',  ( 0.000000000000000000, 0.000000000000000000, -1.000000000000000000 ) ) ;
#30364=DIRECTION ( 'NONE',  ( 0.000000000000000000, -1.000000000000000000, 2.168404344971008128E-16 ) ) ;
#30372=EDGE_CURVE ( 'NONE', #9980, #24584, #28646, .T. ) ;
#30375=DIRECTION ( 'NONE',  ( 0.000000000000000000, -2.168404344971008868E-16, -1.000000000000000000 ) ) ;
#30378=CARTESIAN_POINT ( 'NONE',  ( 50.40000000000001990, -0.6304760106459033064, -3.950000000000022826 ) ) ;
#30380=CARTESIAN_POINT ( 'NONE',  ( -35.85663232820584057, 0.4576450603546802220, -5.200000000000000178 ) ) ;
#30388=VERTEX_POINT ( 'NONE', #16448 ) ;
#30390=CARTESIAN_POINT ( 'NONE',  ( -35.85663232820596846, 3.779372838781794641, -3.883777296072516094 ) ) ;
#30394=DIRECTION ( 'NONE',  ( -1.000000000000000000, -2.586136946169074517E-16, 0.000000000000000000 ) ) ;
#30397=DIRECTION ( 'NONE',  ( -1.000000000000000000, -0.000000000000000000, -0.000000000000000000 ) ) ;
#30399=ADVANCED_FACE ( 'NONE', ( #24044 ), #14547, .F. ) ;
#30407=FACE_OUTER_BOUND ( 'NONE', #22814, .T. ) ;
#30413=EDGE_LOOP ( 'NONE', ( #20632, #697, #25557, #12646 ) ) ;
#30422=VERTEX_POINT ( 'NONE', #21700 ) ;
#30438=CARTESIAN_POINT ( 'NONE',  ( 57.00057550097274373, 0.8023623105721646720, 2.473098203180232879 ) ) ;
#30439=CARTESIAN_POINT ( 'NONE',  ( 57.00000000000001421, 0.6999999999999999556, -2.452039967047845437 ) ) ;
#30445=DIRECTION ( 'NONE',  ( 0.000000000000000000, 1.000000000000000000, 0.000000000000000000 ) ) ;
#30448=DIRECTION ( 'NONE',  ( 0.000000000000000000, 0.000000000000000000, -1.000000000000000000 ) ) ;
#30450=VERTEX_POINT ( 'NONE', #14222 ) ;
#30452=ORIENTED_EDGE ( 'NONE', *, *, #26346, .T. ) ;
#30455=CARTESIAN_POINT ( 'NONE',  ( 51.80000000000001847, -3.726179070414207928, -1.100000000000000089 ) ) ;
#30456=ORIENTED_EDGE ( 'NONE', *, *, #24711, .F. ) ;
#30461=ORIENTED_EDGE ( 'NONE', *, *, #7127, .T. ) ;
#30464=CARTESIAN_POINT ( 'NONE',  ( 57.04415282905778639, -0.8156862745098041323, -2.468735688885368873 ) ) ;
#30469=CARTESIAN_POINT ( 'NONE',  ( 57.04534525700438508, 0.7498361808180106225, -1.778489416763646025 ) ) ;
#30476=EDGE_CURVE ( 'NONE', #26264, #3572, #9504, .T. ) ;
#30477=AXIS2_PLACEMENT_3D ( 'NONE', #10864, #19918, #25122 ) ;
#30487=LINE ( 'NONE', #13703, #6580 ) ;
#30488=ORIENTED_EDGE ( 'NONE', *, *, #19091, .T. ) ;
#30492=ORIENTED_EDGE ( 'NONE', *, *, #22977, .F. ) ;
#30494=DIRECTION ( 'NONE',  ( 0.000000000000000000, 1.000000000000000000, 0.000000000000000000 ) ) ;
#30495=DIRECTION ( 'NONE',  ( 0.000000000000000000, 1.000000000000000000, 0.000000000000000000 ) ) ;
#30497=CARTESIAN_POINT ( 'NONE',  ( -36.23324115033479131, 5.027926281937889819, -1.353187539901933967 ) ) ;
#30499=CARTESIAN_POINT ( 'NONE',  ( 56.99139336475067807, 0.7078862301243328270, 1.763423818528686349 ) ) ;
#30511=CARTESIAN_POINT ( 'NONE',  ( 58.45000000000001705, -0.7500000000000000000, 1.745709025009609228 ) ) ;
#30522=EDGE_LOOP ( 'NONE', ( #17973, #18771, #18927, #9003 ) ) ;
#30526=DIRECTION ( 'NONE',  ( 1.000000000000000000, -0.000000000000000000, -0.000000000000000000 ) ) ;
#30530=DIRECTION ( 'NONE',  ( 0.000000000000000000, 0.000000000000000000, -1.000000000000000000 ) ) ;
#30533=DIRECTION ( 'NONE',  ( 0.000000000000000000, -1.000000000000000000, -1.734723475976807094E-15 ) ) ;
#30534=CARTESIAN_POINT ( 'NONE',  ( -54.49999999999997868, 1.549598385535858380, -4.064203588144675194 ) ) ;
#30537=CARTESIAN_POINT ( 'NONE',  ( 57.02118883257515591, -0.7413508443325595998, 1.786034507790101866 ) ) ;
#30540=CARTESIAN_POINT ( 'NONE',  ( -35.98994760229851408, 3.426725948577779679, -3.937891352654224963 ) ) ;
#30542=VECTOR ( 'NONE', #1410, 1000.000000000000000 ) ;
#30546=DIRECTION ( 'NONE',  ( 1.000000000000000000, 0.000000000000000000, 0.000000000000000000 ) ) ;
#30555=CARTESIAN_POINT ( 'NONE',  ( 47.10000000000002274, -4.179189514726506793, -0.9000000000000000222 ) ) ;
#30558=CARTESIAN_POINT ( 'NONE',  ( 15.44631504820154433, -4.878538113278835020, 1.812957040858152569 ) ) ;
#30560=ORIENTED_EDGE ( 'NONE', *, *, #12073, .T. ) ;
#30572=TOROIDAL_SURFACE ( 'NONE', #17429, -24.59258869922086888, 30.00000000000000000 ) ;
#30580=CARTESIAN_POINT ( 'NONE',  ( 56.95000000000001705, -0.7227197132926967971, 2.497551541979256218 ) ) ;
#30582=DIRECTION ( 'NONE',  ( 1.000000000000000000, 5.172273892338149033E-16, 0.000000000000000000 ) ) ;
#30584=CARTESIAN_POINT ( 'NONE',  ( 57.04413099161754985, 0.7497394063391640273, 2.421432380119032501 ) ) ;
#30589=CARTESIAN_POINT ( 'NONE',  ( 15.39414421509789932, 5.035245099686891379, -1.330662535294792281 ) ) ;
#30601=SPHERICAL_SURFACE ( 'NONE', #2771, 0.05000000000000000278 ) ;
#30607=DIRECTION ( 'NONE',  ( 0.000000000000000000, 0.000000000000000000, -1.000000000000000000 ) ) ;
#30609=CIRCLE ( 'NONE', #19004, 4.000000000000022204 ) ;
#30614=AXIS2_PLACEMENT_3D ( 'NONE', #8634, #28432, #1989 ) ;
#30622=EDGE_CURVE ( 'NONE', #2736, #15656, #27201, .T. ) ;
#30624=CARTESIAN_POINT ( 'NONE',  ( 56.95606009725792518, -0.7486802684473473635, -2.489875068279050918 ) ) ;
#30625=CARTESIAN_POINT ( 'NONE',  ( 15.18463186935387021, 2.199885893005444348, 4.939696249117986326 ) ) ;
#30627=DIRECTION ( 'NONE',  ( 0.000000000000000000, 0.000000000000000000, -1.000000000000000000 ) ) ;
#30628=DIRECTION ( 'NONE',  ( 1.000000000000000000, 9.742518634745087578E-17, -4.338815227902166479E-17 ) ) ;
#30631=DIRECTION ( 'NONE',  ( -1.000000000000000000, 0.000000000000000000, 0.000000000000000000 ) ) ;
#30640=AXIS2_PLACEMENT_3D ( 'NONE', #689, #17956, #17653 ) ;
#30642=ORIENTED_EDGE ( 'NONE', *, *, #8113, .T. ) ;
#30646=ORIENTED_EDGE ( 'NONE', *, *, #3366, .F. ) ;
#30650=CARTESIAN_POINT ( 'NONE',  ( -35.85663232820579793, 4.018128179617487916, 3.618665901676695107 ) ) ;
#30651=ORIENTED_EDGE ( 'NONE', *, *, #686, .F. ) ;
#30652=VERTEX_POINT ( 'NONE', #8974 ) ;
#30653=FACE_OUTER_BOUND ( 'NONE', #10992, .T. ) ;
#30656=VERTEX_POINT ( 'NONE', #11336 ) ;
#30657=CARTESIAN_POINT ( 'NONE',  ( 47.00000000000002132, 1.391941090707534023, 3.750000000000022649 ) ) ;
#30665=TOROIDAL_SURFACE ( 'NONE', #15582, 4.000000000000022204, 0.1000000000000000056 ) ;
#30666=ADVANCED_FACE ( 'NONE', ( #15933, #1071 ), #8654, .T. ) ;
#30667=CARTESIAN_POINT ( 'NONE',  ( -54.47754877553799702, -1.508273929415538062, -3.305418158118663463 ) ) ;
#30669=DIRECTION ( 'NONE',  ( -4.670714851210922627E-16, -0.9333474217026305197, -0.3589743589743593088 ) ) ;
#30672=VECTOR ( 'NONE', #11360, 1000.000000000000000 ) ;
#30674=VECTOR ( 'NONE', #14815, 1000.000000000000000 ) ;
#30676=CARTESIAN_POINT ( 'NONE',  ( 15.03925126672132961, 3.426725943139509845, 3.937891353488782276 ) ) ;
#30680=EDGE_CURVE ( 'NONE', #26503, #16594, #16604, .T. ) ;
#30684=CARTESIAN_POINT ( 'NONE',  ( 47.00000000000002132, 2.478823385132571406E-14, 4.100000000000022737 ) ) ;
#30687=CARTESIAN_POINT ( 'NONE',  ( -36.11187263677869197, -0.3981319440505055596, 5.199999999410220397 ) ) ;
#30694=CARTESIAN_POINT ( 'NONE',  ( 48.46709009337374141, 1.365599538210783281, 3.854893000251051749 ) ) ;
#30697=VERTEX_POINT ( 'NONE', #18488 ) ;
#30699=CARTESIAN_POINT ( 'NONE',  ( 50.40000000000001990, -1.409787217987148233, 3.950000000000022826 ) ) ;
#30708=CARTESIAN_POINT ( 'NONE',  ( -36.92398358572908990, 2.945786441214503171, 4.543674732827777341 ) ) ;
#30711=DIRECTION ( 'NONE',  ( 0.000000000000000000, 1.000000000000000000, 1.224646799147353207E-16 ) ) ;
#30719=CARTESIAN_POINT ( 'NONE',  ( 57.04767748491563140, -0.7500000000000049960, 1.778341924377874639 ) ) ;
#30720=CIRCLE ( 'NONE', #5931, 0.04999999999999991257 ) ;
#30721=CARTESIAN_POINT ( 'NONE',  ( -35.98952425903317476, 2.686240675664352207, -4.475885398016837158 ) ) ;
#30723=DIRECTION ( 'NONE',  ( 0.000000000000000000, 0.000000000000000000, -1.000000000000000000 ) ) ;
#30724=CARTESIAN_POINT ( 'NONE',  ( 15.59140265158955962, 0.9780988077348221621, -5.318542208600380405 ) ) ;
#30726=VECTOR ( 'NONE', #21333, 1000.000000000000000 ) ;
#30728=DIRECTION ( 'NONE',  ( 0.000000000000000000, 1.000000000000000000, 0.000000000000000000 ) ) ;
#30731=DIRECTION ( 'NONE',  ( 0.000000000000000000, 1.000000000000000000, -1.224646799147353207E-16 ) ) ;
#30736=CARTESIAN_POINT ( 'NONE',  ( -36.11122220296842045, 5.068511731019554212, 1.228278365481957790 ) ) ;
#30741=CARTESIAN_POINT ( 'NONE',  ( -36.31440869660541892, -4.962395293451386635, 1.554871187131941834 ) ) ;
#30742=CARTESIAN_POINT ( 'NONE',  ( 50.31550977796904789, -1.386241252175274496, 3.851058308531627894 ) ) ;
#30744=AXIS2_PLACEMENT_3D ( 'NONE', #18820, #26081, #31146 ) ;
#30745=ORIENTED_EDGE ( 'NONE', *, *, #6499, .T. ) ;
#30746=ADVANCED_FACE ( 'NONE', ( #3602 ), #23083, .F. ) ;
#30747=DIRECTION ( 'NONE',  ( 0.000000000000000000, 0.000000000000000000, -1.000000000000000000 ) ) ;
#30750=ORIENTED_EDGE ( 'NONE', *, *, #83, .T. ) ;
#30754=ORIENTED_EDGE ( 'NONE', *, *, #9670, .F. ) ;
#30764=DIRECTION ( 'NONE',  ( 1.000000000000000000, -0.000000000000000000, -0.000000000000000000 ) ) ;
#30765=CARTESIAN_POINT ( 'NONE',  ( 15.45522337368516297, 5.005099703116323795, -1.423440526321878563 ) ) ;
#30766=CARTESIAN_POINT ( 'NONE',  ( 57.03828022491683924, 0.8151581666669124315, 2.468910358759941914 ) ) ;
#30769=CARTESIAN_POINT ( 'NONE',  ( 50.40000000000003411, 0.7619326981554777056, -3.939508824314740032 ) ) ;
#30772=CARTESIAN_POINT ( 'NONE',  ( 50.32795105345940812, -1.409900792624644739, 3.850000304694922271 ) ) ;
#30773=ADVANCED_FACE ( 'NONE', ( #21020 ), #3743, .T. ) ;
#30774=LINE ( 'NONE', #9083, #2855 ) ;
#30777=ADVANCED_FACE ( 'NONE', ( #13239 ), #8408, .T. ) ;
#30778=DIRECTION ( 'NONE',  ( -0.000000000000000000, -1.000000000000000000, 0.000000000000000000 ) ) ;
#30788=CARTESIAN_POINT ( 'NONE',  ( 47.10000000000002274, -4.276948333784438283, -0.9210526315789475671 ) ) ;
#30791=ORIENTED_EDGE ( 'NONE', *, *, #13867, .F. ) ;
#30799=CARTESIAN_POINT ( 'NONE',  ( 16.00221665700883023, 3.629052419422171827, 4.014440194077253388 ) ) ;
#30802=DIRECTION ( 'NONE',  ( 0.000000000000000000, -1.000000000000000000, 0.000000000000000000 ) ) ;
#30809=DIRECTION ( 'NONE',  ( 0.000000000000000000, 1.000000000000000000, -1.224646799147353207E-16 ) ) ;
#30812=EDGE_CURVE ( 'NONE', #18266, #18396, #31248, .T. ) ;
#30813=LINE ( 'NONE', #14013, #29501 ) ;
#30822=EDGE_LOOP ( 'NONE', ( #10175, #17005, #27732, #4767 ) ) ;
#30823=FACE_OUTER_BOUND ( 'NONE', #10686, .T. ) ;
#30826=CARTESIAN_POINT ( 'NONE',  ( 50.40000000000001279, 0.6304760106459513791, 3.950000000000022826 ) ) ;
#30830=CYLINDRICAL_SURFACE ( 'NONE', #27511, 5.407411300779133789 ) ;
#30833=CARTESIAN_POINT ( 'NONE',  ( -54.47366401599046526, -1.505709097230404359, -3.303769268891089350 ) ) ;
#30835=CARTESIAN_POINT ( 'NONE',  ( 57.00000000000001421, 0.7256347085964565125, 1.800308733460772359 ) ) ;
#30837=CARTESIAN_POINT ( 'NONE',  ( 51.87908472284573946, 0.03364117306051616491, 4.372691834281944523 ) ) ;
#30843=LINE ( 'NONE', #9160, #3830 ) ;
#30847=CARTESIAN_POINT ( 'NONE',  ( -36.48174642952978530, 0.4008586329627822908, 5.396496690166785903 ) ) ;
#30855=DIRECTION ( 'NONE',  ( -0.000000000000000000, -0.2573099415204678775, -0.9663289263986325484 ) ) ;
#30859=CARTESIAN_POINT ( 'NONE',  ( 56.95000000000001705, 0.7137254901960785602, 2.500119182087999548 ) ) ;
#30860=CIRCLE ( 'NONE', #4048, 1.000000000000000444 ) ;
#30862=CARTESIAN_POINT ( 'NONE',  ( -35.85663232820584767, -3.817150320979536104, -2.203324261493425862 ) ) ;
#30874=CARTESIAN_POINT ( 'NONE',  ( -36.50489844130355976, 2.884962146574165054, -4.577321775072915599 ) ) ;
#30875=CARTESIAN_POINT ( 'NONE',  ( 48.42277498379875311, 1.384253668070434484, -3.859284659399053741 ) ) ;
#30878=EDGE_CURVE ( 'NONE', #16179, #5897, #2941, .T. ) ;
#30879=CIRCLE ( 'NONE', #15210, 1.000000000000000000 ) ;
#30886=VERTEX_POINT ( 'NONE', #26850 ) ;
#30892=CARTESIAN_POINT ( 'NONE',  ( 15.29954477411457070, -2.199885872770988904, -4.939696258129290030 ) ) ;
#30893=CARTESIAN_POINT ( 'NONE',  ( -35.85663232820592583, 4.804073783693418420, 2.042134687550397398 ) ) ;
#30894=CARTESIAN_POINT ( 'NONE',  ( 15.67083574136753121, -5.009497273852900889, 2.047744636826879461 ) ) ;
#30898=CARTESIAN_POINT ( 'NONE',  ( -36.26369610968610857, -5.012449653004694028, 1.400819699606154822 ) ) ;
#30899=CARTESIAN_POINT ( 'NONE',  ( 50.30837315852409830, -1.391941090707504047, 3.850000000000021849 ) ) ;
#30902=AXIS2_PLACEMENT_3D ( 'NONE', #26882, #13651, #30923 ) ;
#30903=ORIENTED_EDGE ( 'NONE', *, *, #24377, .T. ) ;
#30908=ORIENTED_EDGE ( 'NONE', *, *, #27445, .T. ) ;
#30910=ORIENTED_EDGE ( 'NONE', *, *, #1489, .T. ) ;
#30921=FACE_OUTER_BOUND ( 'NONE', #20586, .T. ) ;
#30922=CARTESIAN_POINT ( 'NONE',  ( -36.79682133506354802, -3.614202567155977874, -4.024415706308069218 ) ) ;
#30923=DIRECTION ( 'NONE',  ( 0.000000000000000000, 0.000000000000000000, -1.000000000000000000 ) ) ;
#30927=VERTEX_POINT ( 'NONE', #4503 ) ;
#30932=AXIS2_PLACEMENT_3D ( 'NONE', #13949, #4150, #1942 ) ;
#30934=CARTESIAN_POINT ( 'NONE',  ( 47.00000000000002842, -4.179189514726506793, -1.000000000000000000 ) ) ;
#30938=ORIENTED_EDGE ( 'NONE', *, *, #2261, .T. ) ;
#30939=CARTESIAN_POINT ( 'NONE',  ( 15.49702763512083337, 4.962395293451323575, 1.554871187131933841 ) ) ;
#30946=PLANE ( 'NONE',  #23292 ) ;
#30953=EDGE_LOOP ( 'NONE', ( #15086, #14213, #4815, #21886 ) ) ;
#30955=EDGE_CURVE ( 'NONE', #17756, #12911, #8006, .T. ) ;
#30956=DIRECTION ( 'NONE',  ( -1.000000000000000000, 0.000000000000000000, 0.000000000000000000 ) ) ;
#30961=CARTESIAN_POINT ( 'NONE',  ( -36.22818246778668083, -2.595266697484658103, 4.757426534476427271 ) ) ;
#30966=CARTESIAN_POINT ( 'NONE',  ( 51.89143965165623484, 1.032956679176618869E-15, -4.375000000000000888 ) ) ;
#30972=CARTESIAN_POINT ( 'NONE',  ( 15.03925126672133139, -4.683225679163343536, 2.703237727951232294 ) ) ;
#30975=DIRECTION ( 'NONE',  ( 0.000000000000000000, 0.3589743589743574215, 0.9333474217026310749 ) ) ;
#30978=CARTESIAN_POINT ( 'NONE',  ( 50.40741710815419196, 1.342093792059667390, 3.874237195466570416 ) ) ;
#30984=FACE_OUTER_BOUND ( 'NONE', #14218, .T. ) ;
#30995=PLANE ( 'NONE',  #1813 ) ;
#30996=CARTESIAN_POINT ( 'NONE',  ( -36.26369610968609436, -0.2166734227622266473, 5.199999998324988049 ) ) ;
#30997=CARTESIAN_POINT ( 'NONE',  ( 33.47623932017462778, -4.683225679163339983, 2.703237727951233182 ) ) ;
#30999=EDGE_CURVE ( 'NONE', #13545, #24391, #6488, .T. ) ;
#31000=CARTESIAN_POINT ( 'NONE',  ( -36.52757395963739384, -4.797343084509235744, 2.497389432263963371 ) ) ;
#31005=DIRECTION ( 'NONE',  ( 0.000000000000000000, 0.000000000000000000, 1.000000000000000000 ) ) ;
#31011=CONICAL_SURFACE ( 'NONE', #17358, 5.407411300779140895, 0.1317529408396977408 ) ;
#31015=CARTESIAN_POINT ( 'NONE',  ( 48.50000000000002132, 1.426739617975221641, 3.843750000000023093 ) ) ;
#31020=EDGE_CURVE ( 'NONE', #4137, #19631, #910, .T. ) ;
#31021=CARTESIAN_POINT ( 'NONE',  ( 57.01637874260923411, -0.7374533274050908416, 1.789443367489095049 ) ) ;
#31025=CARTESIAN_POINT ( 'NONE',  ( 57.00000000000001421, 0.6999999999999999556, -1.745709025009609228 ) ) ;
#31027=FACE_OUTER_BOUND ( 'NONE', #4794, .T. ) ;
#31032=CARTESIAN_POINT ( 'NONE',  ( 50.36033030378881392, -1.282137971188096914, -3.869545987293864453 ) ) ;
#31038=CARTESIAN_POINT ( 'NONE',  ( -35.85663232820582635, 5.086913985776129188, 1.171642053949150553 ) ) ;
#31041=EDGE_LOOP ( 'NONE', ( #1035, #21393, #27973, #20241 ) ) ;
#31042=CARTESIAN_POINT ( 'NONE',  ( -45.15971931043468146, -8.341470767433328331E-15, 0.000000000000000000 ) ) ;
#31043=VERTEX_POINT ( 'NONE', #16863 ) ;
#31044=CARTESIAN_POINT ( 'NONE',  ( 57.05000000000001847, -0.7794871794871794934, -1.732743413496389717 ) ) ;
#31046=VERTEX_POINT ( 'NONE', #30788 ) ;
#31049=FILL_AREA_STYLE_COLOUR ( '', #8065 ) ;
#31051=EDGE_LOOP ( 'NONE', ( #7376, #14735, #16402, #5255 ) ) ;
#31061=EDGE_CURVE ( 'NONE', #4056, #9481, #23685, .T. ) ;
#31062=AXIS2_PLACEMENT_3D ( 'NONE', #27013, #4011, #8741 ) ;
#31066=DIRECTION ( 'NONE',  ( -1.000000000000000000, -0.000000000000000000, -0.000000000000000000 ) ) ;
#31069=FACE_OUTER_BOUND ( 'NONE', #5750, .T. ) ;
#31073=CARTESIAN_POINT ( 'NONE',  ( 51.80000000000001847, -0.2842225609755594795, -1.577752156565102655E-15 ) ) ;
#31084=EDGE_LOOP ( 'NONE', ( #5618, #23238, #22965 ) ) ;
#31085=CARTESIAN_POINT ( 'NONE',  ( 15.03925126672127632, 4.804073783693426414, 2.042134687550409389 ) ) ;
#31086=VERTEX_POINT ( 'NONE', #26500 ) ;
#31087=DIRECTION ( 'NONE',  ( 0.000000000000000000, 1.000000000000000000, -0.000000000000000000 ) ) ;
#31091=DIRECTION ( 'NONE',  ( 1.000000000000000000, -7.137062321707291160E-17, 7.924918191882970879E-17 ) ) ;
#31094=VERTEX_POINT ( 'NONE', #6567 ) ;
#31096=ADVANCED_FACE ( 'NONE', ( #4805 ), #13985, .T. ) ;
#31098=EDGE_CURVE ( 'NONE', #28219, #27463, #12080, .T. ) ;
#31102=EDGE_LOOP ( 'NONE', ( #20560, #10948, #18138, #12611 ) ) ;
#31103=CARTESIAN_POINT ( 'NONE',  ( 58.45000000000001705, -0.8156862745098041323, 2.468735688885368873 ) ) ;
#31106=AXIS2_PLACEMENT_3D ( 'NONE', #5667, #23677, #24965 ) ;
#31107=DIRECTION ( 'NONE',  ( -1.000000000000000000, 0.000000000000000000, 0.000000000000000000 ) ) ;
#31112=FACE_OUTER_BOUND ( 'NONE', #16334, .T. ) ;
#31114=AXIS2_PLACEMENT_3D ( 'NONE', #27254, #10476, #22974 ) ;
#31115=CIRCLE ( 'NONE', #9385, 0.09999999999999982514 ) ;
#31119=CARTESIAN_POINT ( 'NONE',  ( 15.03925126672132961, -3.056483311920829671, -4.206888370749746642 ) ) ;
#31122=CARTESIAN_POINT ( 'NONE',  ( -36.92362342067257686, 3.309998894527826696, 4.278958290368546358 ) ) ;
#31123=ORIENTED_EDGE ( 'NONE', *, *, #5838, .F. ) ;
#31135=EDGE_CURVE ( 'NONE', #3198, #30886, #10558, .T. ) ;
#31140=DIRECTION ( 'NONE',  ( -1.000000000000000000, 0.000000000000000000, 8.673617379883787770E-15 ) ) ;
#31143=VECTOR ( 'NONE', #8523, 1000.000000000000000 ) ;
#31146=DIRECTION ( 'NONE',  ( 0.000000000000000000, -0.3137254901960787046, -0.9495137264943726008 ) ) ;
#31148=CIRCLE ( 'NONE', #3839, 0.09999999999999982514 ) ;
#31149=DIRECTION ( 'NONE',  ( 0.000000000000000000, 0.000000000000000000, -1.000000000000000000 ) ) ;
#31151=CARTESIAN_POINT ( 'NONE',  ( -36.00197790576392265, -1.123735532908290979, 5.289358697221548056 ) ) ;
#31153=CARTESIAN_POINT ( 'NONE',  ( 56.95000000000001705, -0.7137254901960795594, -2.500119182087999103 ) ) ;
#31156=ORIENTED_EDGE ( 'NONE', *, *, #10494, .F. ) ;
#31158=FACE_OUTER_BOUND ( 'NONE', #29158, .T. ) ;
#31159=EDGE_LOOP ( 'NONE', ( #16908, #13343, #23337, #11158 ) ) ;
#31160=CARTESIAN_POINT ( 'NONE',  ( 15.41080140630239192, 0.6967302926296516929, -5.374298406429034891 ) ) ;
#31165=CIRCLE ( 'NONE', #12938, 0.05000000000000012768 ) ;
#31170=VECTOR ( 'NONE', #21602, 1000.000000000000000 ) ;
#31173=EDGE_CURVE ( 'NONE', #9785, #19277, #14586, .T. ) ;
#31180=VECTOR ( 'NONE', #722, 1000.000000000000000 ) ;
#31183=DIRECTION ( 'NONE',  ( 1.000000000000000000, 0.000000000000000000, 0.000000000000000000 ) ) ;
#31186=ORIENTED_EDGE ( 'NONE', *, *, #29531, .F. ) ;
#31188=CARTESIAN_POINT ( 'NONE',  ( -44.49999999999997868, -1.499999999999999556, -4.029888335921975262 ) ) ;
#31190=CARTESIAN_POINT ( 'NONE',  ( -35.85663232820584057, -5.086913985776159386, 1.171642053949095930 ) ) ;
#31194=CARTESIAN_POINT ( 'NONE',  ( 15.18459684427940104, -1.123735532908282320, -5.289358697221548056 ) ) ;
#31197=FACE_OUTER_BOUND ( 'NONE', #3528, .T. ) ;
#31198=VECTOR ( 'NONE', #650, 1000.000000000000000 ) ;
#31199=CARTESIAN_POINT ( 'NONE',  ( -54.49999999999997868, -1.549999999999999600, -4.029888335921975262 ) ) ;
#31208=DIRECTION ( 'NONE',  ( 0.000000000000000000, 0.000000000000000000, -1.000000000000000000 ) ) ;
#31210=CARTESIAN_POINT ( 'NONE',  ( 16.10705563471231017, -5.094475812726788178, 1.819860688632810142 ) ) ;
#31212=ORIENTED_EDGE ( 'NONE', *, *, #27756, .F. ) ;
#31216=DIRECTION ( 'NONE',  ( 1.000000000000000000, 0.000000000000000000, 0.000000000000000000 ) ) ;
#31218=CYLINDRICAL_SURFACE ( 'NONE', #14396, 0.04999999999999991257 ) ;
#31226=ORIENTED_EDGE ( 'NONE', *, *, #1304, .F. ) ;
#31229=ADVANCED_FACE ( 'NONE', ( #7346 ), #3965, .T. ) ;
#31232=CARTESIAN_POINT ( 'NONE',  ( 56.95118308248727601, -0.7317690799413573144, 2.494914055551520793 ) ) ;
#31233=DIRECTION ( 'NONE',  ( 0.000000000000000000, 0.000000000000000000, -1.000000000000000000 ) ) ;
#31234=CARTESIAN_POINT ( 'NONE',  ( -54.49999999999997868, -1.549582583372308253, 3.331868970650947226 ) ) ;
#31241=DIRECTION ( 'NONE',  ( 0.000000000000000000, 0.000000000000000000, 1.000000000000000000 ) ) ;
#31242=CARTESIAN_POINT ( 'NONE',  ( -36.40793637698147478, -2.334444681449701520, -4.877899991435287852 ) ) ;
#31245=CARTESIAN_POINT ( 'NONE',  ( 15.03925126672132961, -1.793057972834796399, 4.026191436120392986 ) ) ;
#31248=B_SPLINE_CURVE_WITH_KNOTS ( 'NONE', 3,
 ( #7231, #26068, #28919, #14190, #28450, #4845, #2486, #19130, #18807, #18961, #4688, #7082, #108, #14343, #12141, #23865 ),
 .UNSPECIFIED., .F., .F.,
 ( 4, 2, 2, 2, 2, 2, 2, 4 ),
 ( 0.000000000000000000, 0.0004351083927046389037, 0.0008702167854092778074, 0.001740433570818555615, 0.002175541963523193977, 0.002610650356227832338, 0.003045758748932470700, 0.003480867141637109495 ),
 .UNSPECIFIED. ) ;
#31249=CARTESIAN_POINT ( 'NONE',  ( 48.30000000000002558, -0.6462379109120512943, 4.048750000000022276 ) ) ;
#31254=ORIENTED_EDGE ( 'NONE', *, *, #29808, .T. ) ;
#31258=CARTESIAN_POINT ( 'NONE',  ( 15.94709373951304343, 4.924630501335168553, 2.234249019593653074 ) ) ;
#31259=EDGE_LOOP ( 'NONE', ( #10090, #19700, #30142, #23415 ) ) ;
#31262=ORIENTED_EDGE ( 'NONE', *, *, #24412, .F. ) ;
#31267=EDGE_CURVE ( 'NONE', #21494, #30274, #10811, .T. ) ;
#31275=ADVANCED_FACE ( 'NONE', ( #1456 ), #28759, .F. ) ;
#31288=DIRECTION ( 'NONE',  ( 1.000000000000000000, -0.000000000000000000, -0.000000000000000000 ) ) ;
#31306=EDGE_CURVE ( 'NONE', #26152, #14356, #2958, .T. ) ;
#31315=CARTESIAN_POINT ( 'NONE',  ( -54.49998548284560940, 1.548795215916124457, 4.063650232134933482 ) ) ;
#31319=LINE ( 'NONE', #29400, #7660 ) ;
#31322=EDGE_CURVE ( 'NONE', #24297, #16545, #14075, .T. ) ;
#31326=CARTESIAN_POINT ( 'NONE',  ( 48.30000000000001847, 2.428612866367529932E-14, 4.000000000000022204 ) ) ;
ENDSEC;
END-ISO-10303-21;
